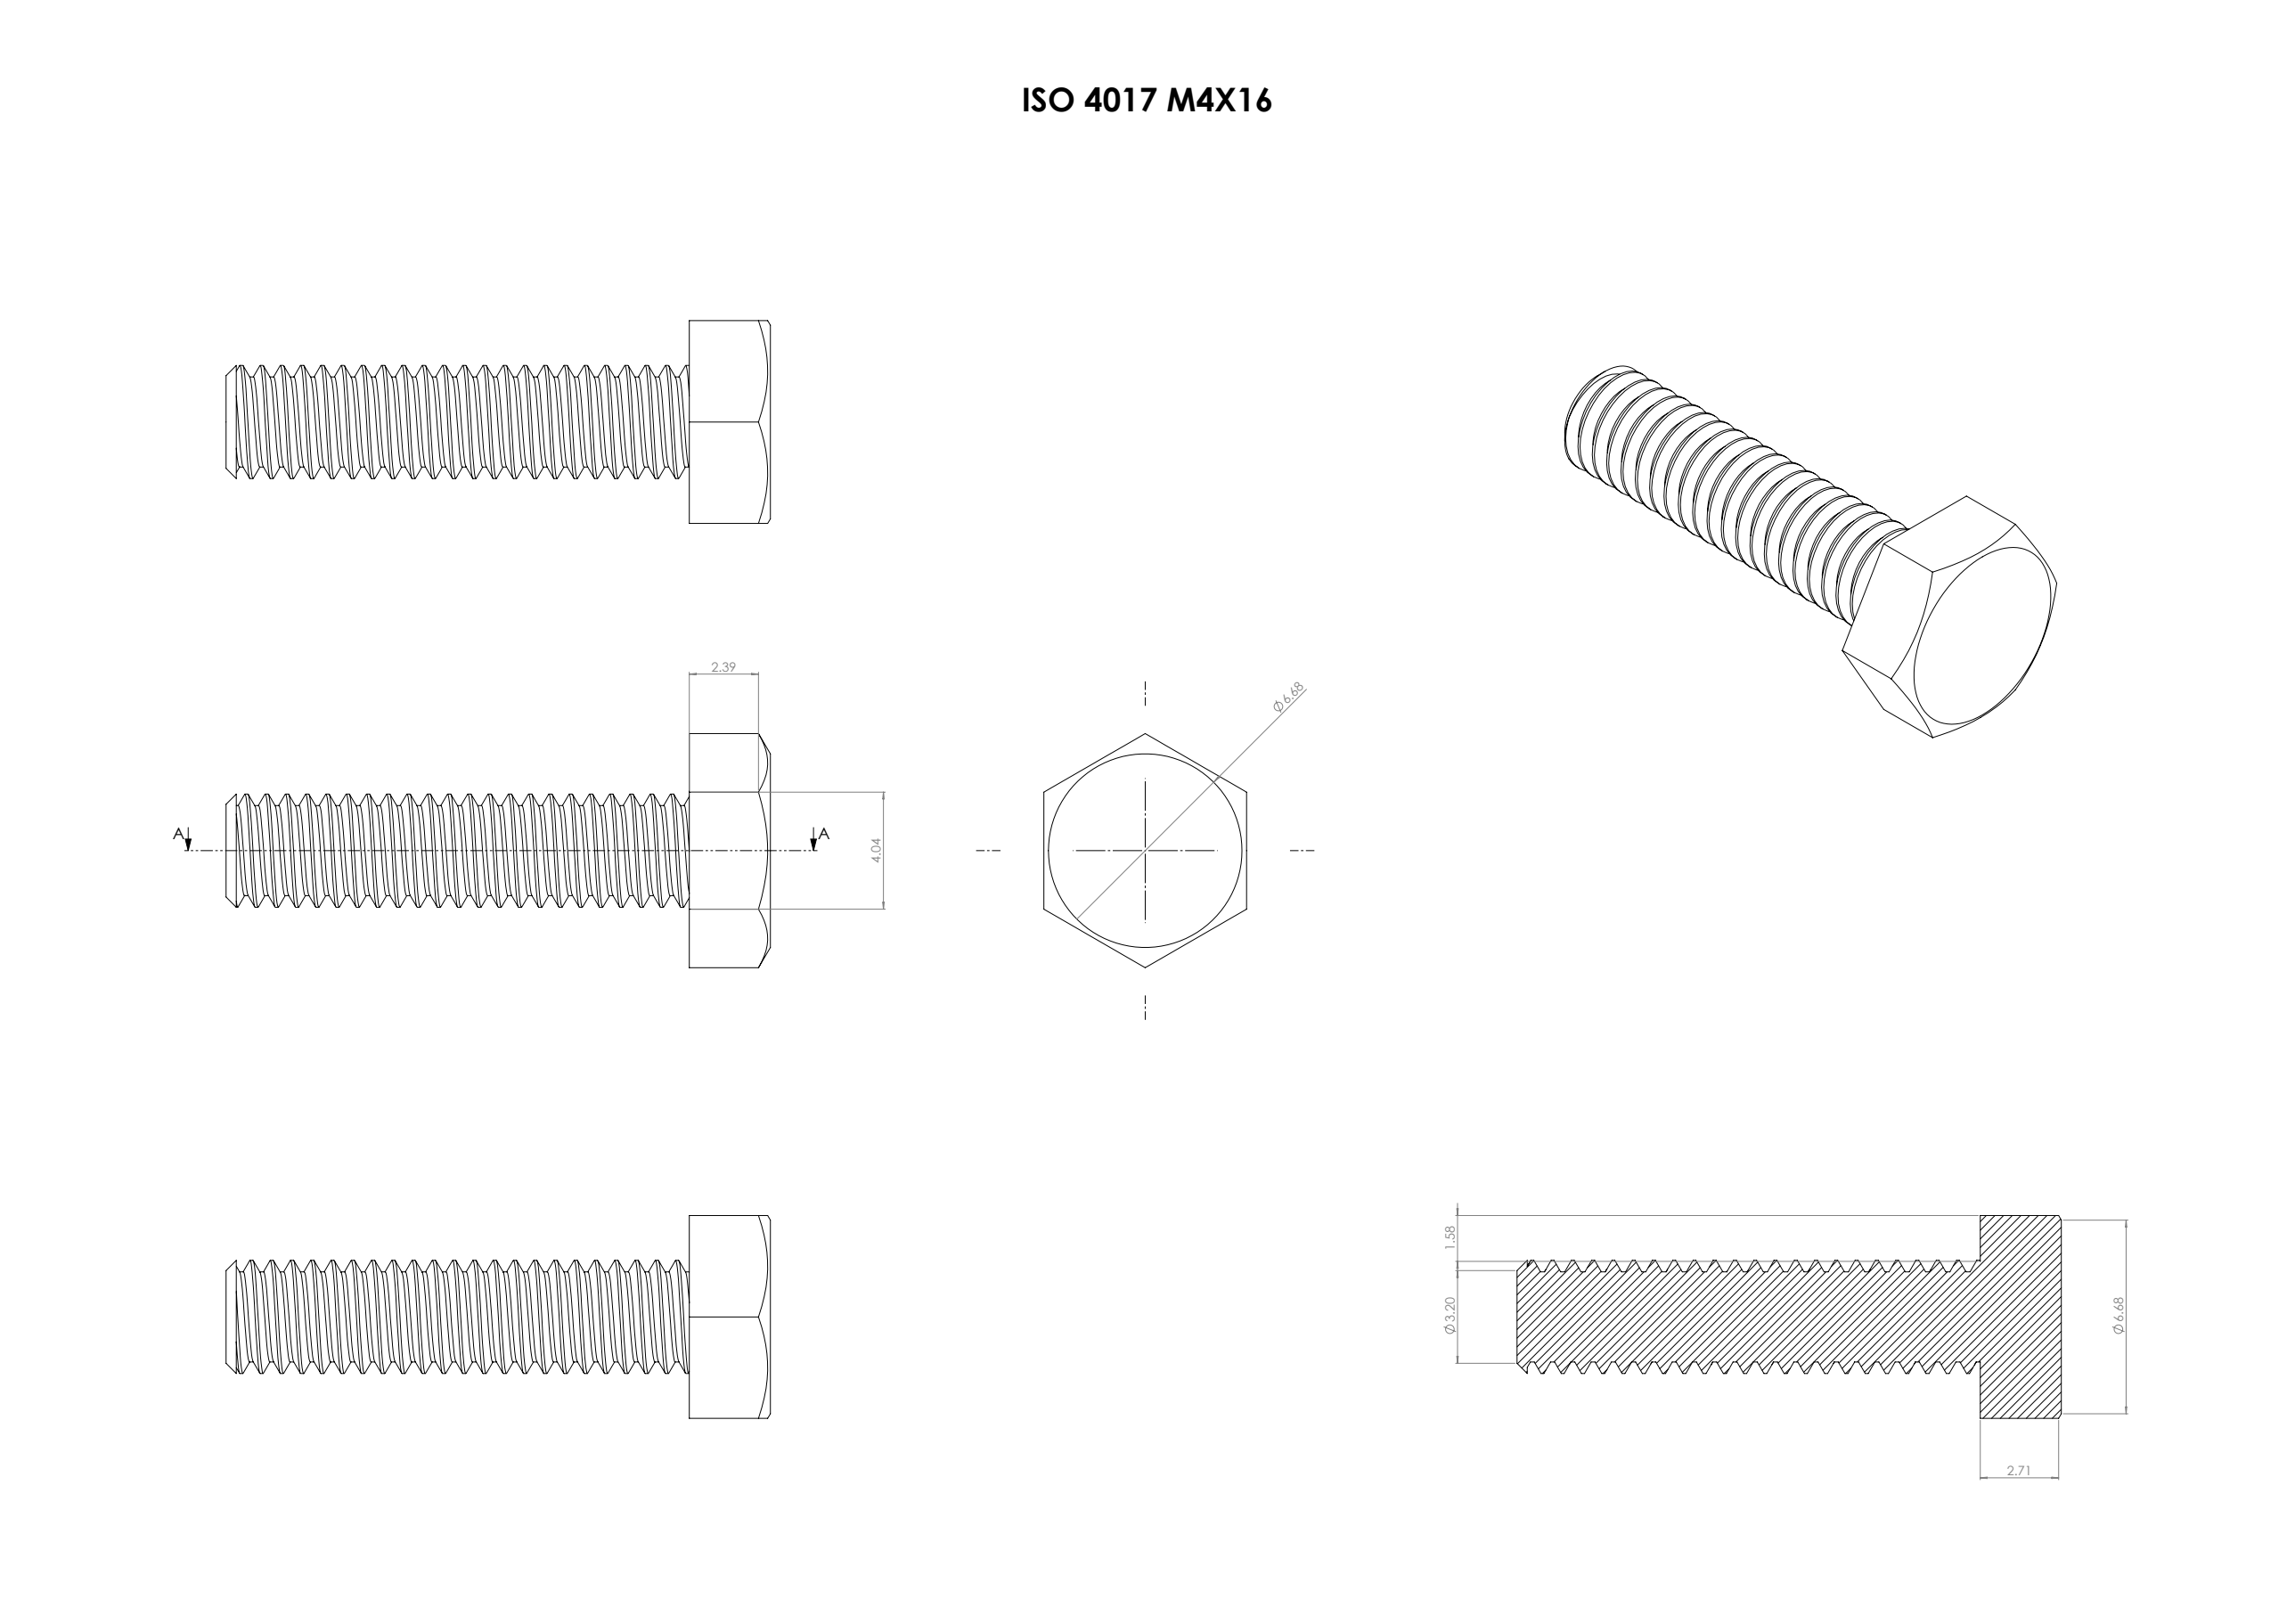
ISO-10303-21;
HEADER;
/* Generated by software containing ST-Developer
 * from STEP Tools, Inc. (www.steptools.com) 
 */

FILE_DESCRIPTION(
/* description */ (''),
/* implementation_level */ '2;1');

FILE_NAME(
/* name */ '09_ISO_4017_M4x16.step',
/* time_stamp */ '2026-10-21T02:01:14-07:00',
/* author */ (''),
/* organization */ (''),
/* preprocessor_version */ 'ST-DEVELOPER v20.2',
/* originating_system */ 'Autodesk Translation Framework v15.15.0.0',
/* authorisation */ '');

FILE_SCHEMA (('AUTOMOTIVE_DESIGN { 1 0 10303 214 3 1 1 }'));
ENDSEC;

DATA;
#10=MECHANICAL_DESIGN_GEOMETRIC_PRESENTATION_REPRESENTATION('',(#622),#37181);
#114=B_SPLINE_SURFACE_WITH_KNOTS('',3,3,((#28629,#28630,#28631,#28632,#28633,
#28634,#28635,#28636,#28637,#28638,#28639,#28640,#28641,#28642,#28643,#28644,
#28645,#28646,#28647,#28648,#28649,#28650,#28651,#28652,#28653,#28654,#28655,
#28656,#28657,#28658,#28659,#28660,#28661,#28662,#28663,#28664,#28665,#28666,
#28667,#28668,#28669,#28670,#28671,#28672,#28673,#28674,#28675,#28676,#28677,
#28678,#28679,#28680,#28681,#28682,#28683,#28684,#28685,#28686,#28687,#28688,
#28689,#28690,#28691,#28692,#28693,#28694,#28695,#28696,#28697,#28698,#28699,
#28700,#28701,#28702,#28703,#28704,#28705,#28706,#28707,#28708,#28709,#28710,
#28711,#28712,#28713,#28714,#28715,#28716,#28717,#28718,#28719,#28720,#28721,
#28722,#28723,#28724,#28725,#28726,#28727,#28728,#28729,#28730,#28731,#28732,
#28733,#28734,#28735,#28736,#28737,#28738,#28739,#28740,#28741,#28742,#28743,
#28744,#28745,#28746,#28747,#28748,#28749,#28750,#28751,#28752,#28753,#28754,
#28755,#28756,#28757,#28758,#28759,#28760,#28761,#28762,#28763,#28764,#28765,
#28766,#28767,#28768,#28769,#28770,#28771,#28772,#28773,#28774),(#28775,
#28776,#28777,#28778,#28779,#28780,#28781,#28782,#28783,#28784,#28785,#28786,
#28787,#28788,#28789,#28790,#28791,#28792,#28793,#28794,#28795,#28796,#28797,
#28798,#28799,#28800,#28801,#28802,#28803,#28804,#28805,#28806,#28807,#28808,
#28809,#28810,#28811,#28812,#28813,#28814,#28815,#28816,#28817,#28818,#28819,
#28820,#28821,#28822,#28823,#28824,#28825,#28826,#28827,#28828,#28829,#28830,
#28831,#28832,#28833,#28834,#28835,#28836,#28837,#28838,#28839,#28840,#28841,
#28842,#28843,#28844,#28845,#28846,#28847,#28848,#28849,#28850,#28851,#28852,
#28853,#28854,#28855,#28856,#28857,#28858,#28859,#28860,#28861,#28862,#28863,
#28864,#28865,#28866,#28867,#28868,#28869,#28870,#28871,#28872,#28873,#28874,
#28875,#28876,#28877,#28878,#28879,#28880,#28881,#28882,#28883,#28884,#28885,
#28886,#28887,#28888,#28889,#28890,#28891,#28892,#28893,#28894,#28895,#28896,
#28897,#28898,#28899,#28900,#28901,#28902,#28903,#28904,#28905,#28906,#28907,
#28908,#28909,#28910,#28911,#28912,#28913,#28914,#28915,#28916,#28917,#28918,
#28919,#28920),(#28921,#28922,#28923,#28924,#28925,#28926,#28927,#28928,
#28929,#28930,#28931,#28932,#28933,#28934,#28935,#28936,#28937,#28938,#28939,
#28940,#28941,#28942,#28943,#28944,#28945,#28946,#28947,#28948,#28949,#28950,
#28951,#28952,#28953,#28954,#28955,#28956,#28957,#28958,#28959,#28960,#28961,
#28962,#28963,#28964,#28965,#28966,#28967,#28968,#28969,#28970,#28971,#28972,
#28973,#28974,#28975,#28976,#28977,#28978,#28979,#28980,#28981,#28982,#28983,
#28984,#28985,#28986,#28987,#28988,#28989,#28990,#28991,#28992,#28993,#28994,
#28995,#28996,#28997,#28998,#28999,#29000,#29001,#29002,#29003,#29004,#29005,
#29006,#29007,#29008,#29009,#29010,#29011,#29012,#29013,#29014,#29015,#29016,
#29017,#29018,#29019,#29020,#29021,#29022,#29023,#29024,#29025,#29026,#29027,
#29028,#29029,#29030,#29031,#29032,#29033,#29034,#29035,#29036,#29037,#29038,
#29039,#29040,#29041,#29042,#29043,#29044,#29045,#29046,#29047,#29048,#29049,
#29050,#29051,#29052,#29053,#29054,#29055,#29056,#29057,#29058,#29059,#29060,
#29061,#29062,#29063,#29064,#29065,#29066),(#29067,#29068,#29069,#29070,
#29071,#29072,#29073,#29074,#29075,#29076,#29077,#29078,#29079,#29080,#29081,
#29082,#29083,#29084,#29085,#29086,#29087,#29088,#29089,#29090,#29091,#29092,
#29093,#29094,#29095,#29096,#29097,#29098,#29099,#29100,#29101,#29102,#29103,
#29104,#29105,#29106,#29107,#29108,#29109,#29110,#29111,#29112,#29113,#29114,
#29115,#29116,#29117,#29118,#29119,#29120,#29121,#29122,#29123,#29124,#29125,
#29126,#29127,#29128,#29129,#29130,#29131,#29132,#29133,#29134,#29135,#29136,
#29137,#29138,#29139,#29140,#29141,#29142,#29143,#29144,#29145,#29146,#29147,
#29148,#29149,#29150,#29151,#29152,#29153,#29154,#29155,#29156,#29157,#29158,
#29159,#29160,#29161,#29162,#29163,#29164,#29165,#29166,#29167,#29168,#29169,
#29170,#29171,#29172,#29173,#29174,#29175,#29176,#29177,#29178,#29179,#29180,
#29181,#29182,#29183,#29184,#29185,#29186,#29187,#29188,#29189,#29190,#29191,
#29192,#29193,#29194,#29195,#29196,#29197,#29198,#29199,#29200,#29201,#29202,
#29203,#29204,#29205,#29206,#29207,#29208,#29209,#29210,#29211,#29212)),
 .UNSPECIFIED.,.F.,.F.,.F.,(4,4),(4,1,1,1,1,1,1,1,1,1,1,1,1,1,1,1,1,1,1,
1,1,1,1,1,1,1,1,1,1,1,1,1,1,1,1,1,1,1,1,1,1,1,1,1,1,1,1,1,1,1,1,1,1,1,1,
1,1,1,1,1,1,1,1,1,1,1,1,1,1,1,1,1,1,1,1,1,1,1,1,1,1,1,1,1,1,1,1,1,1,1,1,
1,1,1,1,1,1,1,1,1,1,1,1,1,1,1,1,1,1,1,1,1,1,1,1,1,1,1,1,1,1,1,1,1,1,1,1,
1,1,1,1,1,1,1,1,1,1,1,1,1,1,1,1,4),(0.,0.0460148164544131),(8.31058692273977,
9.30711355020657,10.3036401776734,11.3001668051402,12.296693432607,13.2932200600738,
14.2897466875406,15.2862733150074,16.2827999424742,17.279326569941,18.2758531974078,
19.2723798248745,20.2689064523413,21.2654330798081,22.2619597072749,23.2584863347417,
24.2550129622085,25.2515395896753,26.2480662171421,27.2445928446089,28.2411194720757,
29.2376460995425,30.2341727270093,31.2306993544761,32.2272259819429,33.2237526094097,
34.2202792368765,35.2168058643433,36.2133324918101,37.2098591192769,38.2063857467437,
39.2029123742105,40.1994390016773,41.1959656291441,42.1924922566109,43.1890188840777,
44.1855455115445,45.1820721390113,46.1785987664781,47.1751253939449,48.1716520214117,
49.1681786488785,50.1647052763453,51.1612319038121,52.1577585312789,53.1542851587457,
54.1508117862125,55.1473384136793,56.1438650411461,57.1403916686129,58.1369182960797,
59.1334449235465,60.1299715510133,61.1264981784801,62.1230248059469,63.1195514334137,
64.1160780608805,65.1126046883473,66.1091313158141,67.1056579432809,68.1021845707477,
69.0987111982145,70.0952378256813,71.0917644531481,72.0882910806149,73.0848177080817,
74.0813443355485,75.0778709630153,76.0743975904821,77.0709242179488,78.0674508454156,
79.0639774728824,80.0605041003492,81.057030727816,82.0535573552828,83.0500839827496,
84.0466106102164,85.0431372376832,86.03966386515,87.0361904926168,88.0327171200836,
89.0292437475504,90.0257703750172,91.022297002484,92.0188236299508,93.0153502574176,
94.0118768848844,95.0084035123512,96.004930139818,97.0014567672848,97.9979833947516,
98.9945100222184,99.9910366496852,100.987563277152,101.984089904619,102.980616532086,
103.977143159552,104.973669787019,105.970196414486,106.966723041953,107.96324966942,
108.959776296886,109.956302924353,110.95282955182,111.949356179287,112.945882806754,
113.94240943422,114.938936061687,115.935462689154,116.931989316621,117.928515944088,
118.925042571554,119.921569199021,120.918095826488,121.914622453955,122.911149081422,
123.907675708888,124.904202336355,125.900728963822,126.897255591289,127.893782218756,
128.890308846222,129.886835473689,130.883362101156,131.879888728623,132.87641535609,
133.872941983556,134.869468611023,135.86599523849,136.862521865957,137.859048493424,
138.85557512089,139.852101748357,140.848628375824,141.845155003291,142.841681630758,
143.838208258224,144.834734885691,145.831261513158,146.827788140625,147.824314768092,
148.820841395558,149.817368023025,150.813894650492),.UNSPECIFIED.);
#115=B_SPLINE_SURFACE_WITH_KNOTS('',3,3,((#29504,#29505,#29506,#29507,#29508,
#29509,#29510,#29511,#29512,#29513,#29514,#29515,#29516,#29517,#29518,#29519,
#29520,#29521,#29522,#29523,#29524,#29525,#29526,#29527,#29528,#29529,#29530,
#29531,#29532,#29533,#29534,#29535,#29536,#29537,#29538,#29539,#29540,#29541,
#29542,#29543,#29544,#29545,#29546,#29547,#29548,#29549,#29550,#29551,#29552,
#29553,#29554,#29555,#29556,#29557,#29558,#29559,#29560,#29561,#29562,#29563,
#29564,#29565,#29566,#29567,#29568,#29569,#29570,#29571,#29572,#29573,#29574,
#29575,#29576,#29577,#29578,#29579,#29580,#29581,#29582,#29583,#29584,#29585,
#29586,#29587,#29588,#29589,#29590,#29591,#29592,#29593,#29594,#29595,#29596,
#29597,#29598,#29599,#29600,#29601,#29602,#29603,#29604,#29605,#29606,#29607,
#29608,#29609,#29610,#29611,#29612,#29613,#29614,#29615,#29616,#29617,#29618,
#29619,#29620,#29621,#29622,#29623,#29624,#29625,#29626,#29627,#29628,#29629,
#29630,#29631,#29632,#29633,#29634,#29635,#29636,#29637,#29638,#29639,#29640,
#29641,#29642,#29643,#29644,#29645,#29646,#29647,#29648,#29649),(#29650,
#29651,#29652,#29653,#29654,#29655,#29656,#29657,#29658,#29659,#29660,#29661,
#29662,#29663,#29664,#29665,#29666,#29667,#29668,#29669,#29670,#29671,#29672,
#29673,#29674,#29675,#29676,#29677,#29678,#29679,#29680,#29681,#29682,#29683,
#29684,#29685,#29686,#29687,#29688,#29689,#29690,#29691,#29692,#29693,#29694,
#29695,#29696,#29697,#29698,#29699,#29700,#29701,#29702,#29703,#29704,#29705,
#29706,#29707,#29708,#29709,#29710,#29711,#29712,#29713,#29714,#29715,#29716,
#29717,#29718,#29719,#29720,#29721,#29722,#29723,#29724,#29725,#29726,#29727,
#29728,#29729,#29730,#29731,#29732,#29733,#29734,#29735,#29736,#29737,#29738,
#29739,#29740,#29741,#29742,#29743,#29744,#29745,#29746,#29747,#29748,#29749,
#29750,#29751,#29752,#29753,#29754,#29755,#29756,#29757,#29758,#29759,#29760,
#29761,#29762,#29763,#29764,#29765,#29766,#29767,#29768,#29769,#29770,#29771,
#29772,#29773,#29774,#29775,#29776,#29777,#29778,#29779,#29780,#29781,#29782,
#29783,#29784,#29785,#29786,#29787,#29788,#29789,#29790,#29791,#29792,#29793,
#29794,#29795),(#29796,#29797,#29798,#29799,#29800,#29801,#29802,#29803,
#29804,#29805,#29806,#29807,#29808,#29809,#29810,#29811,#29812,#29813,#29814,
#29815,#29816,#29817,#29818,#29819,#29820,#29821,#29822,#29823,#29824,#29825,
#29826,#29827,#29828,#29829,#29830,#29831,#29832,#29833,#29834,#29835,#29836,
#29837,#29838,#29839,#29840,#29841,#29842,#29843,#29844,#29845,#29846,#29847,
#29848,#29849,#29850,#29851,#29852,#29853,#29854,#29855,#29856,#29857,#29858,
#29859,#29860,#29861,#29862,#29863,#29864,#29865,#29866,#29867,#29868,#29869,
#29870,#29871,#29872,#29873,#29874,#29875,#29876,#29877,#29878,#29879,#29880,
#29881,#29882,#29883,#29884,#29885,#29886,#29887,#29888,#29889,#29890,#29891,
#29892,#29893,#29894,#29895,#29896,#29897,#29898,#29899,#29900,#29901,#29902,
#29903,#29904,#29905,#29906,#29907,#29908,#29909,#29910,#29911,#29912,#29913,
#29914,#29915,#29916,#29917,#29918,#29919,#29920,#29921,#29922,#29923,#29924,
#29925,#29926,#29927,#29928,#29929,#29930,#29931,#29932,#29933,#29934,#29935,
#29936,#29937,#29938,#29939,#29940,#29941),(#29942,#29943,#29944,#29945,
#29946,#29947,#29948,#29949,#29950,#29951,#29952,#29953,#29954,#29955,#29956,
#29957,#29958,#29959,#29960,#29961,#29962,#29963,#29964,#29965,#29966,#29967,
#29968,#29969,#29970,#29971,#29972,#29973,#29974,#29975,#29976,#29977,#29978,
#29979,#29980,#29981,#29982,#29983,#29984,#29985,#29986,#29987,#29988,#29989,
#29990,#29991,#29992,#29993,#29994,#29995,#29996,#29997,#29998,#29999,#30000,
#30001,#30002,#30003,#30004,#30005,#30006,#30007,#30008,#30009,#30010,#30011,
#30012,#30013,#30014,#30015,#30016,#30017,#30018,#30019,#30020,#30021,#30022,
#30023,#30024,#30025,#30026,#30027,#30028,#30029,#30030,#30031,#30032,#30033,
#30034,#30035,#30036,#30037,#30038,#30039,#30040,#30041,#30042,#30043,#30044,
#30045,#30046,#30047,#30048,#30049,#30050,#30051,#30052,#30053,#30054,#30055,
#30056,#30057,#30058,#30059,#30060,#30061,#30062,#30063,#30064,#30065,#30066,
#30067,#30068,#30069,#30070,#30071,#30072,#30073,#30074,#30075,#30076,#30077,
#30078,#30079,#30080,#30081,#30082,#30083,#30084,#30085,#30086,#30087)),
 .UNSPECIFIED.,.F.,.F.,.F.,(4,4),(4,1,1,1,1,1,1,1,1,1,1,1,1,1,1,1,1,1,1,
1,1,1,1,1,1,1,1,1,1,1,1,1,1,1,1,1,1,1,1,1,1,1,1,1,1,1,1,1,1,1,1,1,1,1,1,
1,1,1,1,1,1,1,1,1,1,1,1,1,1,1,1,1,1,1,1,1,1,1,1,1,1,1,1,1,1,1,1,1,1,1,1,
1,1,1,1,1,1,1,1,1,1,1,1,1,1,1,1,1,1,1,1,1,1,1,1,1,1,1,1,1,1,1,1,1,1,1,1,
1,1,1,1,1,1,1,1,1,1,1,1,1,1,1,1,4),(0.,0.0460148164544131),(11.6154215191106,
12.6119481465774,13.6084747740442,14.605001401511,15.6015280289778,16.5980546564446,
17.5945812839114,18.5911079113782,19.587634538845,20.5841611663118,21.5806877937786,
22.5772144212454,23.5737410487122,24.570267676179,25.5667943036458,26.5633209311126,
27.5598475585794,28.5563741860462,29.552900813513,30.5494274409798,31.5459540684466,
32.5424806959134,33.5390073233802,34.535533950847,35.5320605783138,36.5285872057806,
37.5251138332474,38.5216404607142,39.518167088181,40.5146937156478,41.5112203431146,
42.5077469705814,43.5042735980482,44.500800225515,45.4973268529818,46.4938534804486,
47.4903801079154,48.4869067353822,49.483433362849,50.4799599903158,51.4764866177826,
52.4730132452493,53.4695398727161,54.4660665001829,55.4625931276497,56.4591197551165,
57.4556463825833,58.4521730100501,59.4486996375169,60.4452262649837,61.4417528924505,
62.4382795199173,63.4348061473841,64.4313327748509,65.4278594023177,66.4243860297845,
67.4209126572513,68.4174392847181,69.4139659121849,70.4104925396517,71.4070191671185,
72.4035457945853,73.4000724220521,74.3965990495189,75.3931256769857,76.3896523044525,
77.3861789319193,78.3827055593861,79.3792321868529,80.3757588143197,81.3722854417865,
82.3688120692533,83.3653386967201,84.3618653241869,85.3583919516537,86.3549185791205,
87.3514452065873,88.3479718340541,89.3444984615209,90.3410250889877,91.3375517164545,
92.3340783439213,93.3306049713881,94.3271315988549,95.3236582263217,96.3201848537885,
97.3167114812553,98.313238108722,99.3097647361889,100.306291363656,101.302817991122,
102.299344618589,103.295871246056,104.292397873523,105.28892450099,106.285451128456,
107.281977755923,108.27850438339,109.275031010857,110.271557638324,111.26808426579,
112.264610893257,113.261137520724,114.257664148191,115.254190775658,116.250717403124,
117.247244030591,118.243770658058,119.240297285525,120.236823912992,121.233350540458,
122.229877167925,123.226403795392,124.222930422859,125.219457050326,126.215983677792,
127.212510305259,128.209036932726,129.205563560193,130.20209018766,131.198616815126,
132.195143442593,133.19167007006,134.188196697527,135.184723324994,136.18124995246,
137.177776579927,138.174303207394,139.170829834861,140.167356462328,141.163883089794,
142.160409717261,143.156936344728,144.153462972195,145.149989599662,146.146516227128,
147.143042854595,148.139569482062,149.136096109529,150.132622736996,151.129149364462,
152.125675991929,153.122202619396,154.118729246863),.UNSPECIFIED.);
#281=B_SPLINE_CURVE_WITH_KNOTS('',3,(#26983,#26984,#26985,#26986,#26987,
#26988,#26989,#26990,#26991,#26992),.UNSPECIFIED.,.F.,.F.,(4,3,3,4),(-4.09254174883829,
-3.98610650986719,-2.98957988240039,-2.06514013327809),.UNSPECIFIED.);
#282=B_SPLINE_CURVE_WITH_KNOTS('',3,(#26995,#26996,#26997,#26998,#26999,
#27000,#27001),.UNSPECIFIED.,.F.,.F.,(4,3,4),(0.,0.996526627466801,1.11419103802947),
 .UNSPECIFIED.);
#283=B_SPLINE_CURVE_WITH_KNOTS('',3,(#27006,#27007,#27008,#27009,#27010,
#27011,#27012,#27013,#27014,#27015,#27016,#27017,#27018,#27019,#27020,#27021,
#27022,#27023,#27024,#27025,#27026,#27027),.UNSPECIFIED.,.F.,.F.,(4,3,3,
3,3,3,3,4),(-10.3757270560179,-9.96526627466798,-8.96873964720119,-7.97221301973439,
-6.97568639226759,-5.97915976480079,-4.98263313733399,-4.09254174883829),
 .UNSPECIFIED.);
#284=B_SPLINE_CURVE_WITH_KNOTS('',3,(#27028,#27029,#27030,#27031,#27032,
#27033,#27034,#27035,#27036,#27037,#27038,#27039,#27040,#27041,#27042,#27043,
#27044,#27045,#27046,#27047,#27048,#27049),.UNSPECIFIED.,.F.,.F.,(4,3,3,
3,3,3,3,4),(1.11419103802947,1.9930532549336,2.9895798824004,3.98610650986719,
4.98263313733399,5.97915976480079,6.97568639226759,7.39737634520906),
 .UNSPECIFIED.);
#285=B_SPLINE_CURVE_WITH_KNOTS('',3,(#27054,#27055,#27056,#27057,#27058,
#27059,#27060,#27061,#27062,#27063,#27064,#27065,#27066,#27067,#27068,#27069,
#27070,#27071,#27072,#27073,#27074,#27075),.UNSPECIFIED.,.F.,.F.,(4,3,3,
3,3,3,3,4),(-16.6589123631975,-15.9444260394688,-14.947899412002,-13.9513727845352,
-12.9548461570684,-11.9583195296016,-10.9617929021348,-10.3757270560179),
 .UNSPECIFIED.);
#286=B_SPLINE_CURVE_WITH_KNOTS('',3,(#27076,#27077,#27078,#27079,#27080,
#27081,#27082,#27083,#27084,#27085,#27086,#27087,#27088,#27089,#27090,#27091,
#27092,#27093,#27094,#27095,#27096,#27097),.UNSPECIFIED.,.F.,.F.,(4,3,3,
3,3,3,3,4),(7.39737634520906,7.97221301973439,8.96873964720119,9.96526627466799,
10.9617929021348,11.9583195296016,12.9548461570684,13.6805616523886),
 .UNSPECIFIED.);
#287=B_SPLINE_CURVE_WITH_KNOTS('',3,(#27102,#27103,#27104,#27105,#27106,
#27107,#27108,#27109,#27110,#27111,#27112,#27113,#27114,#27115,#27116,#27117,
#27118,#27119,#27120,#27121,#27122,#27123,#27124,#27125,#27126),
 .UNSPECIFIED.,.F.,.F.,(4,3,3,3,3,3,3,3,4),(-22.942097670377,-22.9201124317364,
-21.9235858042696,-20.9270591768028,-19.930532549336,-18.9340059218692,
-17.9374792944024,-16.9409526669356,-16.6589123631975),.UNSPECIFIED.);
#288=B_SPLINE_CURVE_WITH_KNOTS('',3,(#27127,#27128,#27129,#27130,#27131,
#27132,#27133,#27134,#27135,#27136,#27137,#27138,#27139,#27140,#27141,#27142,
#27143,#27144,#27145,#27146,#27147,#27148,#27149,#27150,#27151),
 .UNSPECIFIED.,.F.,.F.,(4,3,3,3,3,3,3,3,4),(13.6805616523886,13.9513727845352,
14.947899412002,15.9444260394688,16.9409526669356,17.9374792944024,18.9340059218692,
19.930532549336,19.9637469595682),.UNSPECIFIED.);
#289=B_SPLINE_CURVE_WITH_KNOTS('',3,(#27156,#27157,#27158,#27159,#27160,
#27161,#27162,#27163,#27164,#27165,#27166,#27167,#27168,#27169,#27170,#27171,
#27172,#27173,#27174,#27175,#27176,#27177),.UNSPECIFIED.,.F.,.F.,(4,3,3,
3,3,3,3,4),(-29.2252829775566,-28.8992721965371,-27.9027455690703,-26.9062189416035,
-25.9096923141368,-24.91316568667,-23.9166390592032,-22.942097670377),
 .UNSPECIFIED.);
#290=B_SPLINE_CURVE_WITH_KNOTS('',3,(#27178,#27179,#27180,#27181,#27182,
#27183,#27184,#27185,#27186,#27187,#27188,#27189,#27190,#27191,#27192,#27193,
#27194,#27195,#27196,#27197,#27198,#27199),.UNSPECIFIED.,.F.,.F.,(4,3,3,
3,3,3,3,4),(19.9637469595682,20.9270591768028,21.9235858042696,22.9201124317364,
23.9166390592031,24.91316568667,25.9096923141368,26.2469322667478),
 .UNSPECIFIED.);
#291=B_SPLINE_CURVE_WITH_KNOTS('',3,(#27204,#27205,#27206,#27207,#27208,
#27209,#27210,#27211,#27212,#27213,#27214,#27215,#27216,#27217,#27218,#27219,
#27220,#27221,#27222,#27223,#27224,#27225),.UNSPECIFIED.,.F.,.F.,(4,3,3,
3,3,3,3,4),(-35.5084682847362,-34.8784319613379,-33.8819053338711,-32.8853787064043,
-31.8888520789375,-30.8923254514707,-29.8957988240039,-29.2252829775566),
 .UNSPECIFIED.);
#292=B_SPLINE_CURVE_WITH_KNOTS('',3,(#27226,#27227,#27228,#27229,#27230,
#27231,#27232,#27233,#27234,#27235,#27236,#27237,#27238,#27239,#27240,#27241,
#27242,#27243,#27244,#27245,#27246,#27247),.UNSPECIFIED.,.F.,.F.,(4,3,3,
3,3,3,3,4),(26.2469322667478,26.9062189416035,27.9027455690703,28.8992721965371,
29.895798824004,30.8923254514707,31.8888520789375,32.5301175739274),
 .UNSPECIFIED.);
#293=B_SPLINE_CURVE_WITH_KNOTS('',3,(#27252,#27253,#27254,#27255,#27256,
#27257,#27258,#27259,#27260,#27261,#27262,#27263,#27264,#27265,#27266,#27267,
#27268,#27269,#27270,#27271,#27272,#27273),.UNSPECIFIED.,.F.,.F.,(4,3,3,
3,3,3,3,4),(-41.7916535919158,-40.8575917261387,-39.8610650986719,-38.8645384712051,
-37.8680118437383,-36.8714852162715,-35.8749585888047,-35.5084682847362),
 .UNSPECIFIED.);
#294=B_SPLINE_CURVE_WITH_KNOTS('',3,(#27274,#27275,#27276,#27277,#27278,
#27279,#27280,#27281,#27282,#27283,#27284,#27285,#27286,#27287,#27288,#27289,
#27290,#27291,#27292,#27293,#27294,#27295),.UNSPECIFIED.,.F.,.F.,(4,3,3,
3,3,3,3,4),(32.5301175739274,32.8853787064043,33.8819053338711,34.8784319613379,
35.8749585888047,36.8714852162715,37.8680118437383,38.813302881107),
 .UNSPECIFIED.);
#295=B_SPLINE_CURVE_WITH_KNOTS('',3,(#27300,#27301,#27302,#27303,#27304,
#27305,#27306,#27307,#27308,#27309,#27310,#27311,#27312,#27313,#27314,#27315,
#27316,#27317,#27318,#27319,#27320,#27321,#27322,#27323,#27324),
 .UNSPECIFIED.,.F.,.F.,(4,3,3,3,3,3,3,3,4),(-48.0748388990954,-47.8332781184063,
-46.8367514909395,-45.8402248634727,-44.8436982360059,-43.8471716085391,
-42.8506449810723,-41.8541183536055,-41.7916535919158),.UNSPECIFIED.);
#296=B_SPLINE_CURVE_WITH_KNOTS('',3,(#27325,#27326,#27327,#27328,#27329,
#27330,#27331,#27332,#27333,#27334,#27335,#27336,#27337,#27338,#27339,#27340,
#27341,#27342,#27343,#27344,#27345,#27346,#27347,#27348,#27349),
 .UNSPECIFIED.,.F.,.F.,(4,3,3,3,3,3,3,3,4),(38.813302881107,38.8645384712051,
39.8610650986719,40.8575917261387,41.8541183536055,42.8506449810723,43.8471716085391,
44.8436982360059,45.0964881882866),.UNSPECIFIED.);
#297=B_SPLINE_CURVE_WITH_KNOTS('',3,(#27354,#27355,#27356,#27357,#27358,
#27359,#27360,#27361,#27362,#27363,#27364,#27365,#27366,#27367,#27368,#27369,
#27370,#27371,#27372,#27373,#27374,#27375),.UNSPECIFIED.,.F.,.F.,(4,3,3,
3,3,3,3,4),(-54.358024206275,-53.8124378832071,-52.8159112557403,-51.8193846282735,
-50.8228580008067,-49.8263313733399,-48.8298047458731,-48.0748388990954),
 .UNSPECIFIED.);
#298=B_SPLINE_CURVE_WITH_KNOTS('',3,(#27376,#27377,#27378,#27379,#27380,
#27381,#27382,#27383,#27384,#27385,#27386,#27387,#27388,#27389,#27390,#27391,
#27392,#27393,#27394,#27395,#27396,#27397),.UNSPECIFIED.,.F.,.F.,(4,3,3,
3,3,3,3,4),(45.0964881882866,45.8402248634727,46.8367514909395,47.8332781184063,
48.8298047458731,49.8263313733399,50.8228580008067,51.3796734954662),
 .UNSPECIFIED.);
#299=B_SPLINE_CURVE_WITH_KNOTS('',3,(#27402,#27403,#27404,#27405,#27406,
#27407,#27408,#27409,#27410,#27411,#27412,#27413,#27414,#27415,#27416,#27417,
#27418,#27419,#27420,#27421,#27422,#27423),.UNSPECIFIED.,.F.,.F.,(4,3,3,
3,3,3,3,4),(-60.6412095134546,-59.7915976480079,-58.7950710205411,-57.7985443930743,
-56.8020177656075,-55.8054911381407,-54.8089645106739,-54.358024206275),
 .UNSPECIFIED.);
#300=B_SPLINE_CURVE_WITH_KNOTS('',3,(#27424,#27425,#27426,#27427,#27428,
#27429,#27430,#27431,#27432,#27433,#27434,#27435,#27436,#27437,#27438,#27439,
#27440,#27441,#27442,#27443,#27444,#27445),.UNSPECIFIED.,.F.,.F.,(4,3,3,
3,3,3,3,4),(51.3796734954662,51.8193846282735,52.8159112557403,53.8124378832071,
54.8089645106739,55.8054911381407,56.8020177656075,57.6628588026458),
 .UNSPECIFIED.);
#301=B_SPLINE_CURVE_WITH_KNOTS('',3,(#27450,#27451,#27452,#27453,#27454,
#27455,#27456,#27457,#27458,#27459,#27460,#27461,#27462,#27463,#27464,#27465,
#27466,#27467,#27468,#27469,#27470,#27471,#27472,#27473,#27474),
 .UNSPECIFIED.,.F.,.F.,(4,3,3,3,3,3,3,3,4),(-66.9243948206342,-66.7672840402755,
-65.7707574128087,-64.7742307853419,-63.7777041578751,-62.7811775304083,
-61.7846509029415,-60.7881242754747,-60.6412095134546),.UNSPECIFIED.);
#302=B_SPLINE_CURVE_WITH_KNOTS('',3,(#27475,#27476,#27477,#27478,#27479,
#27480,#27481,#27482,#27483,#27484,#27485,#27486,#27487,#27488,#27489,#27490,
#27491,#27492,#27493,#27494,#27495,#27496,#27497,#27498,#27499),
 .UNSPECIFIED.,.F.,.F.,(4,3,3,3,3,3,3,3,4),(57.6628588026458,57.7985443930743,
58.7950710205411,59.7915976480079,60.7881242754747,61.7846509029415,62.7811775304083,
63.7777041578751,63.9460441098254),.UNSPECIFIED.);
#303=B_SPLINE_CURVE_WITH_KNOTS('',3,(#27504,#27505,#27506,#27507,#27508,
#27509,#27510,#27511,#27512,#27513,#27514,#27515,#27516,#27517,#27518,#27519,
#27520,#27521,#27522,#27523,#27524,#27525),.UNSPECIFIED.,.F.,.F.,(4,3,3,
3,3,3,3,4),(-73.2075801278138,-72.7464438050762,-71.7499171776095,-70.7533905501426,
-69.7568639226759,-68.760337295209,-67.7638106677423,-66.9243948206342),
 .UNSPECIFIED.);
#304=B_SPLINE_CURVE_WITH_KNOTS('',3,(#27526,#27527,#27528,#27529,#27530,
#27531,#27532,#27533,#27534,#27535,#27536,#27537,#27538,#27539,#27540,#27541,
#27542,#27543,#27544,#27545,#27546,#27547),.UNSPECIFIED.,.F.,.F.,(4,3,3,
3,3,3,3,4),(63.9460441098254,64.7742307853419,65.7707574128087,66.7672840402755,
67.7638106677423,68.7603372952091,69.7568639226759,70.229229417005),
 .UNSPECIFIED.);
#305=B_SPLINE_CURVE_WITH_KNOTS('',3,(#27552,#27553,#27554,#27555,#27556,
#27557,#27558,#27559,#27560,#27561,#27562,#27563,#27564,#27565,#27566,#27567,
#27568,#27569,#27570,#27571,#27572,#27573),.UNSPECIFIED.,.F.,.F.,(4,3,3,
3,3,3,3,4),(-79.4907654349934,-78.725603569877,-77.7290769424102,-76.7325503149434,
-75.7360236874766,-74.7394970600099,-73.742970432543,-73.2075801278138),
 .UNSPECIFIED.);
#306=B_SPLINE_CURVE_WITH_KNOTS('',3,(#27574,#27575,#27576,#27577,#27578,
#27579,#27580,#27581,#27582,#27583,#27584,#27585,#27586,#27587,#27588,#27589,
#27590,#27591,#27592,#27593,#27594,#27595),.UNSPECIFIED.,.F.,.F.,(4,3,3,
3,3,3,3,4),(70.229229417005,70.7533905501427,71.7499171776095,72.7464438050763,
73.7429704325431,74.7394970600099,75.7360236874767,76.5124147241846),
 .UNSPECIFIED.);
#307=B_SPLINE_CURVE_WITH_KNOTS('',3,(#27600,#27601,#27602,#27603,#27604,
#27605,#27606,#27607,#27608,#27609,#27610,#27611,#27612,#27613,#27614,#27615,
#27616,#27617,#27618,#27619,#27620,#27621,#27622,#27623,#27624),
 .UNSPECIFIED.,.F.,.F.,(4,3,3,3,3,3,3,3,4),(-85.773950742173,-85.7012899621446,
-84.7047633346778,-83.708236707211,-82.7117100797442,-81.7151834522774,
-80.7186568248106,-79.7221301973438,-79.4907654349934),.UNSPECIFIED.);
#308=B_SPLINE_CURVE_WITH_KNOTS('',3,(#27625,#27626,#27627,#27628,#27629,
#27630,#27631,#27632,#27633,#27634,#27635,#27636,#27637,#27638,#27639,#27640,
#27641,#27642,#27643,#27644,#27645,#27646,#27647,#27648,#27649),
 .UNSPECIFIED.,.F.,.F.,(4,3,3,3,3,3,3,3,4),(76.5124147241846,76.7325503149435,
77.7290769424103,78.7256035698771,79.7221301973439,80.7186568248107,81.7151834522775,
82.7117100797443,82.7956000313641),.UNSPECIFIED.);
#309=B_SPLINE_CURVE_WITH_KNOTS('',3,(#27654,#27655,#27656,#27657,#27658,
#27659,#27660,#27661,#27662,#27663,#27664,#27665,#27666,#27667,#27668,#27669,
#27670,#27671,#27672,#27673,#27674,#27675),.UNSPECIFIED.,.F.,.F.,(4,3,3,
3,3,3,3,4),(-92.0571360493526,-91.6804497269454,-90.6839230994786,-89.6873964720118,
-88.690869844545,-87.6943432170782,-86.6978165896114,-85.773950742173),
 .UNSPECIFIED.);
#310=B_SPLINE_CURVE_WITH_KNOTS('',3,(#27676,#27677,#27678,#27679,#27680,
#27681,#27682,#27683,#27684,#27685,#27686,#27687,#27688,#27689,#27690,#27691,
#27692,#27693,#27694,#27695,#27696,#27697),.UNSPECIFIED.,.F.,.F.,(4,3,3,
3,3,3,3,4),(82.7956000313641,83.7082367072111,84.7047633346779,85.7012899621447,
86.6978165896115,87.6943432170783,88.690869844545,89.0787853385437),
 .UNSPECIFIED.);
#311=B_SPLINE_CURVE_WITH_KNOTS('',3,(#27702,#27703,#27704,#27705,#27706,
#27707,#27708,#27709,#27710,#27711,#27712,#27713,#27714,#27715,#27716,#27717,
#27718,#27719,#27720,#27721,#27722,#27723),.UNSPECIFIED.,.F.,.F.,(4,3,3,
3,3,3,3,4),(-98.3403213565322,-97.6596094917462,-96.6630828642794,-95.6665562368126,
-94.6700296093458,-93.673502981879,-92.6769763544122,-92.0571360493526),
 .UNSPECIFIED.);
#312=B_SPLINE_CURVE_WITH_KNOTS('',3,(#27724,#27725,#27726,#27727,#27728,
#27729,#27730,#27731,#27732,#27733,#27734,#27735,#27736,#27737,#27738,#27739,
#27740,#27741,#27742,#27743,#27744,#27745),.UNSPECIFIED.,.F.,.F.,(4,3,3,
3,3,3,3,4),(89.0787853385437,89.6873964720119,90.6839230994786,91.6804497269455,
92.6769763544122,93.673502981879,94.6700296093458,95.3619706457233),
 .UNSPECIFIED.);
#313=B_SPLINE_CURVE_WITH_KNOTS('',3,(#27750,#27751,#27752,#27753,#27754,
#27755,#27756,#27757,#27758,#27759,#27760,#27761,#27762,#27763,#27764,#27765,
#27766,#27767,#27768,#27769,#27770,#27771),.UNSPECIFIED.,.F.,.F.,(4,3,3,
3,3,3,3,4),(-104.623506663712,-103.638769256547,-102.64224262908,-101.645716001613,
-100.649189374147,-99.6526627466798,-98.656136119213,-98.3403213565322),
 .UNSPECIFIED.);
#314=B_SPLINE_CURVE_WITH_KNOTS('',3,(#27772,#27773,#27774,#27775,#27776,
#27777,#27778,#27779,#27780,#27781,#27782,#27783,#27784,#27785,#27786,#27787,
#27788,#27789,#27790,#27791,#27792,#27793),.UNSPECIFIED.,.F.,.F.,(4,3,3,
3,3,3,3,4),(95.3619706457233,95.6665562368126,96.6630828642794,97.6596094917462,
98.656136119213,99.6526627466798,100.649189374147,101.645155952903),
 .UNSPECIFIED.);
#315=B_SPLINE_CURVE_WITH_KNOTS('',3,(#27798,#27799,#27800,#27801,#27802,
#27803,#27804,#27805,#27806,#27807,#27808,#27809,#27810,#27811,#27812,#27813,
#27814,#27815,#27816,#27817,#27818,#27819,#27820,#27821,#27822),
 .UNSPECIFIED.,.F.,.F.,(4,3,3,3,3,3,3,3,4),(-110.906691970891,-110.614455648815,
-109.617929021348,-108.621402393881,-107.624875766414,-106.628349138947,
-105.631822511481,-104.635295884014,-104.623506663712),.UNSPECIFIED.);
#316=B_SPLINE_CURVE_WITH_KNOTS('',3,(#27823,#27824,#27825,#27826,#27827,
#27828,#27829,#27830,#27831,#27832,#27833,#27834,#27835,#27836,#27837,#27838,
#27839,#27840,#27841,#27842,#27843,#27844),.UNSPECIFIED.,.F.,.F.,(4,3,3,
3,3,3,3,4),(101.645155952903,102.64224262908,103.638769256547,104.635295884014,
105.631822511481,106.628349138947,107.624875766414,107.928341260083),
 .UNSPECIFIED.);
#317=B_SPLINE_CURVE_WITH_KNOTS('',3,(#27849,#27850,#27851,#27852,#27853,
#27854,#27855,#27856,#27857,#27858,#27859,#27860,#27861,#27862,#27863,#27864,
#27865,#27866,#27867,#27868,#27869,#27870),.UNSPECIFIED.,.F.,.F.,(4,3,3,
3,3,3,3,4),(-117.189877278071,-116.593615413615,-115.597088786149,-114.600562158682,
-113.604035531215,-112.607508903748,-111.610982276281,-110.906691970891),
 .UNSPECIFIED.);
#318=B_SPLINE_CURVE_WITH_KNOTS('',3,(#27871,#27872,#27873,#27874,#27875,
#27876,#27877,#27878,#27879,#27880,#27881,#27882,#27883,#27884,#27885,#27886,
#27887,#27888,#27889,#27890,#27891,#27892),.UNSPECIFIED.,.F.,.F.,(4,3,3,
3,3,3,3,4),(107.928341260083,108.621402393881,109.617929021348,110.614455648815,
111.610982276281,112.607508903748,113.604035531215,114.211526567262),
 .UNSPECIFIED.);
#319=B_SPLINE_CURVE_WITH_KNOTS('',3,(#27897,#27898,#27899,#27900,#27901,
#27902,#27903,#27904,#27905,#27906,#27907,#27908,#27909,#27910,#27911,#27912,
#27913,#27914,#27915,#27916,#27917,#27918),.UNSPECIFIED.,.F.,.F.,(4,3,3,
3,3,3,3,4),(-123.473062585251,-122.572775178416,-121.576248550949,-120.579721923483,
-119.583195296016,-118.586668668549,-117.590142041082,-117.189877278071),
 .UNSPECIFIED.);
#320=B_SPLINE_CURVE_WITH_KNOTS('',3,(#27919,#27920,#27921,#27922,#27923,
#27924,#27925,#27926,#27927,#27928,#27929,#27930,#27931,#27932,#27933,#27934,
#27935,#27936,#27937,#27938,#27939,#27940),.UNSPECIFIED.,.F.,.F.,(4,3,3,
3,3,3,3,4),(114.211526567262,114.600562158682,115.597088786149,116.593615413615,
117.590142041082,118.586668668549,119.583195296016,120.494711874442),
 .UNSPECIFIED.);
#321=B_SPLINE_CURVE_WITH_KNOTS('',3,(#27945,#27946,#27947,#27948,#27949,
#27950,#27951,#27952,#27953,#27954,#27955,#27956,#27957,#27958,#27959,#27960,
#27961,#27962,#27963,#27964,#27965,#27966,#27967,#27968,#27969),
 .UNSPECIFIED.,.F.,.F.,(4,3,3,3,3,3,3,3,4),(-129.75624789243,-129.548461570684,
-128.551934943217,-127.55540831575,-126.558881688283,-125.562355060817,
-124.56582843335,-123.569301805883,-123.473062585251),.UNSPECIFIED.);
#322=B_SPLINE_CURVE_WITH_KNOTS('',3,(#27970,#27971,#27972,#27973,#27974,
#27975,#27976,#27977,#27978,#27979,#27980,#27981,#27982,#27983,#27984,#27985,
#27986,#27987,#27988,#27989,#27990,#27991,#27992,#27993,#27994),
 .UNSPECIFIED.,.F.,.F.,(4,3,3,3,3,3,3,3,4),(120.494711874442,120.579721923483,
121.576248550949,122.572775178416,123.569301805883,124.56582843335,125.562355060817,
126.558881688283,126.777897181621),.UNSPECIFIED.);
#323=B_SPLINE_CURVE_WITH_KNOTS('',3,(#27999,#28000,#28001,#28002,#28003,
#28004,#28005,#28006,#28007,#28008,#28009,#28010,#28011,#28012,#28013,#28014,
#28015,#28016,#28017,#28018,#28019,#28020),.UNSPECIFIED.,.F.,.F.,(4,3,3,
3,3,3,3,4),(-136.03943319961,-135.527621335485,-134.531094708018,-133.534568080551,
-132.538041453084,-131.541514825617,-130.544988198151,-129.75624789243),
 .UNSPECIFIED.);
#324=B_SPLINE_CURVE_WITH_KNOTS('',3,(#28021,#28022,#28023,#28024,#28025,
#28026,#28027,#28028,#28029,#28030,#28031,#28032,#28033,#28034,#28035,#28036,
#28037,#28038,#28039,#28040,#28041,#28042),.UNSPECIFIED.,.F.,.F.,(4,3,3,
3,3,3,3,4),(126.777897181621,127.55540831575,128.551934943217,129.548461570684,
130.544988198151,131.541514825617,132.538041453084,133.061082488801),
 .UNSPECIFIED.);
#325=B_SPLINE_CURVE_WITH_KNOTS('',3,(#28047,#28048,#28049,#28050,#28051,
#28052,#28053,#28054,#28055,#28056,#28057,#28058,#28059,#28060,#28061,#28062,
#28063,#28064,#28065,#28066,#28067,#28068),.UNSPECIFIED.,.F.,.F.,(4,3,3,
3,3,3,3,4),(-142.322618506789,-141.506781100285,-140.510254472819,-139.513727845352,
-138.517201217885,-137.520674590418,-136.524147962951,-136.03943319961),
 .UNSPECIFIED.);
#326=B_SPLINE_CURVE_WITH_KNOTS('',3,(#28069,#28070,#28071,#28072,#28073,
#28074,#28075,#28076,#28077,#28078,#28079,#28080,#28081,#28082,#28083,#28084,
#28085,#28086,#28087,#28088,#28089,#28090),.UNSPECIFIED.,.F.,.F.,(4,3,3,
3,3,3,3,4),(133.061082488801,133.534568080551,134.531094708018,135.527621335485,
136.524147962951,137.520674590418,138.517201217885,139.34426779598),
 .UNSPECIFIED.);
#327=B_SPLINE_CURVE_WITH_KNOTS('',3,(#28096,#28097,#28098,#28099,#28100,
#28101,#28102,#28103),.UNSPECIFIED.,.F.,.F.,(4,1,1,1,1,4),(147.65485471872,
148.139569482062,149.136096109529,150.132622736996,151.129149364462,152.053589113585),
 .UNSPECIFIED.);
#328=B_SPLINE_CURVE_WITH_KNOTS('',3,(#28106,#28107,#28108,#28109,#28110,
#28111,#28112),.UNSPECIFIED.,.F.,.F.,(4,1,1,1,4),(147.65485471872,147.824314768092,
148.820841395558,149.817368023025,150.813894650492),.UNSPECIFIED.);
#329=B_SPLINE_CURVE_WITH_KNOTS('',3,(#28117,#28118,#28119,#28120,#28121,
#28122,#28123,#28124,#28125,#28126),.UNSPECIFIED.,.F.,.F.,(4,1,1,1,1,1,
1,4),(141.371669411541,142.160409717261,143.156936344728,144.153462972195,
145.149989599662,146.146516227128,147.143042854595,147.65485471872),
 .UNSPECIFIED.);
#330=B_SPLINE_CURVE_WITH_KNOTS('',3,(#28127,#28128,#28129,#28130,#28131,
#28132,#28133,#28134,#28135,#28136),.UNSPECIFIED.,.F.,.F.,(4,1,1,1,1,1,
1,4),(141.371669411541,141.845155003291,142.841681630758,143.838208258224,
144.834734885691,145.831261513158,146.827788140625,147.65485471872),
 .UNSPECIFIED.);
#331=B_SPLINE_CURVE_WITH_KNOTS('',3,(#28141,#28142,#28143,#28144,#28145,
#28146,#28147,#28148,#28149,#28150,#28151),.UNSPECIFIED.,.F.,.F.,(4,1,1,
1,1,1,1,1,4),(135.088484104361,135.184723324994,136.18124995246,137.177776579927,
138.174303207394,139.170829834861,140.167356462328,141.163883089794,141.371669411541),
 .UNSPECIFIED.);
#332=B_SPLINE_CURVE_WITH_KNOTS('',3,(#28152,#28153,#28154,#28155,#28156,
#28157,#28158,#28159,#28160,#28161),.UNSPECIFIED.,.F.,.F.,(4,1,1,1,1,1,
1,4),(135.088484104361,135.86599523849,136.862521865957,137.859048493424,
138.85557512089,139.852101748357,140.848628375824,141.371669411541),
 .UNSPECIFIED.);
#333=B_SPLINE_CURVE_WITH_KNOTS('',3,(#28166,#28167,#28168,#28169,#28170,
#28171,#28172,#28173,#28174,#28175),.UNSPECIFIED.,.F.,.F.,(4,1,1,1,1,1,
1,4),(128.805298797182,129.205563560193,130.20209018766,131.198616815126,
132.195143442593,133.19167007006,134.188196697527,135.088484104361),
 .UNSPECIFIED.);
#334=B_SPLINE_CURVE_WITH_KNOTS('',3,(#28176,#28177,#28178,#28179,#28180,
#28181,#28182,#28183,#28184,#28185,#28186),.UNSPECIFIED.,.F.,.F.,(4,1,1,
1,1,1,1,1,4),(128.805298797182,128.890308846222,129.886835473689,130.883362101156,
131.879888728623,132.87641535609,133.872941983556,134.869468611023,135.088484104361),
 .UNSPECIFIED.);
#335=B_SPLINE_CURVE_WITH_KNOTS('',3,(#28191,#28192,#28193,#28194,#28195,
#28196,#28197,#28198,#28199,#28200),.UNSPECIFIED.,.F.,.F.,(4,1,1,1,1,1,
1,4),(122.522113490002,123.226403795392,124.222930422859,125.219457050326,
126.215983677792,127.212510305259,128.209036932726,128.805298797182),
 .UNSPECIFIED.);
#336=B_SPLINE_CURVE_WITH_KNOTS('',3,(#28201,#28202,#28203,#28204,#28205,
#28206,#28207,#28208,#28209,#28210),.UNSPECIFIED.,.F.,.F.,(4,1,1,1,1,1,
1,4),(122.522113490002,122.911149081422,123.907675708888,124.904202336355,
125.900728963822,126.897255591289,127.893782218756,128.805298797182),
 .UNSPECIFIED.);
#337=B_SPLINE_CURVE_WITH_KNOTS('',3,(#28215,#28216,#28217,#28218,#28219,
#28220,#28221,#28222,#28223,#28224,#28225),.UNSPECIFIED.,.F.,.F.,(4,1,1,
1,1,1,1,1,4),(116.238928182822,116.250717403124,117.247244030591,118.243770658058,
119.240297285525,120.236823912992,121.233350540458,122.229877167925,122.522113490002),
 .UNSPECIFIED.);
#338=B_SPLINE_CURVE_WITH_KNOTS('',3,(#28226,#28227,#28228,#28229,#28230,
#28231,#28232,#28233,#28234,#28235),.UNSPECIFIED.,.F.,.F.,(4,1,1,1,1,1,
1,4),(116.238928182822,116.931989316621,117.928515944088,118.925042571554,
119.921569199021,120.918095826488,121.914622453955,122.522113490002),
 .UNSPECIFIED.);
#339=B_SPLINE_CURVE_WITH_KNOTS('',3,(#28240,#28241,#28242,#28243,#28244,
#28245,#28246,#28247,#28248,#28249),.UNSPECIFIED.,.F.,.F.,(4,1,1,1,1,1,
1,4),(109.955742875643,110.271557638324,111.26808426579,112.264610893257,
113.261137520724,114.257664148191,115.254190775658,116.238928182822),
 .UNSPECIFIED.);
#340=B_SPLINE_CURVE_WITH_KNOTS('',3,(#28250,#28251,#28252,#28253,#28254,
#28255,#28256,#28257,#28258,#28259,#28260),.UNSPECIFIED.,.F.,.F.,(4,1,1,
1,1,1,1,1,4),(109.955742875643,109.956302924353,110.95282955182,111.949356179287,
112.945882806754,113.94240943422,114.938936061687,115.935462689154,116.238928182822),
 .UNSPECIFIED.);
#341=B_SPLINE_CURVE_WITH_KNOTS('',3,(#28265,#28266,#28267,#28268,#28269,
#28270,#28271,#28272,#28273,#28274),.UNSPECIFIED.,.F.,.F.,(4,1,1,1,1,1,
1,4),(103.672557568463,104.292397873523,105.28892450099,106.285451128456,
107.281977755923,108.27850438339,109.275031010857,109.955742875643),
 .UNSPECIFIED.);
#342=B_SPLINE_CURVE_WITH_KNOTS('',3,(#28275,#28276,#28277,#28278,#28279,
#28280,#28281,#28282,#28283,#28284),.UNSPECIFIED.,.F.,.F.,(4,1,1,1,1,1,
1,4),(103.672557568463,103.977143159552,104.973669787019,105.970196414486,
106.966723041953,107.96324966942,108.959776296886,109.955742875643),
 .UNSPECIFIED.);
#343=B_SPLINE_CURVE_WITH_KNOTS('',3,(#28289,#28290,#28291,#28292,#28293,
#28294,#28295,#28296,#28297,#28298),.UNSPECIFIED.,.F.,.F.,(4,1,1,1,1,1,
1,4),(97.3893722612836,98.313238108722,99.3097647361889,100.306291363656,
101.302817991122,102.299344618589,103.295871246056,103.672557568463),
 .UNSPECIFIED.);
#344=B_SPLINE_CURVE_WITH_KNOTS('',3,(#28299,#28300,#28301,#28302,#28303,
#28304,#28305,#28306,#28307,#28308),.UNSPECIFIED.,.F.,.F.,(4,1,1,1,1,1,
1,4),(97.3893722612836,97.9979833947516,98.9945100222184,99.9910366496852,
100.987563277152,101.984089904619,102.980616532086,103.672557568463),
 .UNSPECIFIED.);
#345=B_SPLINE_CURVE_WITH_KNOTS('',3,(#28313,#28314,#28315,#28316,#28317,
#28318,#28319,#28320,#28321,#28322,#28323),.UNSPECIFIED.,.F.,.F.,(4,1,1,
1,1,1,1,1,4),(91.106186954104,91.3375517164545,92.3340783439213,93.3306049713881,
94.3271315988549,95.3236582263217,96.3201848537885,97.3167114812553,97.3893722612836),
 .UNSPECIFIED.);
#346=B_SPLINE_CURVE_WITH_KNOTS('',3,(#28324,#28325,#28326,#28327,#28328,
#28329,#28330,#28331,#28332,#28333),.UNSPECIFIED.,.F.,.F.,(4,1,1,1,1,1,
1,4),(91.106186954104,92.0188236299508,93.0153502574176,94.0118768848844,
95.0084035123512,96.004930139818,97.0014567672848,97.3893722612836),
 .UNSPECIFIED.);
#347=B_SPLINE_CURVE_WITH_KNOTS('',3,(#28338,#28339,#28340,#28341,#28342,
#28343,#28344,#28345,#28346,#28347),.UNSPECIFIED.,.F.,.F.,(4,1,1,1,1,1,
1,4),(84.8230016469244,85.3583919516537,86.3549185791205,87.3514452065873,
88.3479718340541,89.3444984615209,90.3410250889877,91.106186954104),
 .UNSPECIFIED.);
#348=B_SPLINE_CURVE_WITH_KNOTS('',3,(#28348,#28349,#28350,#28351,#28352,
#28353,#28354,#28355,#28356,#28357,#28358),.UNSPECIFIED.,.F.,.F.,(4,1,1,
1,1,1,1,1,4),(84.8230016469244,85.0431372376832,86.03966386515,87.0361904926168,
88.0327171200836,89.0292437475504,90.0257703750172,91.022297002484,91.106186954104),
 .UNSPECIFIED.);
#349=B_SPLINE_CURVE_WITH_KNOTS('',3,(#28363,#28364,#28365,#28366,#28367,
#28368,#28369,#28370,#28371,#28372),.UNSPECIFIED.,.F.,.F.,(4,1,1,1,1,1,
1,4),(78.5398163397449,79.3792321868529,80.3757588143197,81.3722854417865,
82.3688120692533,83.3653386967201,84.3618653241869,84.8230016469244),
 .UNSPECIFIED.);
#350=B_SPLINE_CURVE_WITH_KNOTS('',3,(#28373,#28374,#28375,#28376,#28377,
#28378,#28379,#28380,#28381,#28382),.UNSPECIFIED.,.F.,.F.,(4,1,1,1,1,1,
1,4),(78.5398163397449,79.0639774728824,80.0605041003492,81.057030727816,
82.0535573552828,83.0500839827496,84.0466106102164,84.8230016469244),
 .UNSPECIFIED.);
#351=B_SPLINE_CURVE_WITH_KNOTS('',3,(#28387,#28388,#28389,#28390,#28391,
#28392,#28393,#28394,#28395,#28396,#28397),.UNSPECIFIED.,.F.,.F.,(4,1,1,
1,1,1,1,1,4),(72.2566310325653,72.4035457945853,73.4000724220521,74.3965990495189,
75.3931256769857,76.3896523044525,77.3861789319193,78.3827055593861,78.5398163397449),
 .UNSPECIFIED.);
#352=B_SPLINE_CURVE_WITH_KNOTS('',3,(#28398,#28399,#28400,#28401,#28402,
#28403,#28404,#28405,#28406,#28407),.UNSPECIFIED.,.F.,.F.,(4,1,1,1,1,1,
1,4),(72.2566310325653,73.0848177080817,74.0813443355485,75.0778709630153,
76.0743975904821,77.0709242179488,78.0674508454156,78.5398163397449),
 .UNSPECIFIED.);
#353=B_SPLINE_CURVE_WITH_KNOTS('',3,(#28412,#28413,#28414,#28415,#28416,
#28417,#28418,#28419,#28420,#28421),.UNSPECIFIED.,.F.,.F.,(4,1,1,1,1,1,
1,4),(65.9734457253856,66.4243860297845,67.4209126572513,68.4174392847181,
69.4139659121849,70.4104925396517,71.4070191671185,72.2566310325653),
 .UNSPECIFIED.);
#354=B_SPLINE_CURVE_WITH_KNOTS('',3,(#28422,#28423,#28424,#28425,#28426,
#28427,#28428,#28429,#28430,#28431,#28432),.UNSPECIFIED.,.F.,.F.,(4,1,1,
1,1,1,1,1,4),(65.9734457253856,66.1091313158141,67.1056579432809,68.1021845707477,
69.0987111982145,70.0952378256813,71.0917644531481,72.0882910806149,72.2566310325653),
 .UNSPECIFIED.);
#355=B_SPLINE_CURVE_WITH_KNOTS('',3,(#28437,#28438,#28439,#28440,#28441,
#28442,#28443,#28444,#28445,#28446),.UNSPECIFIED.,.F.,.F.,(4,1,1,1,1,1,
1,4),(59.6902604182061,60.4452262649837,61.4417528924505,62.4382795199173,
63.4348061473841,64.4313327748509,65.4278594023177,65.9734457253856),
 .UNSPECIFIED.);
#356=B_SPLINE_CURVE_WITH_KNOTS('',3,(#28447,#28448,#28449,#28450,#28451,
#28452,#28453,#28454,#28455,#28456),.UNSPECIFIED.,.F.,.F.,(4,1,1,1,1,1,
1,4),(59.6902604182061,60.1299715510133,61.1264981784801,62.1230248059469,
63.1195514334137,64.1160780608805,65.1126046883473,65.9734457253856),
 .UNSPECIFIED.);
#357=B_SPLINE_CURVE_WITH_KNOTS('',3,(#28461,#28462,#28463,#28464,#28465,
#28466,#28467,#28468,#28469,#28470,#28471),.UNSPECIFIED.,.F.,.F.,(4,1,1,
1,1,1,1,1,4),(53.4070751110265,53.4695398727161,54.4660665001829,55.4625931276497,
56.4591197551165,57.4556463825833,58.4521730100501,59.4486996375169,59.6902604182061),
 .UNSPECIFIED.);
#358=B_SPLINE_CURVE_WITH_KNOTS('',3,(#28472,#28473,#28474,#28475,#28476,
#28477,#28478,#28479,#28480,#28481),.UNSPECIFIED.,.F.,.F.,(4,1,1,1,1,1,
1,4),(53.4070751110265,54.1508117862125,55.1473384136793,56.1438650411461,
57.1403916686129,58.1369182960797,59.1334449235465,59.6902604182061),
 .UNSPECIFIED.);
#359=B_SPLINE_CURVE_WITH_KNOTS('',3,(#28486,#28487,#28488,#28489,#28490,
#28491,#28492,#28493,#28494,#28495),.UNSPECIFIED.,.F.,.F.,(4,1,1,1,1,1,
1,4),(47.1238898038469,47.4903801079154,48.4869067353822,49.483433362849,
50.4799599903158,51.4764866177826,52.4730132452493,53.4070751110265),
 .UNSPECIFIED.);
#360=B_SPLINE_CURVE_WITH_KNOTS('',3,(#28496,#28497,#28498,#28499,#28500,
#28501,#28502,#28503,#28504,#28505,#28506),.UNSPECIFIED.,.F.,.F.,(4,1,1,
1,1,1,1,1,4),(47.1238898038469,47.1751253939449,48.1716520214117,49.1681786488785,
50.1647052763453,51.1612319038121,52.1577585312789,53.1542851587457,53.4070751110265),
 .UNSPECIFIED.);
#361=B_SPLINE_CURVE_WITH_KNOTS('',3,(#28511,#28512,#28513,#28514,#28515,
#28516,#28517,#28518,#28519,#28520),.UNSPECIFIED.,.F.,.F.,(4,1,1,1,1,1,
1,4),(40.8407044966673,41.5112203431146,42.5077469705814,43.5042735980482,
44.500800225515,45.4973268529818,46.4938534804486,47.1238898038469),
 .UNSPECIFIED.);
#362=B_SPLINE_CURVE_WITH_KNOTS('',3,(#28521,#28522,#28523,#28524,#28525,
#28526,#28527,#28528,#28529,#28530),.UNSPECIFIED.,.F.,.F.,(4,1,1,1,1,1,
1,4),(40.8407044966673,41.1959656291441,42.1924922566109,43.1890188840777,
44.1855455115445,45.1820721390113,46.1785987664781,47.1238898038469),
 .UNSPECIFIED.);
#363=B_SPLINE_CURVE_WITH_KNOTS('',3,(#28535,#28536,#28537,#28538,#28539,
#28540,#28541,#28542,#28543,#28544),.UNSPECIFIED.,.F.,.F.,(4,1,1,1,1,1,
1,4),(34.5575191894877,35.5320605783138,36.5285872057806,37.5251138332474,
38.5216404607142,39.518167088181,40.5146937156478,40.8407044966673),
 .UNSPECIFIED.);
#364=B_SPLINE_CURVE_WITH_KNOTS('',3,(#28545,#28546,#28547,#28548,#28549,
#28550,#28551,#28552,#28553,#28554),.UNSPECIFIED.,.F.,.F.,(4,1,1,1,1,1,
1,4),(34.5575191894877,35.2168058643433,36.2133324918101,37.2098591192769,
38.2063857467437,39.2029123742105,40.1994390016773,40.8407044966673),
 .UNSPECIFIED.);
#365=B_SPLINE_CURVE_WITH_KNOTS('',3,(#28559,#28560,#28561,#28562,#28563,
#28564,#28565,#28566,#28567,#28568,#28569),.UNSPECIFIED.,.F.,.F.,(4,1,1,
1,1,1,1,1,4),(28.2743338823081,28.5563741860462,29.552900813513,30.5494274409798,
31.5459540684466,32.5424806959134,33.5390073233802,34.535533950847,34.5575191894877),
 .UNSPECIFIED.);
#366=B_SPLINE_CURVE_WITH_KNOTS('',3,(#28570,#28571,#28572,#28573,#28574,
#28575,#28576,#28577,#28578,#28579),.UNSPECIFIED.,.F.,.F.,(4,1,1,1,1,1,
1,4),(28.2743338823081,29.2376460995425,30.2341727270093,31.2306993544761,
32.2272259819429,33.2237526094097,34.2202792368765,34.5575191894877),
 .UNSPECIFIED.);
#367=B_SPLINE_CURVE_WITH_KNOTS('',3,(#28584,#28585,#28586,#28587,#28588,
#28589,#28590,#28591,#28592,#28593),.UNSPECIFIED.,.F.,.F.,(4,1,1,1,1,1,
1,4),(21.9911485751285,22.5772144212454,23.5737410487122,24.570267676179,
25.5667943036458,26.5633209311126,27.5598475585794,28.2743338823081),
 .UNSPECIFIED.);
#368=B_SPLINE_CURVE_WITH_KNOTS('',3,(#28594,#28595,#28596,#28597,#28598,
#28599,#28600,#28601,#28602,#28603,#28604),.UNSPECIFIED.,.F.,.F.,(4,1,1,
1,1,1,1,1,4),(21.9911485751285,22.2619597072749,23.2584863347417,24.2550129622085,
25.2515395896753,26.2480662171421,27.2445928446089,28.2411194720757,28.2743338823081),
 .UNSPECIFIED.);
#369=B_SPLINE_CURVE_WITH_KNOTS('',3,(#28609,#28610,#28611,#28612,#28613,
#28614,#28615,#28616,#28617,#28618),.UNSPECIFIED.,.F.,.F.,(4,1,1,1,1,1,
1,4),(15.7079632679489,16.5980546564446,17.5945812839114,18.5911079113782,
19.587634538845,20.5841611663118,21.5806877937786,21.9911485751285),
 .UNSPECIFIED.);
#370=B_SPLINE_CURVE_WITH_KNOTS('',3,(#28619,#28620,#28621,#28622,#28623,
#28624,#28625,#28626,#28627,#28628),.UNSPECIFIED.,.F.,.F.,(4,1,1,1,1,1,
1,4),(15.7079632679489,16.2827999424742,17.279326569941,18.2758531974078,
19.2723798248745,20.2689064523413,21.2654330798081,21.9911485751285),
 .UNSPECIFIED.);
#371=B_SPLINE_CURVE_WITH_KNOTS('',3,(#29214,#29215,#29216,#29217,#29218,
#29219,#29220,#29221,#29222,#29223,#29224,#29225,#29226,#29227,#29228,#29229,
#29230,#29231,#29232,#29233,#29234,#29235,#29236,#29237,#29238,#29239,#29240,
#29241,#29242,#29243,#29244,#29245,#29246,#29247,#29248,#29249,#29250,#29251,
#29252,#29253,#29254,#29255,#29256,#29257,#29258,#29259,#29260,#29261,#29262,
#29263,#29264,#29265,#29266,#29267,#29268,#29269,#29270,#29271,#29272,#29273,
#29274,#29275,#29276,#29277,#29278,#29279,#29280,#29281,#29282,#29283,#29284,
#29285,#29286,#29287,#29288,#29289,#29290,#29291,#29292,#29293,#29294,#29295,
#29296,#29297,#29298),.UNSPECIFIED.,.F.,.F.,(4,3,3,3,3,3,3,3,3,3,3,3,3,
3,3,3,3,3,3,3,3,3,3,3,3,3,3,3,4),(-0.364629307890647,-0.350570973320307,
-0.328978052818744,-0.318517199510329,-0.314077304067069,-0.309443350704567,
-0.288121479269547,-0.272860168701457,-0.264083461271192,-0.260314272498768,
-0.239583028334462,-0.219361432489358,-0.206028823048227,-0.194764789032429,
-0.191353184809912,-0.171767825397509,-0.166030994724833,-0.145277120384229,
-0.126464847198481,-0.122930812072354,-0.103474254747116,-0.0841030460574836,
-0.065133557541488,-0.0617046221863798,-0.0585874619642264,-0.0400020264087737,
-0.0217528946302394,-0.00408444113370017,0.),.UNSPECIFIED.);
#372=B_SPLINE_CURVE_WITH_KNOTS('',3,(#29299,#29300,#29301,#29302,#29303,
#29304,#29305),.UNSPECIFIED.,.F.,.F.,(4,3,4),(139.34426779598,139.513727845352,
140.438167594474),.UNSPECIFIED.);
#373=B_SPLINE_CURVE_WITH_KNOTS('',3,(#29307,#29308,#29309,#29310,#29311,
#29312,#29313,#29314,#29315,#29316,#29317,#29318,#29319,#29320,#29321,#29322,
#29323,#29324,#29325,#29326,#29327,#29328,#29329,#29330,#29331,#29332,#29333,
#29334,#29335,#29336,#29337,#29338,#29339,#29340,#29341,#29342,#29343,#29344,
#29345,#29346,#29347,#29348,#29349,#29350,#29351,#29352,#29353,#29354,#29355,
#29356,#29357,#29358,#29359,#29360,#29361,#29362,#29363,#29364,#29365,#29366,
#29367,#29368,#29369,#29370,#29371,#29372,#29373,#29374,#29375,#29376,#29377,
#29378,#29379,#29380,#29381,#29382,#29383,#29384,#29385,#29386,#29387,#29388,
#29389,#29390,#29391,#29392,#29393,#29394),.UNSPECIFIED.,.F.,.F.,(4,3,3,
3,3,3,3,3,3,3,3,3,3,3,3,3,3,3,3,3,3,3,3,3,3,3,3,3,3,4),(-0.366397579005848,
-0.354990427718542,-0.337010231564958,-0.326410787528287,-0.321616430488346,
-0.302809998808161,-0.288326910148396,-0.283342059075868,-0.278582852742593,
-0.25916977354628,-0.239351473889624,-0.226249927799729,-0.21981438558208,
-0.215722421417741,-0.212569226271925,-0.19213662083836,-0.186945289530043,
-0.167235228589776,-0.156543539884273,-0.148369952063709,-0.143888792518516,
-0.123411612445278,-0.102503519065178,-0.081437114422489,-0.0761190075298889,
-0.072239458013529,-0.0505972726117569,-0.0289036910298352,-0.0076720951992491,
0.),.UNSPECIFIED.);
#374=B_SPLINE_CURVE_WITH_KNOTS('',3,(#29395,#29396,#29397,#29398,#29399,
#29400,#29401,#29402,#29403),.UNSPECIFIED.,.F.,.F.,(4,1,1,1,1,1,4),(10.3757270560179,
11.3001668051402,12.296693432607,13.2932200600738,14.2897466875406,15.2862733150074,
15.7079632679489),.UNSPECIFIED.);
#375=B_SPLINE_CURVE_WITH_KNOTS('',3,(#29409,#29410,#29411,#29412,#29413,
#29414,#29415,#29416,#29417,#29418,#29419,#29420,#29421,#29422,#29423,#29424,
#29425,#29426,#29427,#29428,#29429,#29430,#29431,#29432,#29433,#29434,#29435,
#29436,#29437,#29438,#29439,#29440,#29441,#29442,#29443,#29444,#29445,#29446,
#29447,#29448,#29449,#29450,#29451,#29452,#29453,#29454,#29455,#29456,#29457,
#29458,#29459,#29460,#29461,#29462,#29463,#29464,#29465,#29466,#29467,#29468,
#29469,#29470,#29471,#29472,#29473,#29474,#29475,#29476,#29477,#29478,#29479,
#29480,#29481,#29482,#29483,#29484,#29485,#29486,#29487,#29488,#29489,#29490,
#29491,#29492,#29493),.UNSPECIFIED.,.F.,.F.,(4,3,3,3,3,3,3,3,3,3,3,3,3,
3,3,3,3,3,3,3,3,3,3,3,3,3,3,3,4),(-0.364629307890666,-0.350570973320324,
-0.328978052669231,-0.318517197828435,-0.314077299887452,-0.309443349083419,
-0.288121477417662,-0.272860167081056,-0.264083457003318,-0.260314270665685,
-0.239583025704171,-0.219361424327907,-0.206028816927134,-0.194764778888859,
-0.191353179101175,-0.171767814271692,-0.166030994724817,-0.145277120384215,
-0.126464843813837,-0.122930811559716,-0.103474253035366,-0.0841030482674331,
-0.0651335676695573,-0.0617046646810245,-0.0585874714057973,-0.0400020414921941,
-0.0217529178875472,-0.00408447427804078,0.),.UNSPECIFIED.);
#376=B_SPLINE_CURVE_WITH_KNOTS('',3,(#29496,#29497,#29498,#29499,#29500,
#29501,#29502,#29503),.UNSPECIFIED.,.F.,.F.,(4,1,1,1,1,4),(11.6154215191106,
12.6119481465774,13.6084747740442,14.605001401511,15.6015280289778,15.7079632679489),
 .UNSPECIFIED.);
#377=B_SPLINE_CURVE_WITH_KNOTS('',3,(#30089,#30090,#30091,#30092,#30093,
#30094,#30095,#30096,#30097,#30098,#30099,#30100,#30101,#30102,#30103,#30104,
#30105,#30106,#30107,#30108,#30109,#30110,#30111,#30112,#30113,#30114,#30115,
#30116,#30117,#30118,#30119,#30120,#30121,#30122,#30123,#30124,#30125,#30126,
#30127,#30128,#30129,#30130,#30131,#30132,#30133,#30134,#30135,#30136,#30137,
#30138,#30139,#30140,#30141,#30142,#30143,#30144,#30145,#30146,#30147,#30148,
#30149,#30150,#30151,#30152,#30153,#30154,#30155,#30156,#30157,#30158,#30159,
#30160,#30161,#30162,#30163,#30164,#30165,#30166,#30167,#30168,#30169,#30170,
#30171,#30172,#30173,#30174,#30175,#30176),.UNSPECIFIED.,.F.,.F.,(4,3,3,
3,3,3,3,3,3,3,3,3,3,3,3,3,3,3,3,3,3,3,3,3,3,3,3,3,3,4),(-0.366397579005786,
-0.354990427718483,-0.337010225011654,-0.326410775254011,-0.321616427612408,
-0.302809991569146,-0.288326903814256,-0.283342034586426,-0.278582850271486,
-0.259169767533232,-0.239351468146884,-0.226249923492668,-0.219814377104185,
-0.215722361896418,-0.212569123121559,-0.192136517860909,-0.18694528953002,
-0.167235226419274,-0.156543536652707,-0.148369941282216,-0.143888792324927,
-0.123411609583119,-0.102503513459085,-0.0814371085565346,-0.0761189992864274,
-0.0722394608782654,-0.0505972736076427,-0.0289036933900785,-0.00767210533094177,
0.),.UNSPECIFIED.);
#378=B_SPLINE_CURVE_WITH_KNOTS('',3,(#30177,#30178,#30179,#30180),
 .UNSPECIFIED.,.F.,.F.,(4,4),(-142.503307727752,-142.322618506789),
 .UNSPECIFIED.);
#596=SHAPE_REPRESENTATION_RELATIONSHIP('SRR','None',#37246,#609);
#609=ADVANCED_BREP_SHAPE_REPRESENTATION('',(#635),#37176);
#622=STYLED_ITEM('',(#37380),#635);
#635=MANIFOLD_SOLID_BREP('Body1',#14784);
#681=FACE_BOUND('',#2937,.T.);
#804=CYLINDRICAL_SURFACE('',#15849,1.954);
#805=CYLINDRICAL_SURFACE('',#15851,1.954);
#806=CYLINDRICAL_SURFACE('',#15852,1.954);
#807=CYLINDRICAL_SURFACE('',#15853,1.954);
#808=CYLINDRICAL_SURFACE('',#15854,1.954);
#809=CYLINDRICAL_SURFACE('',#15855,1.954);
#810=CYLINDRICAL_SURFACE('',#15856,1.954);
#811=CYLINDRICAL_SURFACE('',#15857,1.954);
#812=CYLINDRICAL_SURFACE('',#15858,1.954);
#813=CYLINDRICAL_SURFACE('',#15859,1.954);
#814=CYLINDRICAL_SURFACE('',#15860,1.954);
#815=CYLINDRICAL_SURFACE('',#15861,1.954);
#816=CYLINDRICAL_SURFACE('',#15862,1.954);
#817=CYLINDRICAL_SURFACE('',#15863,1.954);
#818=CYLINDRICAL_SURFACE('',#15864,1.954);
#819=CYLINDRICAL_SURFACE('',#15865,1.954);
#820=CYLINDRICAL_SURFACE('',#15866,1.954);
#821=CYLINDRICAL_SURFACE('',#15867,1.954);
#822=CYLINDRICAL_SURFACE('',#15868,1.954);
#823=CYLINDRICAL_SURFACE('',#15869,1.954);
#824=CYLINDRICAL_SURFACE('',#15870,1.954);
#825=CYLINDRICAL_SURFACE('',#15871,1.954);
#826=CYLINDRICAL_SURFACE('',#15872,1.954);
#827=CYLINDRICAL_SURFACE('',#15873,1.5555);
#828=CYLINDRICAL_SURFACE('',#15875,1.5555);
#829=CYLINDRICAL_SURFACE('',#15876,1.5555);
#830=CYLINDRICAL_SURFACE('',#15877,1.5555);
#831=CYLINDRICAL_SURFACE('',#15878,1.5555);
#832=CYLINDRICAL_SURFACE('',#15879,1.5555);
#833=CYLINDRICAL_SURFACE('',#15880,1.5555);
#834=CYLINDRICAL_SURFACE('',#15881,1.5555);
#835=CYLINDRICAL_SURFACE('',#15882,1.5555);
#836=CYLINDRICAL_SURFACE('',#15883,1.5555);
#837=CYLINDRICAL_SURFACE('',#15884,1.5555);
#838=CYLINDRICAL_SURFACE('',#15885,1.5555);
#839=CYLINDRICAL_SURFACE('',#15886,1.5555);
#840=CYLINDRICAL_SURFACE('',#15887,1.5555);
#841=CYLINDRICAL_SURFACE('',#15888,1.5555);
#842=CYLINDRICAL_SURFACE('',#15889,1.5555);
#843=CYLINDRICAL_SURFACE('',#15890,1.5555);
#844=CYLINDRICAL_SURFACE('',#15891,1.5555);
#845=CYLINDRICAL_SURFACE('',#15892,1.5555);
#846=CYLINDRICAL_SURFACE('',#15893,1.5555);
#847=CYLINDRICAL_SURFACE('',#15894,1.5555);
#848=CYLINDRICAL_SURFACE('',#15895,1.5555);
#849=CYLINDRICAL_SURFACE('',#15900,1.5555);
#850=CYLINDRICAL_SURFACE('',#15901,1.954);
#1239=CIRCLE('',#15850,1.954);
#1240=CIRCLE('',#15874,1.5555);
#1241=CIRCLE('',#15897,1.954);
#1242=CIRCLE('',#15898,1.954);
#1243=CIRCLE('',#15899,1.5555);
#1244=CIRCLE('',#15902,1.954);
#1245=CIRCLE('',#15904,1.6);
#1246=CIRCLE('',#15907,3.34203030879952);
#1356=CONICAL_SURFACE('',#15905,1.8,0.785398163397448);
#1357=CONICAL_SURFACE('',#15906,3.83322594216369,1.03985037524359);
#1995=FACE_OUTER_BOUND('',#2876,.T.);
#1996=FACE_OUTER_BOUND('',#2877,.T.);
#1997=FACE_OUTER_BOUND('',#2878,.T.);
#1998=FACE_OUTER_BOUND('',#2879,.T.);
#1999=FACE_OUTER_BOUND('',#2880,.T.);
#2000=FACE_OUTER_BOUND('',#2881,.T.);
#2001=FACE_OUTER_BOUND('',#2882,.T.);
#2002=FACE_OUTER_BOUND('',#2883,.T.);
#2003=FACE_OUTER_BOUND('',#2884,.T.);
#2004=FACE_OUTER_BOUND('',#2885,.T.);
#2005=FACE_OUTER_BOUND('',#2886,.T.);
#2006=FACE_OUTER_BOUND('',#2887,.T.);
#2007=FACE_OUTER_BOUND('',#2888,.T.);
#2008=FACE_OUTER_BOUND('',#2889,.T.);
#2009=FACE_OUTER_BOUND('',#2890,.T.);
#2010=FACE_OUTER_BOUND('',#2891,.T.);
#2011=FACE_OUTER_BOUND('',#2892,.T.);
#2012=FACE_OUTER_BOUND('',#2893,.T.);
#2013=FACE_OUTER_BOUND('',#2894,.T.);
#2014=FACE_OUTER_BOUND('',#2895,.T.);
#2015=FACE_OUTER_BOUND('',#2896,.T.);
#2016=FACE_OUTER_BOUND('',#2897,.T.);
#2017=FACE_OUTER_BOUND('',#2898,.T.);
#2018=FACE_OUTER_BOUND('',#2899,.T.);
#2019=FACE_OUTER_BOUND('',#2900,.T.);
#2020=FACE_OUTER_BOUND('',#2901,.T.);
#2021=FACE_OUTER_BOUND('',#2902,.T.);
#2022=FACE_OUTER_BOUND('',#2903,.T.);
#2023=FACE_OUTER_BOUND('',#2904,.T.);
#2024=FACE_OUTER_BOUND('',#2905,.T.);
#2025=FACE_OUTER_BOUND('',#2906,.T.);
#2026=FACE_OUTER_BOUND('',#2907,.T.);
#2027=FACE_OUTER_BOUND('',#2908,.T.);
#2028=FACE_OUTER_BOUND('',#2909,.T.);
#2029=FACE_OUTER_BOUND('',#2910,.T.);
#2030=FACE_OUTER_BOUND('',#2911,.T.);
#2031=FACE_OUTER_BOUND('',#2912,.T.);
#2032=FACE_OUTER_BOUND('',#2913,.T.);
#2033=FACE_OUTER_BOUND('',#2914,.T.);
#2034=FACE_OUTER_BOUND('',#2915,.T.);
#2035=FACE_OUTER_BOUND('',#2916,.T.);
#2036=FACE_OUTER_BOUND('',#2917,.T.);
#2037=FACE_OUTER_BOUND('',#2918,.T.);
#2038=FACE_OUTER_BOUND('',#2919,.T.);
#2039=FACE_OUTER_BOUND('',#2920,.T.);
#2040=FACE_OUTER_BOUND('',#2921,.T.);
#2041=FACE_OUTER_BOUND('',#2922,.T.);
#2042=FACE_OUTER_BOUND('',#2923,.T.);
#2043=FACE_OUTER_BOUND('',#2924,.T.);
#2044=FACE_OUTER_BOUND('',#2925,.T.);
#2045=FACE_OUTER_BOUND('',#2926,.T.);
#2046=FACE_OUTER_BOUND('',#2927,.T.);
#2047=FACE_OUTER_BOUND('',#2928,.T.);
#2048=FACE_OUTER_BOUND('',#2929,.T.);
#2049=FACE_OUTER_BOUND('',#2930,.T.);
#2050=FACE_OUTER_BOUND('',#2931,.T.);
#2051=FACE_OUTER_BOUND('',#2932,.T.);
#2052=FACE_OUTER_BOUND('',#2933,.T.);
#2053=FACE_OUTER_BOUND('',#2934,.T.);
#2054=FACE_OUTER_BOUND('',#2935,.T.);
#2055=FACE_OUTER_BOUND('',#2936,.T.);
#2876=EDGE_LOOP('',(#12285,#12286,#12287,#12288));
#2877=EDGE_LOOP('',(#12289,#12290,#12291,#12292));
#2878=EDGE_LOOP('',(#12293,#12294,#12295,#12296));
#2879=EDGE_LOOP('',(#12297,#12298,#12299,#12300));
#2880=EDGE_LOOP('',(#12301,#12302,#12303,#12304));
#2881=EDGE_LOOP('',(#12305,#12306,#12307,#12308));
#2882=EDGE_LOOP('',(#12309,#12310,#12311,#12312));
#2883=EDGE_LOOP('',(#12313,#12314,#12315,#12316));
#2884=EDGE_LOOP('',(#12317,#12318,#12319,#12320));
#2885=EDGE_LOOP('',(#12321,#12322,#12323,#12324));
#2886=EDGE_LOOP('',(#12325,#12326,#12327,#12328));
#2887=EDGE_LOOP('',(#12329,#12330,#12331,#12332));
#2888=EDGE_LOOP('',(#12333,#12334,#12335,#12336));
#2889=EDGE_LOOP('',(#12337,#12338,#12339,#12340));
#2890=EDGE_LOOP('',(#12341,#12342,#12343,#12344));
#2891=EDGE_LOOP('',(#12345,#12346,#12347,#12348));
#2892=EDGE_LOOP('',(#12349,#12350,#12351,#12352));
#2893=EDGE_LOOP('',(#12353,#12354,#12355,#12356));
#2894=EDGE_LOOP('',(#12357,#12358,#12359,#12360));
#2895=EDGE_LOOP('',(#12361,#12362,#12363,#12364));
#2896=EDGE_LOOP('',(#12365,#12366,#12367,#12368));
#2897=EDGE_LOOP('',(#12369,#12370,#12371,#12372));
#2898=EDGE_LOOP('',(#12373,#12374,#12375,#12376));
#2899=EDGE_LOOP('',(#12377,#12378,#12379,#12380));
#2900=EDGE_LOOP('',(#12381,#12382,#12383,#12384));
#2901=EDGE_LOOP('',(#12385,#12386,#12387,#12388));
#2902=EDGE_LOOP('',(#12389,#12390,#12391,#12392));
#2903=EDGE_LOOP('',(#12393,#12394,#12395,#12396));
#2904=EDGE_LOOP('',(#12397,#12398,#12399,#12400));
#2905=EDGE_LOOP('',(#12401,#12402,#12403,#12404));
#2906=EDGE_LOOP('',(#12405,#12406,#12407,#12408));
#2907=EDGE_LOOP('',(#12409,#12410,#12411,#12412));
#2908=EDGE_LOOP('',(#12413,#12414,#12415,#12416));
#2909=EDGE_LOOP('',(#12417,#12418,#12419,#12420));
#2910=EDGE_LOOP('',(#12421,#12422,#12423,#12424));
#2911=EDGE_LOOP('',(#12425,#12426,#12427,#12428));
#2912=EDGE_LOOP('',(#12429,#12430,#12431,#12432));
#2913=EDGE_LOOP('',(#12433,#12434,#12435,#12436));
#2914=EDGE_LOOP('',(#12437,#12438,#12439,#12440));
#2915=EDGE_LOOP('',(#12441,#12442,#12443,#12444));
#2916=EDGE_LOOP('',(#12445,#12446,#12447,#12448));
#2917=EDGE_LOOP('',(#12449,#12450,#12451,#12452));
#2918=EDGE_LOOP('',(#12453,#12454,#12455,#12456));
#2919=EDGE_LOOP('',(#12457,#12458,#12459,#12460));
#2920=EDGE_LOOP('',(#12461,#12462,#12463,#12464));
#2921=EDGE_LOOP('',(#12465,#12466,#12467,#12468,#12469,#12470,#12471,#12472,
#12473,#12474,#12475,#12476,#12477,#12478,#12479,#12480,#12481,#12482,#12483,
#12484,#12485,#12486,#12487,#12488,#12489,#12490,#12491,#12492,#12493,#12494,
#12495,#12496,#12497,#12498,#12499,#12500,#12501,#12502,#12503,#12504,#12505,
#12506,#12507,#12508,#12509,#12510,#12511,#12512,#12513));
#2922=EDGE_LOOP('',(#12514,#12515,#12516,#12517,#12518));
#2923=EDGE_LOOP('',(#12519,#12520,#12521,#12522));
#2924=EDGE_LOOP('',(#12523,#12524,#12525,#12526,#12527,#12528,#12529,#12530,
#12531,#12532,#12533,#12534,#12535,#12536,#12537,#12538,#12539,#12540,#12541,
#12542,#12543,#12544,#12545,#12546,#12547,#12548,#12549,#12550,#12551,#12552,
#12553,#12554,#12555,#12556,#12557,#12558,#12559,#12560,#12561,#12562,#12563,
#12564,#12565,#12566,#12567,#12568,#12569,#12570,#12571));
#2925=EDGE_LOOP('',(#12572,#12573,#12574,#12575));
#2926=EDGE_LOOP('',(#12576));
#2927=EDGE_LOOP('',(#12577,#12578,#12579,#12580,#12581,#12582));
#2928=EDGE_LOOP('',(#12583,#12584,#12585,#12586,#12587,#12588,#12589,#12590,
#12591,#12592));
#2929=EDGE_LOOP('',(#12593,#12594,#12595,#12596));
#2930=EDGE_LOOP('',(#12597,#12598,#12599,#12600));
#2931=EDGE_LOOP('',(#12601,#12602,#12603,#12604));
#2932=EDGE_LOOP('',(#12605,#12606,#12607,#12608));
#2933=EDGE_LOOP('',(#12609,#12610,#12611,#12612));
#2934=EDGE_LOOP('',(#12613,#12614,#12615,#12616,#12617));
#2935=EDGE_LOOP('',(#12618));
#2936=EDGE_LOOP('',(#12619,#12620,#12621,#12622,#12623,#12624));
#2937=EDGE_LOOP('',(#12625,#12626,#12627,#12628));
#3168=(
BOUNDED_CURVE()
B_SPLINE_CURVE(2,(#30191,#30192,#30193),.UNSPECIFIED.,.F.,.F.)
B_SPLINE_CURVE_WITH_KNOTS((3,3),(0.0476157841635492,0.475541178108418),
 .UNSPECIFIED.)
CURVE()
GEOMETRIC_REPRESENTATION_ITEM()
RATIONAL_B_SPLINE_CURVE((1.03978013844038,1.20063468565316,1.03978013844038))
REPRESENTATION_ITEM('')
);
#3169=(
BOUNDED_CURVE()
B_SPLINE_CURVE(2,(#30195,#30196,#30197),.UNSPECIFIED.,.F.,.F.)
B_SPLINE_CURVE_WITH_KNOTS((3,3),(0.0476157841635493,0.475541178108419),
 .UNSPECIFIED.)
CURVE()
GEOMETRIC_REPRESENTATION_ITEM()
RATIONAL_B_SPLINE_CURVE((1.03978013844038,1.20063468565316,1.03978013844038))
REPRESENTATION_ITEM('')
);
#3170=(
BOUNDED_CURVE()
B_SPLINE_CURVE(2,(#30199,#30200,#30201),.UNSPECIFIED.,.F.,.F.)
B_SPLINE_CURVE_WITH_KNOTS((3,3),(0.0476157841635493,0.475541178108419),
 .UNSPECIFIED.)
CURVE()
GEOMETRIC_REPRESENTATION_ITEM()
RATIONAL_B_SPLINE_CURVE((1.03978013844038,1.20063468565316,1.03978013844038))
REPRESENTATION_ITEM('')
);
#3171=(
BOUNDED_CURVE()
B_SPLINE_CURVE(2,(#30203,#30204,#30205),.UNSPECIFIED.,.F.,.F.)
B_SPLINE_CURVE_WITH_KNOTS((3,3),(0.0476157841635494,0.475541178108419),
 .UNSPECIFIED.)
CURVE()
GEOMETRIC_REPRESENTATION_ITEM()
RATIONAL_B_SPLINE_CURVE((1.03978013844038,1.20063468565316,1.03978013844038))
REPRESENTATION_ITEM('')
);
#3172=(
BOUNDED_CURVE()
B_SPLINE_CURVE(2,(#30207,#30208,#30209),.UNSPECIFIED.,.F.,.F.)
B_SPLINE_CURVE_WITH_KNOTS((3,3),(0.261578481135984,0.475541178108418),
 .UNSPECIFIED.)
CURVE()
GEOMETRIC_REPRESENTATION_ITEM()
RATIONAL_B_SPLINE_CURVE((1.12020741204677,1.12020741204677,1.03978013844038))
REPRESENTATION_ITEM('')
);
#3173=(
BOUNDED_CURVE()
B_SPLINE_CURVE(2,(#30214,#30215,#30216),.UNSPECIFIED.,.F.,.F.)
B_SPLINE_CURVE_WITH_KNOTS((3,3),(0.0476157841635493,0.261578481135984),
 .UNSPECIFIED.)
CURVE()
GEOMETRIC_REPRESENTATION_ITEM()
RATIONAL_B_SPLINE_CURVE((1.03978013844038,1.12020741204677,1.12020741204677))
REPRESENTATION_ITEM('')
);
#3174=(
BOUNDED_CURVE()
B_SPLINE_CURVE(2,(#30217,#30218,#30219),.UNSPECIFIED.,.F.,.F.)
B_SPLINE_CURVE_WITH_KNOTS((3,3),(0.0476157841635491,0.475541178108418),
 .UNSPECIFIED.)
CURVE()
GEOMETRIC_REPRESENTATION_ITEM()
RATIONAL_B_SPLINE_CURVE((1.03978013844038,1.20063468565316,1.03978013844038))
REPRESENTATION_ITEM('')
);
#4241=LINE('',#26981,#5480);
#4242=LINE('',#27005,#5481);
#4243=LINE('',#27053,#5482);
#4244=LINE('',#27101,#5483);
#4245=LINE('',#27155,#5484);
#4246=LINE('',#27203,#5485);
#4247=LINE('',#27251,#5486);
#4248=LINE('',#27299,#5487);
#4249=LINE('',#27353,#5488);
#4250=LINE('',#27401,#5489);
#4251=LINE('',#27449,#5490);
#4252=LINE('',#27503,#5491);
#4253=LINE('',#27551,#5492);
#4254=LINE('',#27599,#5493);
#4255=LINE('',#27653,#5494);
#4256=LINE('',#27701,#5495);
#4257=LINE('',#27749,#5496);
#4258=LINE('',#27797,#5497);
#4259=LINE('',#27848,#5498);
#4260=LINE('',#27896,#5499);
#4261=LINE('',#27944,#5500);
#4262=LINE('',#27998,#5501);
#4263=LINE('',#28046,#5502);
#4264=LINE('',#28094,#5503);
#4265=LINE('',#28116,#5504);
#4266=LINE('',#28140,#5505);
#4267=LINE('',#28165,#5506);
#4268=LINE('',#28190,#5507);
#4269=LINE('',#28214,#5508);
#4270=LINE('',#28239,#5509);
#4271=LINE('',#28264,#5510);
#4272=LINE('',#28288,#5511);
#4273=LINE('',#28312,#5512);
#4274=LINE('',#28337,#5513);
#4275=LINE('',#28362,#5514);
#4276=LINE('',#28386,#5515);
#4277=LINE('',#28411,#5516);
#4278=LINE('',#28436,#5517);
#4279=LINE('',#28460,#5518);
#4280=LINE('',#28485,#5519);
#4281=LINE('',#28510,#5520);
#4282=LINE('',#28534,#5521);
#4283=LINE('',#28558,#5522);
#4284=LINE('',#28583,#5523);
#4285=LINE('',#28608,#5524);
#4286=LINE('',#30187,#5525);
#4287=LINE('',#30211,#5526);
#4288=LINE('',#30222,#5527);
#4289=LINE('',#30224,#5528);
#4290=LINE('',#30225,#5529);
#4291=LINE('',#30228,#5530);
#4292=LINE('',#30229,#5531);
#4293=LINE('',#30232,#5532);
#4294=LINE('',#30233,#5533);
#4295=LINE('',#30236,#5534);
#4296=LINE('',#30237,#5535);
#4297=LINE('',#30240,#5536);
#4298=LINE('',#30241,#5537);
#4299=LINE('',#30243,#5538);
#5480=VECTOR('',#18997,2.);
#5481=VECTOR('',#19002,2.);
#5482=VECTOR('',#19005,2.);
#5483=VECTOR('',#19008,2.);
#5484=VECTOR('',#19011,2.);
#5485=VECTOR('',#19014,2.);
#5486=VECTOR('',#19017,2.);
#5487=VECTOR('',#19020,2.);
#5488=VECTOR('',#19023,2.);
#5489=VECTOR('',#19026,2.);
#5490=VECTOR('',#19029,2.);
#5491=VECTOR('',#19032,2.);
#5492=VECTOR('',#19035,2.);
#5493=VECTOR('',#19038,2.);
#5494=VECTOR('',#19041,2.);
#5495=VECTOR('',#19044,2.);
#5496=VECTOR('',#19047,2.);
#5497=VECTOR('',#19050,2.);
#5498=VECTOR('',#19053,2.);
#5499=VECTOR('',#19056,2.);
#5500=VECTOR('',#19059,2.);
#5501=VECTOR('',#19062,2.);
#5502=VECTOR('',#19065,2.);
#5503=VECTOR('',#19068,1.5555);
#5504=VECTOR('',#19073,1.5555);
#5505=VECTOR('',#19076,1.5555);
#5506=VECTOR('',#19079,1.5555);
#5507=VECTOR('',#19082,1.5555);
#5508=VECTOR('',#19085,1.5555);
#5509=VECTOR('',#19088,1.5555);
#5510=VECTOR('',#19091,1.5555);
#5511=VECTOR('',#19094,1.5555);
#5512=VECTOR('',#19097,1.5555);
#5513=VECTOR('',#19100,1.5555);
#5514=VECTOR('',#19103,1.5555);
#5515=VECTOR('',#19106,1.5555);
#5516=VECTOR('',#19109,1.5555);
#5517=VECTOR('',#19112,1.5555);
#5518=VECTOR('',#19115,1.5555);
#5519=VECTOR('',#19118,1.5555);
#5520=VECTOR('',#19121,1.5555);
#5521=VECTOR('',#19124,1.5555);
#5522=VECTOR('',#19127,1.5555);
#5523=VECTOR('',#19130,1.5555);
#5524=VECTOR('',#19133,1.5555);
#5525=VECTOR('',#19154,1.8);
#5526=VECTOR('',#19157,3.83322594216369);
#5527=VECTOR('',#19162,10.);
#5528=VECTOR('',#19163,10.);
#5529=VECTOR('',#19164,10.);
#5530=VECTOR('',#19167,10.);
#5531=VECTOR('',#19168,10.);
#5532=VECTOR('',#19171,10.);
#5533=VECTOR('',#19172,10.);
#5534=VECTOR('',#19175,10.);
#5535=VECTOR('',#19176,10.);
#5536=VECTOR('',#19179,10.);
#5537=VECTOR('',#19180,10.);
#5538=VECTOR('',#19183,10.);
#6638=VERTEX_POINT('',#26979);
#6639=VERTEX_POINT('',#26980);
#6640=VERTEX_POINT('',#26982);
#6641=VERTEX_POINT('',#26993);
#6642=VERTEX_POINT('',#27003);
#6643=VERTEX_POINT('',#27004);
#6644=VERTEX_POINT('',#27051);
#6645=VERTEX_POINT('',#27052);
#6646=VERTEX_POINT('',#27099);
#6647=VERTEX_POINT('',#27100);
#6648=VERTEX_POINT('',#27153);
#6649=VERTEX_POINT('',#27154);
#6650=VERTEX_POINT('',#27201);
#6651=VERTEX_POINT('',#27202);
#6652=VERTEX_POINT('',#27249);
#6653=VERTEX_POINT('',#27250);
#6654=VERTEX_POINT('',#27297);
#6655=VERTEX_POINT('',#27298);
#6656=VERTEX_POINT('',#27351);
#6657=VERTEX_POINT('',#27352);
#6658=VERTEX_POINT('',#27399);
#6659=VERTEX_POINT('',#27400);
#6660=VERTEX_POINT('',#27447);
#6661=VERTEX_POINT('',#27448);
#6662=VERTEX_POINT('',#27501);
#6663=VERTEX_POINT('',#27502);
#6664=VERTEX_POINT('',#27549);
#6665=VERTEX_POINT('',#27550);
#6666=VERTEX_POINT('',#27597);
#6667=VERTEX_POINT('',#27598);
#6668=VERTEX_POINT('',#27651);
#6669=VERTEX_POINT('',#27652);
#6670=VERTEX_POINT('',#27699);
#6671=VERTEX_POINT('',#27700);
#6672=VERTEX_POINT('',#27747);
#6673=VERTEX_POINT('',#27748);
#6674=VERTEX_POINT('',#27795);
#6675=VERTEX_POINT('',#27796);
#6676=VERTEX_POINT('',#27846);
#6677=VERTEX_POINT('',#27847);
#6678=VERTEX_POINT('',#27894);
#6679=VERTEX_POINT('',#27895);
#6680=VERTEX_POINT('',#27942);
#6681=VERTEX_POINT('',#27943);
#6682=VERTEX_POINT('',#27996);
#6683=VERTEX_POINT('',#27997);
#6684=VERTEX_POINT('',#28044);
#6685=VERTEX_POINT('',#28045);
#6686=VERTEX_POINT('',#28092);
#6687=VERTEX_POINT('',#28093);
#6688=VERTEX_POINT('',#28095);
#6689=VERTEX_POINT('',#28104);
#6690=VERTEX_POINT('',#28114);
#6691=VERTEX_POINT('',#28115);
#6692=VERTEX_POINT('',#28138);
#6693=VERTEX_POINT('',#28139);
#6694=VERTEX_POINT('',#28163);
#6695=VERTEX_POINT('',#28164);
#6696=VERTEX_POINT('',#28188);
#6697=VERTEX_POINT('',#28189);
#6698=VERTEX_POINT('',#28212);
#6699=VERTEX_POINT('',#28213);
#6700=VERTEX_POINT('',#28237);
#6701=VERTEX_POINT('',#28238);
#6702=VERTEX_POINT('',#28262);
#6703=VERTEX_POINT('',#28263);
#6704=VERTEX_POINT('',#28286);
#6705=VERTEX_POINT('',#28287);
#6706=VERTEX_POINT('',#28310);
#6707=VERTEX_POINT('',#28311);
#6708=VERTEX_POINT('',#28335);
#6709=VERTEX_POINT('',#28336);
#6710=VERTEX_POINT('',#28360);
#6711=VERTEX_POINT('',#28361);
#6712=VERTEX_POINT('',#28384);
#6713=VERTEX_POINT('',#28385);
#6714=VERTEX_POINT('',#28409);
#6715=VERTEX_POINT('',#28410);
#6716=VERTEX_POINT('',#28434);
#6717=VERTEX_POINT('',#28435);
#6718=VERTEX_POINT('',#28458);
#6719=VERTEX_POINT('',#28459);
#6720=VERTEX_POINT('',#28483);
#6721=VERTEX_POINT('',#28484);
#6722=VERTEX_POINT('',#28508);
#6723=VERTEX_POINT('',#28509);
#6724=VERTEX_POINT('',#28532);
#6725=VERTEX_POINT('',#28533);
#6726=VERTEX_POINT('',#28556);
#6727=VERTEX_POINT('',#28557);
#6728=VERTEX_POINT('',#28581);
#6729=VERTEX_POINT('',#28582);
#6730=VERTEX_POINT('',#28606);
#6731=VERTEX_POINT('',#28607);
#6732=VERTEX_POINT('',#29213);
#6733=VERTEX_POINT('',#29306);
#6734=VERTEX_POINT('',#29405);
#6735=VERTEX_POINT('',#29408);
#6736=VERTEX_POINT('',#30088);
#6737=VERTEX_POINT('',#30184);
#6738=VERTEX_POINT('',#30189);
#6739=VERTEX_POINT('',#30190);
#6740=VERTEX_POINT('',#30194);
#6741=VERTEX_POINT('',#30198);
#6742=VERTEX_POINT('',#30202);
#6743=VERTEX_POINT('',#30206);
#6744=VERTEX_POINT('',#30210);
#6745=VERTEX_POINT('',#30213);
#6746=VERTEX_POINT('',#30221);
#6747=VERTEX_POINT('',#30223);
#6748=VERTEX_POINT('',#30227);
#6749=VERTEX_POINT('',#30231);
#6750=VERTEX_POINT('',#30235);
#6751=VERTEX_POINT('',#30239);
#8584=EDGE_CURVE('',#6638,#6639,#4241,.T.);
#8585=EDGE_CURVE('',#6638,#6640,#281,.T.);
#8586=EDGE_CURVE('',#6640,#6641,#1239,.T.);
#8587=EDGE_CURVE('',#6641,#6639,#282,.T.);
#8588=EDGE_CURVE('',#6642,#6643,#4242,.T.);
#8589=EDGE_CURVE('',#6642,#6638,#283,.T.);
#8590=EDGE_CURVE('',#6639,#6643,#284,.T.);
#8591=EDGE_CURVE('',#6644,#6645,#4243,.T.);
#8592=EDGE_CURVE('',#6644,#6642,#285,.T.);
#8593=EDGE_CURVE('',#6643,#6645,#286,.T.);
#8594=EDGE_CURVE('',#6646,#6647,#4244,.T.);
#8595=EDGE_CURVE('',#6646,#6644,#287,.T.);
#8596=EDGE_CURVE('',#6645,#6647,#288,.T.);
#8597=EDGE_CURVE('',#6648,#6649,#4245,.T.);
#8598=EDGE_CURVE('',#6648,#6646,#289,.T.);
#8599=EDGE_CURVE('',#6647,#6649,#290,.T.);
#8600=EDGE_CURVE('',#6650,#6651,#4246,.T.);
#8601=EDGE_CURVE('',#6650,#6648,#291,.T.);
#8602=EDGE_CURVE('',#6649,#6651,#292,.T.);
#8603=EDGE_CURVE('',#6652,#6653,#4247,.T.);
#8604=EDGE_CURVE('',#6652,#6650,#293,.T.);
#8605=EDGE_CURVE('',#6651,#6653,#294,.T.);
#8606=EDGE_CURVE('',#6654,#6655,#4248,.T.);
#8607=EDGE_CURVE('',#6654,#6652,#295,.T.);
#8608=EDGE_CURVE('',#6653,#6655,#296,.T.);
#8609=EDGE_CURVE('',#6656,#6657,#4249,.T.);
#8610=EDGE_CURVE('',#6656,#6654,#297,.T.);
#8611=EDGE_CURVE('',#6655,#6657,#298,.T.);
#8612=EDGE_CURVE('',#6658,#6659,#4250,.T.);
#8613=EDGE_CURVE('',#6658,#6656,#299,.T.);
#8614=EDGE_CURVE('',#6657,#6659,#300,.T.);
#8615=EDGE_CURVE('',#6660,#6661,#4251,.T.);
#8616=EDGE_CURVE('',#6660,#6658,#301,.T.);
#8617=EDGE_CURVE('',#6659,#6661,#302,.T.);
#8618=EDGE_CURVE('',#6662,#6663,#4252,.T.);
#8619=EDGE_CURVE('',#6662,#6660,#303,.T.);
#8620=EDGE_CURVE('',#6661,#6663,#304,.T.);
#8621=EDGE_CURVE('',#6664,#6665,#4253,.T.);
#8622=EDGE_CURVE('',#6664,#6662,#305,.T.);
#8623=EDGE_CURVE('',#6663,#6665,#306,.T.);
#8624=EDGE_CURVE('',#6666,#6667,#4254,.T.);
#8625=EDGE_CURVE('',#6666,#6664,#307,.T.);
#8626=EDGE_CURVE('',#6665,#6667,#308,.T.);
#8627=EDGE_CURVE('',#6668,#6669,#4255,.T.);
#8628=EDGE_CURVE('',#6668,#6666,#309,.T.);
#8629=EDGE_CURVE('',#6667,#6669,#310,.T.);
#8630=EDGE_CURVE('',#6670,#6671,#4256,.T.);
#8631=EDGE_CURVE('',#6670,#6668,#311,.T.);
#8632=EDGE_CURVE('',#6669,#6671,#312,.T.);
#8633=EDGE_CURVE('',#6672,#6673,#4257,.T.);
#8634=EDGE_CURVE('',#6672,#6670,#313,.T.);
#8635=EDGE_CURVE('',#6671,#6673,#314,.T.);
#8636=EDGE_CURVE('',#6674,#6675,#4258,.T.);
#8637=EDGE_CURVE('',#6674,#6672,#315,.T.);
#8638=EDGE_CURVE('',#6673,#6675,#316,.T.);
#8639=EDGE_CURVE('',#6676,#6677,#4259,.T.);
#8640=EDGE_CURVE('',#6676,#6674,#317,.T.);
#8641=EDGE_CURVE('',#6675,#6677,#318,.T.);
#8642=EDGE_CURVE('',#6678,#6679,#4260,.T.);
#8643=EDGE_CURVE('',#6678,#6676,#319,.T.);
#8644=EDGE_CURVE('',#6677,#6679,#320,.T.);
#8645=EDGE_CURVE('',#6680,#6681,#4261,.T.);
#8646=EDGE_CURVE('',#6680,#6678,#321,.T.);
#8647=EDGE_CURVE('',#6679,#6681,#322,.T.);
#8648=EDGE_CURVE('',#6682,#6683,#4262,.T.);
#8649=EDGE_CURVE('',#6682,#6680,#323,.T.);
#8650=EDGE_CURVE('',#6681,#6683,#324,.T.);
#8651=EDGE_CURVE('',#6684,#6685,#4263,.T.);
#8652=EDGE_CURVE('',#6684,#6682,#325,.T.);
#8653=EDGE_CURVE('',#6683,#6685,#326,.T.);
#8654=EDGE_CURVE('',#6686,#6687,#4264,.T.);
#8655=EDGE_CURVE('',#6686,#6688,#327,.T.);
#8656=EDGE_CURVE('',#6689,#6688,#1240,.T.);
#8657=EDGE_CURVE('',#6687,#6689,#328,.T.);
#8658=EDGE_CURVE('',#6690,#6691,#4265,.T.);
#8659=EDGE_CURVE('',#6690,#6686,#329,.T.);
#8660=EDGE_CURVE('',#6691,#6687,#330,.T.);
#8661=EDGE_CURVE('',#6692,#6693,#4266,.T.);
#8662=EDGE_CURVE('',#6692,#6690,#331,.T.);
#8663=EDGE_CURVE('',#6693,#6691,#332,.T.);
#8664=EDGE_CURVE('',#6694,#6695,#4267,.T.);
#8665=EDGE_CURVE('',#6694,#6692,#333,.T.);
#8666=EDGE_CURVE('',#6695,#6693,#334,.T.);
#8667=EDGE_CURVE('',#6696,#6697,#4268,.T.);
#8668=EDGE_CURVE('',#6696,#6694,#335,.T.);
#8669=EDGE_CURVE('',#6697,#6695,#336,.T.);
#8670=EDGE_CURVE('',#6698,#6699,#4269,.T.);
#8671=EDGE_CURVE('',#6698,#6696,#337,.T.);
#8672=EDGE_CURVE('',#6699,#6697,#338,.T.);
#8673=EDGE_CURVE('',#6700,#6701,#4270,.T.);
#8674=EDGE_CURVE('',#6700,#6698,#339,.T.);
#8675=EDGE_CURVE('',#6701,#6699,#340,.T.);
#8676=EDGE_CURVE('',#6702,#6703,#4271,.T.);
#8677=EDGE_CURVE('',#6702,#6700,#341,.T.);
#8678=EDGE_CURVE('',#6703,#6701,#342,.T.);
#8679=EDGE_CURVE('',#6704,#6705,#4272,.T.);
#8680=EDGE_CURVE('',#6704,#6702,#343,.T.);
#8681=EDGE_CURVE('',#6705,#6703,#344,.T.);
#8682=EDGE_CURVE('',#6706,#6707,#4273,.T.);
#8683=EDGE_CURVE('',#6706,#6704,#345,.T.);
#8684=EDGE_CURVE('',#6707,#6705,#346,.T.);
#8685=EDGE_CURVE('',#6708,#6709,#4274,.T.);
#8686=EDGE_CURVE('',#6708,#6706,#347,.T.);
#8687=EDGE_CURVE('',#6709,#6707,#348,.T.);
#8688=EDGE_CURVE('',#6710,#6711,#4275,.T.);
#8689=EDGE_CURVE('',#6710,#6708,#349,.T.);
#8690=EDGE_CURVE('',#6711,#6709,#350,.T.);
#8691=EDGE_CURVE('',#6712,#6713,#4276,.T.);
#8692=EDGE_CURVE('',#6712,#6710,#351,.T.);
#8693=EDGE_CURVE('',#6713,#6711,#352,.T.);
#8694=EDGE_CURVE('',#6714,#6715,#4277,.T.);
#8695=EDGE_CURVE('',#6714,#6712,#353,.T.);
#8696=EDGE_CURVE('',#6715,#6713,#354,.T.);
#8697=EDGE_CURVE('',#6716,#6717,#4278,.T.);
#8698=EDGE_CURVE('',#6716,#6714,#355,.T.);
#8699=EDGE_CURVE('',#6717,#6715,#356,.T.);
#8700=EDGE_CURVE('',#6718,#6719,#4279,.T.);
#8701=EDGE_CURVE('',#6718,#6716,#357,.T.);
#8702=EDGE_CURVE('',#6719,#6717,#358,.T.);
#8703=EDGE_CURVE('',#6720,#6721,#4280,.T.);
#8704=EDGE_CURVE('',#6720,#6718,#359,.T.);
#8705=EDGE_CURVE('',#6721,#6719,#360,.T.);
#8706=EDGE_CURVE('',#6722,#6723,#4281,.T.);
#8707=EDGE_CURVE('',#6722,#6720,#361,.T.);
#8708=EDGE_CURVE('',#6723,#6721,#362,.T.);
#8709=EDGE_CURVE('',#6724,#6725,#4282,.T.);
#8710=EDGE_CURVE('',#6724,#6722,#363,.T.);
#8711=EDGE_CURVE('',#6725,#6723,#364,.T.);
#8712=EDGE_CURVE('',#6726,#6727,#4283,.T.);
#8713=EDGE_CURVE('',#6726,#6724,#365,.T.);
#8714=EDGE_CURVE('',#6727,#6725,#366,.T.);
#8715=EDGE_CURVE('',#6728,#6729,#4284,.T.);
#8716=EDGE_CURVE('',#6728,#6726,#367,.T.);
#8717=EDGE_CURVE('',#6729,#6727,#368,.T.);
#8718=EDGE_CURVE('',#6730,#6731,#4285,.T.);
#8719=EDGE_CURVE('',#6730,#6728,#369,.T.);
#8720=EDGE_CURVE('',#6731,#6729,#370,.T.);
#8721=EDGE_CURVE('',#6732,#6689,#371,.T.);
#8722=EDGE_CURVE('',#6685,#6732,#372,.T.);
#8723=EDGE_CURVE('',#6733,#6641,#373,.T.);
#8724=EDGE_CURVE('',#6733,#6731,#374,.T.);
#8725=EDGE_CURVE('',#6641,#6734,#1241,.T.);
#8726=EDGE_CURVE('',#6734,#6640,#1242,.T.);
#8727=EDGE_CURVE('',#6640,#6735,#375,.T.);
#8728=EDGE_CURVE('',#6735,#6733,#1243,.T.);
#8729=EDGE_CURVE('',#6735,#6730,#376,.T.);
#8730=EDGE_CURVE('',#6688,#6736,#377,.T.);
#8731=EDGE_CURVE('',#6736,#6684,#378,.T.);
#8732=EDGE_CURVE('',#6736,#6732,#1244,.F.);
#8733=EDGE_CURVE('',#6737,#6737,#1245,.T.);
#8734=EDGE_CURVE('',#6734,#6737,#4286,.T.);
#8735=EDGE_CURVE('',#6738,#6739,#3168,.T.);
#8736=EDGE_CURVE('',#6740,#6738,#3169,.T.);
#8737=EDGE_CURVE('',#6741,#6740,#3170,.T.);
#8738=EDGE_CURVE('',#6742,#6741,#3171,.T.);
#8739=EDGE_CURVE('',#6743,#6742,#3172,.T.);
#8740=EDGE_CURVE('',#6743,#6744,#4287,.T.);
#8741=EDGE_CURVE('',#6744,#6744,#1246,.T.);
#8742=EDGE_CURVE('',#6745,#6743,#3173,.T.);
#8743=EDGE_CURVE('',#6739,#6745,#3174,.T.);
#8744=EDGE_CURVE('',#6746,#6741,#4288,.T.);
#8745=EDGE_CURVE('',#6746,#6747,#4289,.T.);
#8746=EDGE_CURVE('',#6747,#6742,#4290,.T.);
#8747=EDGE_CURVE('',#6748,#6740,#4291,.T.);
#8748=EDGE_CURVE('',#6748,#6746,#4292,.T.);
#8749=EDGE_CURVE('',#6749,#6738,#4293,.T.);
#8750=EDGE_CURVE('',#6749,#6748,#4294,.T.);
#8751=EDGE_CURVE('',#6750,#6739,#4295,.T.);
#8752=EDGE_CURVE('',#6750,#6749,#4296,.T.);
#8753=EDGE_CURVE('',#6751,#6745,#4297,.T.);
#8754=EDGE_CURVE('',#6751,#6750,#4298,.T.);
#8755=EDGE_CURVE('',#6747,#6751,#4299,.T.);
#12285=ORIENTED_EDGE('',*,*,#8584,.F.);
#12286=ORIENTED_EDGE('',*,*,#8585,.T.);
#12287=ORIENTED_EDGE('',*,*,#8586,.T.);
#12288=ORIENTED_EDGE('',*,*,#8587,.T.);
#12289=ORIENTED_EDGE('',*,*,#8588,.F.);
#12290=ORIENTED_EDGE('',*,*,#8589,.T.);
#12291=ORIENTED_EDGE('',*,*,#8584,.T.);
#12292=ORIENTED_EDGE('',*,*,#8590,.T.);
#12293=ORIENTED_EDGE('',*,*,#8591,.F.);
#12294=ORIENTED_EDGE('',*,*,#8592,.T.);
#12295=ORIENTED_EDGE('',*,*,#8588,.T.);
#12296=ORIENTED_EDGE('',*,*,#8593,.T.);
#12297=ORIENTED_EDGE('',*,*,#8594,.F.);
#12298=ORIENTED_EDGE('',*,*,#8595,.T.);
#12299=ORIENTED_EDGE('',*,*,#8591,.T.);
#12300=ORIENTED_EDGE('',*,*,#8596,.T.);
#12301=ORIENTED_EDGE('',*,*,#8597,.F.);
#12302=ORIENTED_EDGE('',*,*,#8598,.T.);
#12303=ORIENTED_EDGE('',*,*,#8594,.T.);
#12304=ORIENTED_EDGE('',*,*,#8599,.T.);
#12305=ORIENTED_EDGE('',*,*,#8600,.F.);
#12306=ORIENTED_EDGE('',*,*,#8601,.T.);
#12307=ORIENTED_EDGE('',*,*,#8597,.T.);
#12308=ORIENTED_EDGE('',*,*,#8602,.T.);
#12309=ORIENTED_EDGE('',*,*,#8603,.F.);
#12310=ORIENTED_EDGE('',*,*,#8604,.T.);
#12311=ORIENTED_EDGE('',*,*,#8600,.T.);
#12312=ORIENTED_EDGE('',*,*,#8605,.T.);
#12313=ORIENTED_EDGE('',*,*,#8606,.F.);
#12314=ORIENTED_EDGE('',*,*,#8607,.T.);
#12315=ORIENTED_EDGE('',*,*,#8603,.T.);
#12316=ORIENTED_EDGE('',*,*,#8608,.T.);
#12317=ORIENTED_EDGE('',*,*,#8609,.F.);
#12318=ORIENTED_EDGE('',*,*,#8610,.T.);
#12319=ORIENTED_EDGE('',*,*,#8606,.T.);
#12320=ORIENTED_EDGE('',*,*,#8611,.T.);
#12321=ORIENTED_EDGE('',*,*,#8612,.F.);
#12322=ORIENTED_EDGE('',*,*,#8613,.T.);
#12323=ORIENTED_EDGE('',*,*,#8609,.T.);
#12324=ORIENTED_EDGE('',*,*,#8614,.T.);
#12325=ORIENTED_EDGE('',*,*,#8615,.F.);
#12326=ORIENTED_EDGE('',*,*,#8616,.T.);
#12327=ORIENTED_EDGE('',*,*,#8612,.T.);
#12328=ORIENTED_EDGE('',*,*,#8617,.T.);
#12329=ORIENTED_EDGE('',*,*,#8618,.F.);
#12330=ORIENTED_EDGE('',*,*,#8619,.T.);
#12331=ORIENTED_EDGE('',*,*,#8615,.T.);
#12332=ORIENTED_EDGE('',*,*,#8620,.T.);
#12333=ORIENTED_EDGE('',*,*,#8621,.F.);
#12334=ORIENTED_EDGE('',*,*,#8622,.T.);
#12335=ORIENTED_EDGE('',*,*,#8618,.T.);
#12336=ORIENTED_EDGE('',*,*,#8623,.T.);
#12337=ORIENTED_EDGE('',*,*,#8624,.F.);
#12338=ORIENTED_EDGE('',*,*,#8625,.T.);
#12339=ORIENTED_EDGE('',*,*,#8621,.T.);
#12340=ORIENTED_EDGE('',*,*,#8626,.T.);
#12341=ORIENTED_EDGE('',*,*,#8627,.F.);
#12342=ORIENTED_EDGE('',*,*,#8628,.T.);
#12343=ORIENTED_EDGE('',*,*,#8624,.T.);
#12344=ORIENTED_EDGE('',*,*,#8629,.T.);
#12345=ORIENTED_EDGE('',*,*,#8630,.F.);
#12346=ORIENTED_EDGE('',*,*,#8631,.T.);
#12347=ORIENTED_EDGE('',*,*,#8627,.T.);
#12348=ORIENTED_EDGE('',*,*,#8632,.T.);
#12349=ORIENTED_EDGE('',*,*,#8633,.F.);
#12350=ORIENTED_EDGE('',*,*,#8634,.T.);
#12351=ORIENTED_EDGE('',*,*,#8630,.T.);
#12352=ORIENTED_EDGE('',*,*,#8635,.T.);
#12353=ORIENTED_EDGE('',*,*,#8636,.F.);
#12354=ORIENTED_EDGE('',*,*,#8637,.T.);
#12355=ORIENTED_EDGE('',*,*,#8633,.T.);
#12356=ORIENTED_EDGE('',*,*,#8638,.T.);
#12357=ORIENTED_EDGE('',*,*,#8639,.F.);
#12358=ORIENTED_EDGE('',*,*,#8640,.T.);
#12359=ORIENTED_EDGE('',*,*,#8636,.T.);
#12360=ORIENTED_EDGE('',*,*,#8641,.T.);
#12361=ORIENTED_EDGE('',*,*,#8642,.F.);
#12362=ORIENTED_EDGE('',*,*,#8643,.T.);
#12363=ORIENTED_EDGE('',*,*,#8639,.T.);
#12364=ORIENTED_EDGE('',*,*,#8644,.T.);
#12365=ORIENTED_EDGE('',*,*,#8645,.F.);
#12366=ORIENTED_EDGE('',*,*,#8646,.T.);
#12367=ORIENTED_EDGE('',*,*,#8642,.T.);
#12368=ORIENTED_EDGE('',*,*,#8647,.T.);
#12369=ORIENTED_EDGE('',*,*,#8648,.F.);
#12370=ORIENTED_EDGE('',*,*,#8649,.T.);
#12371=ORIENTED_EDGE('',*,*,#8645,.T.);
#12372=ORIENTED_EDGE('',*,*,#8650,.T.);
#12373=ORIENTED_EDGE('',*,*,#8651,.F.);
#12374=ORIENTED_EDGE('',*,*,#8652,.T.);
#12375=ORIENTED_EDGE('',*,*,#8648,.T.);
#12376=ORIENTED_EDGE('',*,*,#8653,.T.);
#12377=ORIENTED_EDGE('',*,*,#8654,.F.);
#12378=ORIENTED_EDGE('',*,*,#8655,.T.);
#12379=ORIENTED_EDGE('',*,*,#8656,.F.);
#12380=ORIENTED_EDGE('',*,*,#8657,.F.);
#12381=ORIENTED_EDGE('',*,*,#8658,.F.);
#12382=ORIENTED_EDGE('',*,*,#8659,.T.);
#12383=ORIENTED_EDGE('',*,*,#8654,.T.);
#12384=ORIENTED_EDGE('',*,*,#8660,.F.);
#12385=ORIENTED_EDGE('',*,*,#8661,.F.);
#12386=ORIENTED_EDGE('',*,*,#8662,.T.);
#12387=ORIENTED_EDGE('',*,*,#8658,.T.);
#12388=ORIENTED_EDGE('',*,*,#8663,.F.);
#12389=ORIENTED_EDGE('',*,*,#8664,.F.);
#12390=ORIENTED_EDGE('',*,*,#8665,.T.);
#12391=ORIENTED_EDGE('',*,*,#8661,.T.);
#12392=ORIENTED_EDGE('',*,*,#8666,.F.);
#12393=ORIENTED_EDGE('',*,*,#8667,.F.);
#12394=ORIENTED_EDGE('',*,*,#8668,.T.);
#12395=ORIENTED_EDGE('',*,*,#8664,.T.);
#12396=ORIENTED_EDGE('',*,*,#8669,.F.);
#12397=ORIENTED_EDGE('',*,*,#8670,.F.);
#12398=ORIENTED_EDGE('',*,*,#8671,.T.);
#12399=ORIENTED_EDGE('',*,*,#8667,.T.);
#12400=ORIENTED_EDGE('',*,*,#8672,.F.);
#12401=ORIENTED_EDGE('',*,*,#8673,.F.);
#12402=ORIENTED_EDGE('',*,*,#8674,.T.);
#12403=ORIENTED_EDGE('',*,*,#8670,.T.);
#12404=ORIENTED_EDGE('',*,*,#8675,.F.);
#12405=ORIENTED_EDGE('',*,*,#8676,.F.);
#12406=ORIENTED_EDGE('',*,*,#8677,.T.);
#12407=ORIENTED_EDGE('',*,*,#8673,.T.);
#12408=ORIENTED_EDGE('',*,*,#8678,.F.);
#12409=ORIENTED_EDGE('',*,*,#8679,.F.);
#12410=ORIENTED_EDGE('',*,*,#8680,.T.);
#12411=ORIENTED_EDGE('',*,*,#8676,.T.);
#12412=ORIENTED_EDGE('',*,*,#8681,.F.);
#12413=ORIENTED_EDGE('',*,*,#8682,.F.);
#12414=ORIENTED_EDGE('',*,*,#8683,.T.);
#12415=ORIENTED_EDGE('',*,*,#8679,.T.);
#12416=ORIENTED_EDGE('',*,*,#8684,.F.);
#12417=ORIENTED_EDGE('',*,*,#8685,.F.);
#12418=ORIENTED_EDGE('',*,*,#8686,.T.);
#12419=ORIENTED_EDGE('',*,*,#8682,.T.);
#12420=ORIENTED_EDGE('',*,*,#8687,.F.);
#12421=ORIENTED_EDGE('',*,*,#8688,.F.);
#12422=ORIENTED_EDGE('',*,*,#8689,.T.);
#12423=ORIENTED_EDGE('',*,*,#8685,.T.);
#12424=ORIENTED_EDGE('',*,*,#8690,.F.);
#12425=ORIENTED_EDGE('',*,*,#8691,.F.);
#12426=ORIENTED_EDGE('',*,*,#8692,.T.);
#12427=ORIENTED_EDGE('',*,*,#8688,.T.);
#12428=ORIENTED_EDGE('',*,*,#8693,.F.);
#12429=ORIENTED_EDGE('',*,*,#8694,.F.);
#12430=ORIENTED_EDGE('',*,*,#8695,.T.);
#12431=ORIENTED_EDGE('',*,*,#8691,.T.);
#12432=ORIENTED_EDGE('',*,*,#8696,.F.);
#12433=ORIENTED_EDGE('',*,*,#8697,.F.);
#12434=ORIENTED_EDGE('',*,*,#8698,.T.);
#12435=ORIENTED_EDGE('',*,*,#8694,.T.);
#12436=ORIENTED_EDGE('',*,*,#8699,.F.);
#12437=ORIENTED_EDGE('',*,*,#8700,.F.);
#12438=ORIENTED_EDGE('',*,*,#8701,.T.);
#12439=ORIENTED_EDGE('',*,*,#8697,.T.);
#12440=ORIENTED_EDGE('',*,*,#8702,.F.);
#12441=ORIENTED_EDGE('',*,*,#8703,.F.);
#12442=ORIENTED_EDGE('',*,*,#8704,.T.);
#12443=ORIENTED_EDGE('',*,*,#8700,.T.);
#12444=ORIENTED_EDGE('',*,*,#8705,.F.);
#12445=ORIENTED_EDGE('',*,*,#8706,.F.);
#12446=ORIENTED_EDGE('',*,*,#8707,.T.);
#12447=ORIENTED_EDGE('',*,*,#8703,.T.);
#12448=ORIENTED_EDGE('',*,*,#8708,.F.);
#12449=ORIENTED_EDGE('',*,*,#8709,.F.);
#12450=ORIENTED_EDGE('',*,*,#8710,.T.);
#12451=ORIENTED_EDGE('',*,*,#8706,.T.);
#12452=ORIENTED_EDGE('',*,*,#8711,.F.);
#12453=ORIENTED_EDGE('',*,*,#8712,.F.);
#12454=ORIENTED_EDGE('',*,*,#8713,.T.);
#12455=ORIENTED_EDGE('',*,*,#8709,.T.);
#12456=ORIENTED_EDGE('',*,*,#8714,.F.);
#12457=ORIENTED_EDGE('',*,*,#8715,.F.);
#12458=ORIENTED_EDGE('',*,*,#8716,.T.);
#12459=ORIENTED_EDGE('',*,*,#8712,.T.);
#12460=ORIENTED_EDGE('',*,*,#8717,.F.);
#12461=ORIENTED_EDGE('',*,*,#8718,.F.);
#12462=ORIENTED_EDGE('',*,*,#8719,.T.);
#12463=ORIENTED_EDGE('',*,*,#8715,.T.);
#12464=ORIENTED_EDGE('',*,*,#8720,.F.);
#12465=ORIENTED_EDGE('',*,*,#8721,.F.);
#12466=ORIENTED_EDGE('',*,*,#8722,.F.);
#12467=ORIENTED_EDGE('',*,*,#8653,.F.);
#12468=ORIENTED_EDGE('',*,*,#8650,.F.);
#12469=ORIENTED_EDGE('',*,*,#8647,.F.);
#12470=ORIENTED_EDGE('',*,*,#8644,.F.);
#12471=ORIENTED_EDGE('',*,*,#8641,.F.);
#12472=ORIENTED_EDGE('',*,*,#8638,.F.);
#12473=ORIENTED_EDGE('',*,*,#8635,.F.);
#12474=ORIENTED_EDGE('',*,*,#8632,.F.);
#12475=ORIENTED_EDGE('',*,*,#8629,.F.);
#12476=ORIENTED_EDGE('',*,*,#8626,.F.);
#12477=ORIENTED_EDGE('',*,*,#8623,.F.);
#12478=ORIENTED_EDGE('',*,*,#8620,.F.);
#12479=ORIENTED_EDGE('',*,*,#8617,.F.);
#12480=ORIENTED_EDGE('',*,*,#8614,.F.);
#12481=ORIENTED_EDGE('',*,*,#8611,.F.);
#12482=ORIENTED_EDGE('',*,*,#8608,.F.);
#12483=ORIENTED_EDGE('',*,*,#8605,.F.);
#12484=ORIENTED_EDGE('',*,*,#8602,.F.);
#12485=ORIENTED_EDGE('',*,*,#8599,.F.);
#12486=ORIENTED_EDGE('',*,*,#8596,.F.);
#12487=ORIENTED_EDGE('',*,*,#8593,.F.);
#12488=ORIENTED_EDGE('',*,*,#8590,.F.);
#12489=ORIENTED_EDGE('',*,*,#8587,.F.);
#12490=ORIENTED_EDGE('',*,*,#8723,.F.);
#12491=ORIENTED_EDGE('',*,*,#8724,.T.);
#12492=ORIENTED_EDGE('',*,*,#8720,.T.);
#12493=ORIENTED_EDGE('',*,*,#8717,.T.);
#12494=ORIENTED_EDGE('',*,*,#8714,.T.);
#12495=ORIENTED_EDGE('',*,*,#8711,.T.);
#12496=ORIENTED_EDGE('',*,*,#8708,.T.);
#12497=ORIENTED_EDGE('',*,*,#8705,.T.);
#12498=ORIENTED_EDGE('',*,*,#8702,.T.);
#12499=ORIENTED_EDGE('',*,*,#8699,.T.);
#12500=ORIENTED_EDGE('',*,*,#8696,.T.);
#12501=ORIENTED_EDGE('',*,*,#8693,.T.);
#12502=ORIENTED_EDGE('',*,*,#8690,.T.);
#12503=ORIENTED_EDGE('',*,*,#8687,.T.);
#12504=ORIENTED_EDGE('',*,*,#8684,.T.);
#12505=ORIENTED_EDGE('',*,*,#8681,.T.);
#12506=ORIENTED_EDGE('',*,*,#8678,.T.);
#12507=ORIENTED_EDGE('',*,*,#8675,.T.);
#12508=ORIENTED_EDGE('',*,*,#8672,.T.);
#12509=ORIENTED_EDGE('',*,*,#8669,.T.);
#12510=ORIENTED_EDGE('',*,*,#8666,.T.);
#12511=ORIENTED_EDGE('',*,*,#8663,.T.);
#12512=ORIENTED_EDGE('',*,*,#8660,.T.);
#12513=ORIENTED_EDGE('',*,*,#8657,.T.);
#12514=ORIENTED_EDGE('',*,*,#8725,.T.);
#12515=ORIENTED_EDGE('',*,*,#8726,.T.);
#12516=ORIENTED_EDGE('',*,*,#8727,.T.);
#12517=ORIENTED_EDGE('',*,*,#8728,.T.);
#12518=ORIENTED_EDGE('',*,*,#8723,.T.);
#12519=ORIENTED_EDGE('',*,*,#8718,.T.);
#12520=ORIENTED_EDGE('',*,*,#8724,.F.);
#12521=ORIENTED_EDGE('',*,*,#8728,.F.);
#12522=ORIENTED_EDGE('',*,*,#8729,.T.);
#12523=ORIENTED_EDGE('',*,*,#8730,.F.);
#12524=ORIENTED_EDGE('',*,*,#8655,.F.);
#12525=ORIENTED_EDGE('',*,*,#8659,.F.);
#12526=ORIENTED_EDGE('',*,*,#8662,.F.);
#12527=ORIENTED_EDGE('',*,*,#8665,.F.);
#12528=ORIENTED_EDGE('',*,*,#8668,.F.);
#12529=ORIENTED_EDGE('',*,*,#8671,.F.);
#12530=ORIENTED_EDGE('',*,*,#8674,.F.);
#12531=ORIENTED_EDGE('',*,*,#8677,.F.);
#12532=ORIENTED_EDGE('',*,*,#8680,.F.);
#12533=ORIENTED_EDGE('',*,*,#8683,.F.);
#12534=ORIENTED_EDGE('',*,*,#8686,.F.);
#12535=ORIENTED_EDGE('',*,*,#8689,.F.);
#12536=ORIENTED_EDGE('',*,*,#8692,.F.);
#12537=ORIENTED_EDGE('',*,*,#8695,.F.);
#12538=ORIENTED_EDGE('',*,*,#8698,.F.);
#12539=ORIENTED_EDGE('',*,*,#8701,.F.);
#12540=ORIENTED_EDGE('',*,*,#8704,.F.);
#12541=ORIENTED_EDGE('',*,*,#8707,.F.);
#12542=ORIENTED_EDGE('',*,*,#8710,.F.);
#12543=ORIENTED_EDGE('',*,*,#8713,.F.);
#12544=ORIENTED_EDGE('',*,*,#8716,.F.);
#12545=ORIENTED_EDGE('',*,*,#8719,.F.);
#12546=ORIENTED_EDGE('',*,*,#8729,.F.);
#12547=ORIENTED_EDGE('',*,*,#8727,.F.);
#12548=ORIENTED_EDGE('',*,*,#8585,.F.);
#12549=ORIENTED_EDGE('',*,*,#8589,.F.);
#12550=ORIENTED_EDGE('',*,*,#8592,.F.);
#12551=ORIENTED_EDGE('',*,*,#8595,.F.);
#12552=ORIENTED_EDGE('',*,*,#8598,.F.);
#12553=ORIENTED_EDGE('',*,*,#8601,.F.);
#12554=ORIENTED_EDGE('',*,*,#8604,.F.);
#12555=ORIENTED_EDGE('',*,*,#8607,.F.);
#12556=ORIENTED_EDGE('',*,*,#8610,.F.);
#12557=ORIENTED_EDGE('',*,*,#8613,.F.);
#12558=ORIENTED_EDGE('',*,*,#8616,.F.);
#12559=ORIENTED_EDGE('',*,*,#8619,.F.);
#12560=ORIENTED_EDGE('',*,*,#8622,.F.);
#12561=ORIENTED_EDGE('',*,*,#8625,.F.);
#12562=ORIENTED_EDGE('',*,*,#8628,.F.);
#12563=ORIENTED_EDGE('',*,*,#8631,.F.);
#12564=ORIENTED_EDGE('',*,*,#8634,.F.);
#12565=ORIENTED_EDGE('',*,*,#8637,.F.);
#12566=ORIENTED_EDGE('',*,*,#8640,.F.);
#12567=ORIENTED_EDGE('',*,*,#8643,.F.);
#12568=ORIENTED_EDGE('',*,*,#8646,.F.);
#12569=ORIENTED_EDGE('',*,*,#8649,.F.);
#12570=ORIENTED_EDGE('',*,*,#8652,.F.);
#12571=ORIENTED_EDGE('',*,*,#8731,.F.);
#12572=ORIENTED_EDGE('',*,*,#8651,.T.);
#12573=ORIENTED_EDGE('',*,*,#8722,.T.);
#12574=ORIENTED_EDGE('',*,*,#8732,.F.);
#12575=ORIENTED_EDGE('',*,*,#8731,.T.);
#12576=ORIENTED_EDGE('',*,*,#8733,.F.);
#12577=ORIENTED_EDGE('',*,*,#8725,.F.);
#12578=ORIENTED_EDGE('',*,*,#8586,.F.);
#12579=ORIENTED_EDGE('',*,*,#8726,.F.);
#12580=ORIENTED_EDGE('',*,*,#8734,.T.);
#12581=ORIENTED_EDGE('',*,*,#8733,.T.);
#12582=ORIENTED_EDGE('',*,*,#8734,.F.);
#12583=ORIENTED_EDGE('',*,*,#8735,.F.);
#12584=ORIENTED_EDGE('',*,*,#8736,.F.);
#12585=ORIENTED_EDGE('',*,*,#8737,.F.);
#12586=ORIENTED_EDGE('',*,*,#8738,.F.);
#12587=ORIENTED_EDGE('',*,*,#8739,.F.);
#12588=ORIENTED_EDGE('',*,*,#8740,.T.);
#12589=ORIENTED_EDGE('',*,*,#8741,.F.);
#12590=ORIENTED_EDGE('',*,*,#8740,.F.);
#12591=ORIENTED_EDGE('',*,*,#8742,.F.);
#12592=ORIENTED_EDGE('',*,*,#8743,.F.);
#12593=ORIENTED_EDGE('',*,*,#8738,.T.);
#12594=ORIENTED_EDGE('',*,*,#8744,.F.);
#12595=ORIENTED_EDGE('',*,*,#8745,.T.);
#12596=ORIENTED_EDGE('',*,*,#8746,.T.);
#12597=ORIENTED_EDGE('',*,*,#8737,.T.);
#12598=ORIENTED_EDGE('',*,*,#8747,.F.);
#12599=ORIENTED_EDGE('',*,*,#8748,.T.);
#12600=ORIENTED_EDGE('',*,*,#8744,.T.);
#12601=ORIENTED_EDGE('',*,*,#8736,.T.);
#12602=ORIENTED_EDGE('',*,*,#8749,.F.);
#12603=ORIENTED_EDGE('',*,*,#8750,.T.);
#12604=ORIENTED_EDGE('',*,*,#8747,.T.);
#12605=ORIENTED_EDGE('',*,*,#8735,.T.);
#12606=ORIENTED_EDGE('',*,*,#8751,.F.);
#12607=ORIENTED_EDGE('',*,*,#8752,.T.);
#12608=ORIENTED_EDGE('',*,*,#8749,.T.);
#12609=ORIENTED_EDGE('',*,*,#8743,.T.);
#12610=ORIENTED_EDGE('',*,*,#8753,.F.);
#12611=ORIENTED_EDGE('',*,*,#8754,.T.);
#12612=ORIENTED_EDGE('',*,*,#8751,.T.);
#12613=ORIENTED_EDGE('',*,*,#8742,.T.);
#12614=ORIENTED_EDGE('',*,*,#8739,.T.);
#12615=ORIENTED_EDGE('',*,*,#8746,.F.);
#12616=ORIENTED_EDGE('',*,*,#8755,.T.);
#12617=ORIENTED_EDGE('',*,*,#8753,.T.);
#12618=ORIENTED_EDGE('',*,*,#8741,.T.);
#12619=ORIENTED_EDGE('',*,*,#8750,.F.);
#12620=ORIENTED_EDGE('',*,*,#8752,.F.);
#12621=ORIENTED_EDGE('',*,*,#8754,.F.);
#12622=ORIENTED_EDGE('',*,*,#8755,.F.);
#12623=ORIENTED_EDGE('',*,*,#8745,.F.);
#12624=ORIENTED_EDGE('',*,*,#8748,.F.);
#12625=ORIENTED_EDGE('',*,*,#8732,.T.);
#12626=ORIENTED_EDGE('',*,*,#8721,.T.);
#12627=ORIENTED_EDGE('',*,*,#8656,.T.);
#12628=ORIENTED_EDGE('',*,*,#8730,.T.);
#13890=PLANE('',#15896);
#13891=PLANE('',#15903);
#13892=PLANE('',#15908);
#13893=PLANE('',#15909);
#13894=PLANE('',#15910);
#13895=PLANE('',#15911);
#13896=PLANE('',#15912);
#13897=PLANE('',#15913);
#13898=PLANE('',#15914);
#13899=PLANE('',#15915);
#14563=ADVANCED_FACE('',(#1995),#804,.T.);
#14564=ADVANCED_FACE('',(#1996),#805,.T.);
#14565=ADVANCED_FACE('',(#1997),#806,.T.);
#14566=ADVANCED_FACE('',(#1998),#807,.T.);
#14567=ADVANCED_FACE('',(#1999),#808,.T.);
#14568=ADVANCED_FACE('',(#2000),#809,.T.);
#14569=ADVANCED_FACE('',(#2001),#810,.T.);
#14570=ADVANCED_FACE('',(#2002),#811,.T.);
#14571=ADVANCED_FACE('',(#2003),#812,.T.);
#14572=ADVANCED_FACE('',(#2004),#813,.T.);
#14573=ADVANCED_FACE('',(#2005),#814,.T.);
#14574=ADVANCED_FACE('',(#2006),#815,.T.);
#14575=ADVANCED_FACE('',(#2007),#816,.T.);
#14576=ADVANCED_FACE('',(#2008),#817,.T.);
#14577=ADVANCED_FACE('',(#2009),#818,.T.);
#14578=ADVANCED_FACE('',(#2010),#819,.T.);
#14579=ADVANCED_FACE('',(#2011),#820,.T.);
#14580=ADVANCED_FACE('',(#2012),#821,.T.);
#14581=ADVANCED_FACE('',(#2013),#822,.T.);
#14582=ADVANCED_FACE('',(#2014),#823,.T.);
#14583=ADVANCED_FACE('',(#2015),#824,.T.);
#14584=ADVANCED_FACE('',(#2016),#825,.T.);
#14585=ADVANCED_FACE('',(#2017),#826,.T.);
#14586=ADVANCED_FACE('',(#2018),#827,.T.);
#14587=ADVANCED_FACE('',(#2019),#828,.T.);
#14588=ADVANCED_FACE('',(#2020),#829,.T.);
#14589=ADVANCED_FACE('',(#2021),#830,.T.);
#14590=ADVANCED_FACE('',(#2022),#831,.T.);
#14591=ADVANCED_FACE('',(#2023),#832,.T.);
#14592=ADVANCED_FACE('',(#2024),#833,.T.);
#14593=ADVANCED_FACE('',(#2025),#834,.T.);
#14594=ADVANCED_FACE('',(#2026),#835,.T.);
#14595=ADVANCED_FACE('',(#2027),#836,.T.);
#14596=ADVANCED_FACE('',(#2028),#837,.T.);
#14597=ADVANCED_FACE('',(#2029),#838,.T.);
#14598=ADVANCED_FACE('',(#2030),#839,.T.);
#14599=ADVANCED_FACE('',(#2031),#840,.T.);
#14600=ADVANCED_FACE('',(#2032),#841,.T.);
#14601=ADVANCED_FACE('',(#2033),#842,.T.);
#14602=ADVANCED_FACE('',(#2034),#843,.T.);
#14603=ADVANCED_FACE('',(#2035),#844,.T.);
#14604=ADVANCED_FACE('',(#2036),#845,.T.);
#14605=ADVANCED_FACE('',(#2037),#846,.T.);
#14606=ADVANCED_FACE('',(#2038),#847,.T.);
#14607=ADVANCED_FACE('',(#2039),#848,.T.);
#14608=ADVANCED_FACE('',(#2040),#114,.F.);
#14609=ADVANCED_FACE('',(#2041),#13890,.T.);
#14610=ADVANCED_FACE('',(#2042),#849,.T.);
#14611=ADVANCED_FACE('',(#2043),#115,.F.);
#14612=ADVANCED_FACE('',(#2044),#850,.T.);
#14613=ADVANCED_FACE('',(#2045),#13891,.T.);
#14614=ADVANCED_FACE('',(#2046),#1356,.T.);
#14615=ADVANCED_FACE('',(#2047),#1357,.T.);
#14616=ADVANCED_FACE('',(#2048),#13892,.T.);
#14617=ADVANCED_FACE('',(#2049),#13893,.T.);
#14618=ADVANCED_FACE('',(#2050),#13894,.T.);
#14619=ADVANCED_FACE('',(#2051),#13895,.T.);
#14620=ADVANCED_FACE('',(#2052),#13896,.T.);
#14621=ADVANCED_FACE('',(#2053),#13897,.T.);
#14622=ADVANCED_FACE('',(#2054),#13898,.T.);
#14623=ADVANCED_FACE('',(#2055,#681),#13899,.F.);
#14784=CLOSED_SHELL('',(#14563,#14564,#14565,#14566,#14567,#14568,#14569,
#14570,#14571,#14572,#14573,#14574,#14575,#14576,#14577,#14578,#14579,#14580,
#14581,#14582,#14583,#14584,#14585,#14586,#14587,#14588,#14589,#14590,#14591,
#14592,#14593,#14594,#14595,#14596,#14597,#14598,#14599,#14600,#14601,#14602,
#14603,#14604,#14605,#14606,#14607,#14608,#14609,#14610,#14611,#14612,#14613,
#14614,#14615,#14616,#14617,#14618,#14619,#14620,#14621,#14622,#14623));
#15848=AXIS2_PLACEMENT_3D('',#26977,#18993,#18994);
#15849=AXIS2_PLACEMENT_3D('',#26978,#18995,#18996);
#15850=AXIS2_PLACEMENT_3D('',#26994,#18998,#18999);
#15851=AXIS2_PLACEMENT_3D('',#27002,#19000,#19001);
#15852=AXIS2_PLACEMENT_3D('',#27050,#19003,#19004);
#15853=AXIS2_PLACEMENT_3D('',#27098,#19006,#19007);
#15854=AXIS2_PLACEMENT_3D('',#27152,#19009,#19010);
#15855=AXIS2_PLACEMENT_3D('',#27200,#19012,#19013);
#15856=AXIS2_PLACEMENT_3D('',#27248,#19015,#19016);
#15857=AXIS2_PLACEMENT_3D('',#27296,#19018,#19019);
#15858=AXIS2_PLACEMENT_3D('',#27350,#19021,#19022);
#15859=AXIS2_PLACEMENT_3D('',#27398,#19024,#19025);
#15860=AXIS2_PLACEMENT_3D('',#27446,#19027,#19028);
#15861=AXIS2_PLACEMENT_3D('',#27500,#19030,#19031);
#15862=AXIS2_PLACEMENT_3D('',#27548,#19033,#19034);
#15863=AXIS2_PLACEMENT_3D('',#27596,#19036,#19037);
#15864=AXIS2_PLACEMENT_3D('',#27650,#19039,#19040);
#15865=AXIS2_PLACEMENT_3D('',#27698,#19042,#19043);
#15866=AXIS2_PLACEMENT_3D('',#27746,#19045,#19046);
#15867=AXIS2_PLACEMENT_3D('',#27794,#19048,#19049);
#15868=AXIS2_PLACEMENT_3D('',#27845,#19051,#19052);
#15869=AXIS2_PLACEMENT_3D('',#27893,#19054,#19055);
#15870=AXIS2_PLACEMENT_3D('',#27941,#19057,#19058);
#15871=AXIS2_PLACEMENT_3D('',#27995,#19060,#19061);
#15872=AXIS2_PLACEMENT_3D('',#28043,#19063,#19064);
#15873=AXIS2_PLACEMENT_3D('',#28091,#19066,#19067);
#15874=AXIS2_PLACEMENT_3D('',#28105,#19069,#19070);
#15875=AXIS2_PLACEMENT_3D('',#28113,#19071,#19072);
#15876=AXIS2_PLACEMENT_3D('',#28137,#19074,#19075);
#15877=AXIS2_PLACEMENT_3D('',#28162,#19077,#19078);
#15878=AXIS2_PLACEMENT_3D('',#28187,#19080,#19081);
#15879=AXIS2_PLACEMENT_3D('',#28211,#19083,#19084);
#15880=AXIS2_PLACEMENT_3D('',#28236,#19086,#19087);
#15881=AXIS2_PLACEMENT_3D('',#28261,#19089,#19090);
#15882=AXIS2_PLACEMENT_3D('',#28285,#19092,#19093);
#15883=AXIS2_PLACEMENT_3D('',#28309,#19095,#19096);
#15884=AXIS2_PLACEMENT_3D('',#28334,#19098,#19099);
#15885=AXIS2_PLACEMENT_3D('',#28359,#19101,#19102);
#15886=AXIS2_PLACEMENT_3D('',#28383,#19104,#19105);
#15887=AXIS2_PLACEMENT_3D('',#28408,#19107,#19108);
#15888=AXIS2_PLACEMENT_3D('',#28433,#19110,#19111);
#15889=AXIS2_PLACEMENT_3D('',#28457,#19113,#19114);
#15890=AXIS2_PLACEMENT_3D('',#28482,#19116,#19117);
#15891=AXIS2_PLACEMENT_3D('',#28507,#19119,#19120);
#15892=AXIS2_PLACEMENT_3D('',#28531,#19122,#19123);
#15893=AXIS2_PLACEMENT_3D('',#28555,#19125,#19126);
#15894=AXIS2_PLACEMENT_3D('',#28580,#19128,#19129);
#15895=AXIS2_PLACEMENT_3D('',#28605,#19131,#19132);
#15896=AXIS2_PLACEMENT_3D('',#29404,#19134,#19135);
#15897=AXIS2_PLACEMENT_3D('',#29406,#19136,#19137);
#15898=AXIS2_PLACEMENT_3D('',#29407,#19138,#19139);
#15899=AXIS2_PLACEMENT_3D('',#29494,#19140,#19141);
#15900=AXIS2_PLACEMENT_3D('',#29495,#19142,#19143);
#15901=AXIS2_PLACEMENT_3D('',#30181,#19144,#19145);
#15902=AXIS2_PLACEMENT_3D('',#30182,#19146,#19147);
#15903=AXIS2_PLACEMENT_3D('',#30183,#19148,#19149);
#15904=AXIS2_PLACEMENT_3D('',#30185,#19150,#19151);
#15905=AXIS2_PLACEMENT_3D('',#30186,#19152,#19153);
#15906=AXIS2_PLACEMENT_3D('',#30188,#19155,#19156);
#15907=AXIS2_PLACEMENT_3D('',#30212,#19158,#19159);
#15908=AXIS2_PLACEMENT_3D('',#30220,#19160,#19161);
#15909=AXIS2_PLACEMENT_3D('',#30226,#19165,#19166);
#15910=AXIS2_PLACEMENT_3D('',#30230,#19169,#19170);
#15911=AXIS2_PLACEMENT_3D('',#30234,#19173,#19174);
#15912=AXIS2_PLACEMENT_3D('',#30238,#19177,#19178);
#15913=AXIS2_PLACEMENT_3D('',#30242,#19181,#19182);
#15914=AXIS2_PLACEMENT_3D('',#30244,#19184,#19185);
#15915=AXIS2_PLACEMENT_3D('',#30245,#19186,#19187);
#18993=DIRECTION('axis',(0.,0.,1.));
#18994=DIRECTION('refdir',(1.,0.,0.));
#18995=DIRECTION('center_axis',(1.,0.,0.));
#18996=DIRECTION('ref_axis',(0.,1.,0.));
#18997=DIRECTION('',(-1.,0.,0.));
#18998=DIRECTION('center_axis',(1.,0.,0.));
#18999=DIRECTION('ref_axis',(0.,1.,0.));
#19000=DIRECTION('center_axis',(1.,0.,0.));
#19001=DIRECTION('ref_axis',(0.,1.,0.));
#19002=DIRECTION('',(-1.,0.,0.));
#19003=DIRECTION('center_axis',(1.,0.,0.));
#19004=DIRECTION('ref_axis',(0.,1.,0.));
#19005=DIRECTION('',(-1.,0.,0.));
#19006=DIRECTION('center_axis',(1.,0.,0.));
#19007=DIRECTION('ref_axis',(0.,1.,0.));
#19008=DIRECTION('',(-1.,0.,0.));
#19009=DIRECTION('center_axis',(1.,0.,0.));
#19010=DIRECTION('ref_axis',(0.,1.,0.));
#19011=DIRECTION('',(-1.,0.,0.));
#19012=DIRECTION('center_axis',(1.,0.,0.));
#19013=DIRECTION('ref_axis',(0.,1.,0.));
#19014=DIRECTION('',(-1.,0.,0.));
#19015=DIRECTION('center_axis',(1.,0.,0.));
#19016=DIRECTION('ref_axis',(0.,1.,0.));
#19017=DIRECTION('',(-1.,0.,0.));
#19018=DIRECTION('center_axis',(1.,0.,0.));
#19019=DIRECTION('ref_axis',(0.,1.,0.));
#19020=DIRECTION('',(-1.,0.,0.));
#19021=DIRECTION('center_axis',(1.,0.,0.));
#19022=DIRECTION('ref_axis',(0.,1.,0.));
#19023=DIRECTION('',(-1.,0.,0.));
#19024=DIRECTION('center_axis',(1.,0.,0.));
#19025=DIRECTION('ref_axis',(0.,1.,0.));
#19026=DIRECTION('',(-1.,0.,0.));
#19027=DIRECTION('center_axis',(1.,0.,0.));
#19028=DIRECTION('ref_axis',(0.,1.,0.));
#19029=DIRECTION('',(-1.,0.,0.));
#19030=DIRECTION('center_axis',(1.,0.,0.));
#19031=DIRECTION('ref_axis',(0.,1.,0.));
#19032=DIRECTION('',(-1.,0.,0.));
#19033=DIRECTION('center_axis',(1.,0.,0.));
#19034=DIRECTION('ref_axis',(0.,1.,0.));
#19035=DIRECTION('',(-1.,0.,0.));
#19036=DIRECTION('center_axis',(1.,0.,0.));
#19037=DIRECTION('ref_axis',(0.,1.,0.));
#19038=DIRECTION('',(-1.,0.,0.));
#19039=DIRECTION('center_axis',(1.,0.,0.));
#19040=DIRECTION('ref_axis',(0.,1.,0.));
#19041=DIRECTION('',(-1.,0.,0.));
#19042=DIRECTION('center_axis',(1.,0.,0.));
#19043=DIRECTION('ref_axis',(0.,1.,0.));
#19044=DIRECTION('',(-1.,0.,0.));
#19045=DIRECTION('center_axis',(1.,0.,0.));
#19046=DIRECTION('ref_axis',(0.,1.,0.));
#19047=DIRECTION('',(-1.,0.,0.));
#19048=DIRECTION('center_axis',(1.,0.,0.));
#19049=DIRECTION('ref_axis',(0.,1.,0.));
#19050=DIRECTION('',(-1.,0.,0.));
#19051=DIRECTION('center_axis',(1.,0.,0.));
#19052=DIRECTION('ref_axis',(0.,1.,0.));
#19053=DIRECTION('',(-1.,0.,0.));
#19054=DIRECTION('center_axis',(1.,0.,0.));
#19055=DIRECTION('ref_axis',(0.,1.,0.));
#19056=DIRECTION('',(-1.,0.,0.));
#19057=DIRECTION('center_axis',(1.,0.,0.));
#19058=DIRECTION('ref_axis',(0.,1.,0.));
#19059=DIRECTION('',(-1.,0.,0.));
#19060=DIRECTION('center_axis',(1.,0.,0.));
#19061=DIRECTION('ref_axis',(0.,1.,0.));
#19062=DIRECTION('',(-1.,0.,0.));
#19063=DIRECTION('center_axis',(1.,0.,0.));
#19064=DIRECTION('ref_axis',(0.,1.,0.));
#19065=DIRECTION('',(-1.,0.,0.));
#19066=DIRECTION('center_axis',(1.,0.,0.));
#19067=DIRECTION('ref_axis',(0.,1.,4.93993055488555E-14));
#19068=DIRECTION('',(1.,0.,0.));
#19069=DIRECTION('center_axis',(1.,0.,0.));
#19070=DIRECTION('ref_axis',(0.,1.,4.93993055488555E-14));
#19071=DIRECTION('center_axis',(1.,0.,0.));
#19072=DIRECTION('ref_axis',(0.,1.,4.93993055488555E-14));
#19073=DIRECTION('',(1.,0.,0.));
#19074=DIRECTION('center_axis',(1.,0.,0.));
#19075=DIRECTION('ref_axis',(0.,1.,4.93993055488555E-14));
#19076=DIRECTION('',(1.,0.,0.));
#19077=DIRECTION('center_axis',(1.,0.,0.));
#19078=DIRECTION('ref_axis',(0.,1.,4.93993055488555E-14));
#19079=DIRECTION('',(1.,0.,0.));
#19080=DIRECTION('center_axis',(1.,0.,0.));
#19081=DIRECTION('ref_axis',(0.,1.,4.93993055488555E-14));
#19082=DIRECTION('',(1.,0.,0.));
#19083=DIRECTION('center_axis',(1.,0.,0.));
#19084=DIRECTION('ref_axis',(0.,1.,4.93993055488555E-14));
#19085=DIRECTION('',(1.,0.,0.));
#19086=DIRECTION('center_axis',(1.,0.,0.));
#19087=DIRECTION('ref_axis',(0.,1.,4.93993055488555E-14));
#19088=DIRECTION('',(1.,0.,0.));
#19089=DIRECTION('center_axis',(1.,0.,0.));
#19090=DIRECTION('ref_axis',(0.,1.,4.93993055488555E-14));
#19091=DIRECTION('',(1.,0.,0.));
#19092=DIRECTION('center_axis',(1.,0.,0.));
#19093=DIRECTION('ref_axis',(0.,1.,4.93993055488555E-14));
#19094=DIRECTION('',(1.,0.,0.));
#19095=DIRECTION('center_axis',(1.,0.,0.));
#19096=DIRECTION('ref_axis',(0.,1.,4.93993055488555E-14));
#19097=DIRECTION('',(1.,0.,0.));
#19098=DIRECTION('center_axis',(1.,0.,0.));
#19099=DIRECTION('ref_axis',(0.,1.,4.93993055488555E-14));
#19100=DIRECTION('',(1.,0.,0.));
#19101=DIRECTION('center_axis',(1.,0.,0.));
#19102=DIRECTION('ref_axis',(0.,1.,4.93993055488555E-14));
#19103=DIRECTION('',(1.,0.,0.));
#19104=DIRECTION('center_axis',(1.,0.,0.));
#19105=DIRECTION('ref_axis',(0.,1.,4.93993055488555E-14));
#19106=DIRECTION('',(1.,0.,0.));
#19107=DIRECTION('center_axis',(1.,0.,0.));
#19108=DIRECTION('ref_axis',(0.,1.,4.93993055488555E-14));
#19109=DIRECTION('',(1.,0.,0.));
#19110=DIRECTION('center_axis',(1.,0.,0.));
#19111=DIRECTION('ref_axis',(0.,1.,4.93993055488555E-14));
#19112=DIRECTION('',(1.,0.,0.));
#19113=DIRECTION('center_axis',(1.,0.,0.));
#19114=DIRECTION('ref_axis',(0.,1.,4.93993055488555E-14));
#19115=DIRECTION('',(1.,0.,0.));
#19116=DIRECTION('center_axis',(1.,0.,0.));
#19117=DIRECTION('ref_axis',(0.,1.,4.93993055488555E-14));
#19118=DIRECTION('',(1.,0.,0.));
#19119=DIRECTION('center_axis',(1.,0.,0.));
#19120=DIRECTION('ref_axis',(0.,1.,4.93993055488555E-14));
#19121=DIRECTION('',(1.,0.,0.));
#19122=DIRECTION('center_axis',(1.,0.,0.));
#19123=DIRECTION('ref_axis',(0.,1.,4.93993055488555E-14));
#19124=DIRECTION('',(1.,0.,0.));
#19125=DIRECTION('center_axis',(1.,0.,0.));
#19126=DIRECTION('ref_axis',(0.,1.,4.93993055488555E-14));
#19127=DIRECTION('',(1.,0.,0.));
#19128=DIRECTION('center_axis',(1.,0.,0.));
#19129=DIRECTION('ref_axis',(0.,1.,4.93993055488555E-14));
#19130=DIRECTION('',(1.,0.,0.));
#19131=DIRECTION('center_axis',(1.,0.,0.));
#19132=DIRECTION('ref_axis',(0.,1.,4.93993055488555E-14));
#19133=DIRECTION('',(1.,0.,0.));
#19134=DIRECTION('center_axis',(1.,0.,0.));
#19135=DIRECTION('ref_axis',(0.,0.,-1.));
#19136=DIRECTION('center_axis',(1.,0.,0.));
#19137=DIRECTION('ref_axis',(0.,1.,0.));
#19138=DIRECTION('center_axis',(1.,0.,0.));
#19139=DIRECTION('ref_axis',(0.,1.,0.));
#19140=DIRECTION('center_axis',(-1.,0.,0.));
#19141=DIRECTION('ref_axis',(0.,1.,4.93993055488555E-14));
#19142=DIRECTION('center_axis',(1.,0.,0.));
#19143=DIRECTION('ref_axis',(0.,1.,4.93993055488555E-14));
#19144=DIRECTION('center_axis',(1.,0.,0.));
#19145=DIRECTION('ref_axis',(0.,1.,0.));
#19146=DIRECTION('center_axis',(-1.,0.,0.));
#19147=DIRECTION('ref_axis',(0.,1.,0.));
#19148=DIRECTION('center_axis',(-1.,0.,0.));
#19149=DIRECTION('ref_axis',(0.,0.,1.));
#19150=DIRECTION('center_axis',(1.,0.,0.));
#19151=DIRECTION('ref_axis',(0.,0.,-1.));
#19152=DIRECTION('center_axis',(1.,0.,0.));
#19153=DIRECTION('ref_axis',(0.,1.,0.));
#19154=DIRECTION('',(-0.707106781186548,0.707106781186547,8.65956056235493E-17));
#19155=DIRECTION('center_axis',(-1.,0.,0.));
#19156=DIRECTION('ref_axis',(0.,1.,0.));
#19157=DIRECTION('',(0.506349288588207,0.862328474507375,1.05604780611908E-16));
#19158=DIRECTION('center_axis',(1.,0.,0.));
#19159=DIRECTION('ref_axis',(0.,1.,0.));
#19160=DIRECTION('center_axis',(0.,-0.5,0.866025403784439));
#19161=DIRECTION('ref_axis',(0.,-0.866025403784439,-0.5));
#19162=DIRECTION('',(1.,0.,0.));
#19163=DIRECTION('',(0.,-0.866025403784439,-0.5));
#19164=DIRECTION('',(1.,0.,0.));
#19165=DIRECTION('center_axis',(0.,0.5,0.866025403784439));
#19166=DIRECTION('ref_axis',(0.,-0.866025403784439,0.5));
#19167=DIRECTION('',(1.,0.,0.));
#19168=DIRECTION('',(0.,-0.866025403784439,0.5));
#19169=DIRECTION('center_axis',(0.,1.,-2.74708955197652E-16));
#19170=DIRECTION('ref_axis',(0.,2.74708955197652E-16,1.));
#19171=DIRECTION('',(1.,0.,0.));
#19172=DIRECTION('',(0.,2.74708955197652E-16,1.));
#19173=DIRECTION('center_axis',(0.,0.5,-0.866025403784439));
#19174=DIRECTION('ref_axis',(0.,0.866025403784439,0.5));
#19175=DIRECTION('',(1.,0.,0.));
#19176=DIRECTION('',(0.,0.866025403784439,0.5));
#19177=DIRECTION('center_axis',(0.,-0.5,-0.866025403784439));
#19178=DIRECTION('ref_axis',(0.,0.866025403784439,-0.5));
#19179=DIRECTION('',(1.,0.,0.));
#19180=DIRECTION('',(0.,0.866025403784439,-0.5));
#19181=DIRECTION('center_axis',(0.,-1.,-1.37354477598826E-16));
#19182=DIRECTION('ref_axis',(0.,1.37354477598826E-16,-1.));
#19183=DIRECTION('',(0.,1.37354477598826E-16,-1.));
#19184=DIRECTION('center_axis',(1.,0.,0.));
#19185=DIRECTION('ref_axis',(0.,0.,-1.));
#19186=DIRECTION('center_axis',(1.,0.,0.));
#19187=DIRECTION('ref_axis',(0.,0.,-1.));
#26977=CARTESIAN_POINT('',(0.,0.,0.));
#26978=CARTESIAN_POINT('Origin',(-7.7,0.,0.));
#26979=CARTESIAN_POINT('',(-15.4201303078758,-1.95627805222981,0.00129796472068854));
#26980=CARTESIAN_POINT('',(-15.5218696921242,-1.95584014130724,0.00207447844652431));
#26981=CARTESIAN_POINT('',(-7.7,-1.954,-2.39295984553393E-16));
#26982=CARTESIAN_POINT('',(-15.646,0.8625464214531,1.75510199459808));
#26983=CARTESIAN_POINT('Ctrl Pts',(-15.4201303078758,-1.95627805222981,
0.00129796472068854));
#26984=CARTESIAN_POINT('Ctrl Pts',(-15.4240829032361,-1.9567658369566,0.0703871063130427));
#26985=CARTESIAN_POINT('Ctrl Pts',(-15.4280354985964,-1.95342314936077,
0.139425514587532));
#26986=CARTESIAN_POINT('Ctrl Pts',(-15.4319880939568,-1.94609376501883,
0.20803425151521));
#26987=CARTESIAN_POINT('Ctrl Pts',(-15.4689952596497,-1.8774705653127,0.850400763642468));
#26988=CARTESIAN_POINT('Ctrl Pts',(-15.5060024253426,-1.45936912727697,
1.4551018111239));
#26989=CARTESIAN_POINT('Ctrl Pts',(-15.5430095910356,-0.882640818020853,
1.74666960837442));
#26990=CARTESIAN_POINT('Ctrl Pts',(-15.5773397273571,-0.347631959425933,
2.01714593475978));
#26991=CARTESIAN_POINT('Ctrl Pts',(-15.6116698636785,0.323884289759532,
2.01815339646098));
#26992=CARTESIAN_POINT('Ctrl Pts',(-15.646,0.863566983235696,1.7563826775686));
#26993=CARTESIAN_POINT('',(-15.646,-0.861525859670576,1.75382131162752));
#26994=CARTESIAN_POINT('Origin',(-15.646,0.,0.));
#26995=CARTESIAN_POINT('Ctrl Pts',(-15.646,-0.861525859670577,1.75382131162752));
#26996=CARTESIAN_POINT('Ctrl Pts',(-15.6089928343071,-1.44410240528909,
1.4676434918232));
#26997=CARTESIAN_POINT('Ctrl Pts',(-15.5719856686141,-1.86790219595322,
0.87091756707116));
#26998=CARTESIAN_POINT('Ctrl Pts',(-15.5349785029212,-1.94344388370824,
0.230308838951939));
#26999=CARTESIAN_POINT('Ctrl Pts',(-15.5306088993222,-1.95236343278762,
0.154669266141868));
#27000=CARTESIAN_POINT('Ctrl Pts',(-15.5262392957232,-1.95642770878322,
0.0784178971029367));
#27001=CARTESIAN_POINT('Ctrl Pts',(-15.5218696921242,-1.95584014130724,
0.00207447844652431));
#27002=CARTESIAN_POINT('Origin',(-7.7,0.,0.));
#27003=CARTESIAN_POINT('',(-14.7201303078758,-1.95121230271199,0.000898656016518479));
#27004=CARTESIAN_POINT('',(-14.8218696921242,-1.95111217225575,0.000805047651922751));
#27005=CARTESIAN_POINT('',(-7.7,-1.954,-2.39295984553393E-16));
#27006=CARTESIAN_POINT('Ctrl Pts',(-14.7201303078758,-1.95121230271199,
0.000898656016518479));
#27007=CARTESIAN_POINT('Ctrl Pts',(-14.7353732424118,-1.95232561653816,
0.269132749016255));
#27008=CARTESIAN_POINT('Ctrl Pts',(-14.7506161769478,-1.90081399086995,
0.536957184421699));
#27009=CARTESIAN_POINT('Ctrl Pts',(-14.7658591114838,-1.7946187287383,0.78098321012694));
#27010=CARTESIAN_POINT('Ctrl Pts',(-14.8028662771768,-1.53679529898949,
1.37343550632542));
#27011=CARTESIAN_POINT('Ctrl Pts',(-14.8398734428697,-0.956648445347352,
1.82561211140535));
#27012=CARTESIAN_POINT('Ctrl Pts',(-14.8768806085626,-0.319173913014248,
1.93098415809826));
#27013=CARTESIAN_POINT('Ctrl Pts',(-14.9138877742556,0.318300619318858,
2.03635620479117));
#27014=CARTESIAN_POINT('Ctrl Pts',(-14.9508949399485,1.01310283034293,1.79492369309705));
#27015=CARTESIAN_POINT('Ctrl Pts',(-14.9879021056415,1.447857066046,1.31693812925936));
#27016=CARTESIAN_POINT('Ctrl Pts',(-15.0249092713344,1.88261130174908,0.838952565421676));
#27017=CARTESIAN_POINT('Ctrl Pts',(-15.0619164370273,2.05731756213117,0.124413949440425));
#27018=CARTESIAN_POINT('Ctrl Pts',(-15.0989236027203,1.89218361321693,-0.500235697810672));
#27019=CARTESIAN_POINT('Ctrl Pts',(-15.1359307684132,1.72704966430269,-1.12488534506177));
#27020=CARTESIAN_POINT('Ctrl Pts',(-15.1729379341062,1.22207550609213,-1.65964602358271));
#27021=CARTESIAN_POINT('Ctrl Pts',(-15.2099450997991,0.607903721093593,
-1.86035794818561));
#27022=CARTESIAN_POINT('Ctrl Pts',(-15.2469522654921,-0.00626806390494887,
-2.06106987278851));
#27023=CARTESIAN_POINT('Ctrl Pts',(-15.283959431185,-0.729637475691471,
-1.92773304347336));
#27024=CARTESIAN_POINT('Ctrl Pts',(-15.3209665968779,-1.23174970089647,
-1.52104864042925));
#27025=CARTESIAN_POINT('Ctrl Pts',(-15.3540211672105,-1.68023321894303,
-1.1578006598858));
#27026=CARTESIAN_POINT('Ctrl Pts',(-15.3870757375432,-1.95219883007605,
-0.576477315011743));
#27027=CARTESIAN_POINT('Ctrl Pts',(-15.4201303078758,-1.95627805222981,
0.00129796472068854));
#27028=CARTESIAN_POINT('Ctrl Pts',(-15.5218696921242,-1.95584014130724,
0.00207447844652431));
#27029=CARTESIAN_POINT('Ctrl Pts',(-15.4892321300303,-1.95145146632858,
-0.568151861409059));
#27030=CARTESIAN_POINT('Ctrl Pts',(-15.4565945679363,-1.68753944404723,
-1.14351359006107));
#27031=CARTESIAN_POINT('Ctrl Pts',(-15.4239570058423,-1.24887387924439,
-1.50743054347954));
#27032=CARTESIAN_POINT('Ctrl Pts',(-15.3869498401494,-0.751478602179619,
-1.92006966630539));
#27033=CARTESIAN_POINT('Ctrl Pts',(-15.3499426744565,-0.0294044632041637,
-2.06085638047067));
#27034=CARTESIAN_POINT('Ctrl Pts',(-15.3129355087635,0.587041512969193,
-1.86689340445069));
#27035=CARTESIAN_POINT('Ctrl Pts',(-15.2759283430706,1.20348748914255,-1.67293042843072));
#27036=CARTESIAN_POINT('Ctrl Pts',(-15.2389211773776,1.71430530251381,-1.14421776222549));
#27037=CARTESIAN_POINT('Ctrl Pts',(-15.2019140116847,1.88641226529163,-0.521543698302765));
#27038=CARTESIAN_POINT('Ctrl Pts',(-15.1649068459917,2.05851922806946,0.10113036561996));
#27039=CARTESIAN_POINT('Ctrl Pts',(-15.1278996802988,1.89191534025386,0.817765827260178));
#27040=CARTESIAN_POINT('Ctrl Pts',(-15.0908925146059,1.46257189903353,1.30064584196409));
#27041=CARTESIAN_POINT('Ctrl Pts',(-15.0538853489129,1.03322845781319,1.78352585666799));
#27042=CARTESIAN_POINT('Ctrl Pts',(-15.01687818322,0.341145463188129,2.03265042443559));
#27043=CARTESIAN_POINT('Ctrl Pts',(-14.979871017527,-0.297480529695576,
1.93442073680281));
#27044=CARTESIAN_POINT('Ctrl Pts',(-14.9428638518341,-0.936106522579279,
1.83619104917002));
#27045=CARTESIAN_POINT('Ctrl Pts',(-14.9058566861412,-1.52127551372162,
1.39060710613685));
#27046=CARTESIAN_POINT('Ctrl Pts',(-14.8688495204482,-1.78573084508169,
0.801099057527319));
#27047=CARTESIAN_POINT('Ctrl Pts',(-14.8531895776736,-1.89763769549855,
0.551642982370853));
#27048=CARTESIAN_POINT('Ctrl Pts',(-14.8375296348989,-1.95211622085639,
0.276415256812969));
#27049=CARTESIAN_POINT('Ctrl Pts',(-14.8218696921242,-1.95111217225575,
0.000805047651922751));
#27050=CARTESIAN_POINT('Origin',(-7.7,0.,0.));
#27051=CARTESIAN_POINT('',(-14.0201303078758,-1.9530433091271,-0.00171791376288949));
#27052=CARTESIAN_POINT('',(-14.1218696921242,-1.95325151398278,-0.00174533096842624));
#27053=CARTESIAN_POINT('',(-7.7,-1.954,-2.39295984553393E-16));
#27054=CARTESIAN_POINT('Ctrl Pts',(-14.0201303078758,-1.9530433091271,-0.00171791376288949));
#27055=CARTESIAN_POINT('Ctrl Pts',(-14.0466635815875,-1.94908819668861,
0.464092547322558));
#27056=CARTESIAN_POINT('Ctrl Pts',(-14.0731968552992,-1.78205766518633,
0.932451059956011));
#27057=CARTESIAN_POINT('Ctrl Pts',(-14.0997301290109,-1.4785191386022,1.28240795655502));
#27058=CARTESIAN_POINT('Ctrl Pts',(-14.1367372947038,-1.05516012645965,
1.770508784163));
#27059=CARTESIAN_POINT('Ctrl Pts',(-14.1737444603967,-0.36625003980843,
2.02828115120971));
#27060=CARTESIAN_POINT('Ctrl Pts',(-14.2107516260897,0.273532057131348,
1.93798058286632));
#27061=CARTESIAN_POINT('Ctrl Pts',(-14.2477587917826,0.913314154071121,
1.84768001452293));
#27062=CARTESIAN_POINT('Ctrl Pts',(-14.2847659574756,1.50396826129945,1.40930651078944));
#27063=CARTESIAN_POINT('Ctrl Pts',(-14.3217731231685,1.77569634071135,0.823098916020689));
#27064=CARTESIAN_POINT('Ctrl Pts',(-14.3587802888615,2.04742442012326,0.236891321251938));
#27065=CARTESIAN_POINT('Ctrl Pts',(-14.3957874545544,2.00022647171874,-0.497150364552078));
#27066=CARTESIAN_POINT('Ctrl Pts',(-14.4327946202473,1.65566169603906,-1.04373070318105));
#27067=CARTESIAN_POINT('Ctrl Pts',(-14.4698017859403,1.31109692035938,-1.59031104181003));
#27068=CARTESIAN_POINT('Ctrl Pts',(-14.5068089516332,0.66916531740454,-1.94943003326396));
#27069=CARTESIAN_POINT('Ctrl Pts',(-14.5438161173262,0.0230868684858276,
-1.95705220165554));
#27070=CARTESIAN_POINT('Ctrl Pts',(-14.5808232830191,-0.622991580432885,
-1.96467437004712));
#27071=CARTESIAN_POINT('Ctrl Pts',(-14.617830448712,-1.27321687531547,-1.62079971537635));
#27072=CARTESIAN_POINT('Ctrl Pts',(-14.654837614405,-1.63057951982903,-1.08249839438246));
#27073=CARTESIAN_POINT('Ctrl Pts',(-14.6766018455619,-1.84074755232787,
-0.765918776278231));
#27074=CARTESIAN_POINT('Ctrl Pts',(-14.6983660767188,-1.94962268626342,
-0.38209247934674));
#27075=CARTESIAN_POINT('Ctrl Pts',(-14.7201303078758,-1.95121230271199,
0.000898656016518479));
#27076=CARTESIAN_POINT('Ctrl Pts',(-14.8218696921242,-1.95111217225575,
0.000805047651922751));
#27077=CARTESIAN_POINT('Ctrl Pts',(-14.800522469206,-1.94974347955955,-0.374899554732456));
#27078=CARTESIAN_POINT('Ctrl Pts',(-14.7791752462877,-1.8452747003299,-0.751314904469925));
#27079=CARTESIAN_POINT('Ctrl Pts',(-14.7578280233694,-1.64263463153156,
-1.06412750934765));
#27080=CARTESIAN_POINT('Ctrl Pts',(-14.7208208576765,-1.2913414150436,-1.60641387342718));
#27081=CARTESIAN_POINT('Ctrl Pts',(-14.6838136919835,-0.645013310489882,
-1.95755444740034));
#27082=CARTESIAN_POINT('Ctrl Pts',(-14.6468065262906,0.00111119976138999,
-1.95718427626721));
#27083=CARTESIAN_POINT('Ctrl Pts',(-14.6097993605976,0.647235710012662,
-1.95681410513408));
#27084=CARTESIAN_POINT('Ctrl Pts',(-14.5727921949047,1.29315662596149,-1.60493318889466));
#27085=CARTESIAN_POINT('Ctrl Pts',(-14.5357850292117,1.64383653694154,-1.06225813541516));
#27086=CARTESIAN_POINT('Ctrl Pts',(-14.4987778635188,1.9945164479216,-0.519583081935655));
#27087=CARTESIAN_POINT('Ctrl Pts',(-14.4617706978259,2.04995535393287,0.21388610878393));
#27088=CARTESIAN_POINT('Ctrl Pts',(-14.4247635321329,1.78482724106282,0.803108842016717));
#27089=CARTESIAN_POINT('Ctrl Pts',(-14.38775636644,1.51969912819276,1.39233157524951));
#27090=CARTESIAN_POINT('Ctrl Pts',(-14.350749200747,0.934003996441376,1.8373078509955));
#27091=CARTESIAN_POINT('Ctrl Pts',(-14.3137420350541,0.295276058031193,
1.93478632229321));
#27092=CARTESIAN_POINT('Ctrl Pts',(-14.2767348693612,-0.34345188037899,
2.03226479359092));
#27093=CARTESIAN_POINT('Ctrl Pts',(-14.2397277036682,-1.03521262544797,
1.78224546044036));
#27094=CARTESIAN_POINT('Ctrl Pts',(-14.2027205379753,-1.46402569115998,
1.29892954146499));
#27095=CARTESIAN_POINT('Ctrl Pts',(-14.1757702560249,-1.77630664563288,
0.946957158722955));
#27096=CARTESIAN_POINT('Ctrl Pts',(-14.1488199740746,-1.94913573752573,
0.471258095804866));
#27097=CARTESIAN_POINT('Ctrl Pts',(-14.1218696921242,-1.95325151398278,
-0.00174533096842624));
#27098=CARTESIAN_POINT('Origin',(-7.7,0.,0.));
#27099=CARTESIAN_POINT('',(-13.3201303078758,-1.95714464087111,0.00026399773373942));
#27100=CARTESIAN_POINT('',(-13.4218696921242,-1.95708965070517,0.000396557255078462));
#27101=CARTESIAN_POINT('',(-7.7,-1.954,-2.39295984553393E-16));
#27102=CARTESIAN_POINT('Ctrl Pts',(-13.3201303078758,-1.95714464087111,
0.00026399773373942));
#27103=CARTESIAN_POINT('Ctrl Pts',(-13.3209467550702,-1.95717172753317,
0.0145195559070077));
#27104=CARTESIAN_POINT('Ctrl Pts',(-13.3217632022646,-1.95702941419436,
0.0287745591326669));
#27105=CARTESIAN_POINT('Ctrl Pts',(-13.3225796494591,-1.95671604674699,
0.0430258010876729));
#27106=CARTESIAN_POINT('Ctrl Pts',(-13.359586815152,-1.94251201600704,0.688992957266154));
#27107=CARTESIAN_POINT('Ctrl Pts',(-13.396593980845,-1.57686979233981,1.32723241737986));
#27108=CARTESIAN_POINT('Ctrl Pts',(-13.4336011465379,-1.02680677935604,
1.66621029520631));
#27109=CARTESIAN_POINT('Ctrl Pts',(-13.4706083122308,-0.476743766372259,
2.00518817303275));
#27110=CARTESIAN_POINT('Ctrl Pts',(-13.5076154779238,0.257740035928053,
2.04490446857193));
#27111=CARTESIAN_POINT('Ctrl Pts',(-13.5446226436167,0.841148427119235,
1.76721765005178));
#27112=CARTESIAN_POINT('Ctrl Pts',(-13.5816298093097,1.42455681831042,1.48953083153163));
#27113=CARTESIAN_POINT('Ctrl Pts',(-13.6186369750026,1.85688979839247,0.894440898952159));
#27114=CARTESIAN_POINT('Ctrl Pts',(-13.6556441406956,1.94066707730226,0.253771957552514));
#27115=CARTESIAN_POINT('Ctrl Pts',(-13.6926513063885,2.02444435621205,-0.386896983847131));
#27116=CARTESIAN_POINT('Ctrl Pts',(-13.7296584720814,1.75966593394958,-1.07314493406695));
#27117=CARTESIAN_POINT('Ctrl Pts',(-13.7666656377744,1.26727683046446,-1.49150875303897));
#27118=CARTESIAN_POINT('Ctrl Pts',(-13.8036728034673,0.774887726979341,
-1.90987257201099));
#27119=CARTESIAN_POINT('Ctrl Pts',(-13.8406799691603,0.0548879422715688,
-2.06035225973521));
#27120=CARTESIAN_POINT('Ctrl Pts',(-13.8776871348532,-0.563842314011695,
-1.87421202025266));
#27121=CARTESIAN_POINT('Ctrl Pts',(-13.9146943005461,-1.18257257029496,
-1.68807178077012));
#27122=CARTESIAN_POINT('Ctrl Pts',(-13.9517014662391,-1.70003329815372,
-1.1653116140808));
#27123=CARTESIAN_POINT('Ctrl Pts',(-13.988708631932,-1.87985969326617,-0.544716886651509));
#27124=CARTESIAN_POINT('Ctrl Pts',(-13.9991825239133,-1.93075476189727,
-0.369074088357832));
#27125=CARTESIAN_POINT('Ctrl Pts',(-14.0096564158945,-1.9546045722002,-0.185594524925036));
#27126=CARTESIAN_POINT('Ctrl Pts',(-14.0201303078758,-1.9530433091271,-0.00171791376288949));
#27127=CARTESIAN_POINT('Ctrl Pts',(-14.1218696921242,-1.95325151398278,
-0.00174533096842624));
#27128=CARTESIAN_POINT('Ctrl Pts',(-14.1118128083816,-1.95478737492165,
-0.178253334917205));
#27129=CARTESIAN_POINT('Ctrl Pts',(-14.101755924639,-1.9328296346151,-0.354385967185775));
#27130=CARTESIAN_POINT('Ctrl Pts',(-14.0916990408964,-1.88585775871412,
-0.523573852172993));
#27131=CARTESIAN_POINT('Ctrl Pts',(-14.0546918752035,-1.7130113742012,-1.14614882203543));
#27132=CARTESIAN_POINT('Ctrl Pts',(-14.0176847095106,-1.20145321882029,
-1.67468625696012));
#27133=CARTESIAN_POINT('Ctrl Pts',(-13.9806775438176,-0.584852122809202,
-1.86776236812173));
#27134=CARTESIAN_POINT('Ctrl Pts',(-13.9436703781247,0.0317489732018875,
-2.06083847928334));
#27135=CARTESIAN_POINT('Ctrl Pts',(-13.9066632124317,0.753393009843159,
-1.91845326668187));
#27136=CARTESIAN_POINT('Ctrl Pts',(-13.8696560467388,1.25044882013409,-1.50564487944031));
#27137=CARTESIAN_POINT('Ctrl Pts',(-13.8326488810459,1.74750463042501,-1.09283649219875));
#27138=CARTESIAN_POINT('Ctrl Pts',(-13.7956417153529,2.0199722143656,-0.409604930317106));
#27139=CARTESIAN_POINT('Ctrl Pts',(-13.75863454966,1.94339425729846,0.231964346352179));
#27140=CARTESIAN_POINT('Ctrl Pts',(-13.721627383967,1.86681630023132,0.873533623021462));
#27141=CARTESIAN_POINT('Ctrl Pts',(-13.6846202182741,1.44119280215647,1.47344061447839));
#27142=CARTESIAN_POINT('Ctrl Pts',(-13.6476130525811,0.860939335837695,
1.75766096163323));
#27143=CARTESIAN_POINT('Ctrl Pts',(-13.6106058868882,0.280685869518923,
2.04188130878808));
#27144=CARTESIAN_POINT('Ctrl Pts',(-13.5735987211953,-0.454197565043769,
2.01041501164085));
#27145=CARTESIAN_POINT('Ctrl Pts',(-13.5365915555023,-1.00803223878929,
1.67763514366989));
#27146=CARTESIAN_POINT('Ctrl Pts',(-13.4995843898094,-1.56186691253481,
1.34485527569892));
#27147=CARTESIAN_POINT('Ctrl Pts',(-13.4625772241164,-1.93465282546315,
0.710761836904218));
#27148=CARTESIAN_POINT('Ctrl Pts',(-13.4255700584235,-1.95610948460737,
0.0649949216400037));
#27149=CARTESIAN_POINT('Ctrl Pts',(-13.4243366029904,-1.95682463888362,
0.0434713951763571));
#27150=CARTESIAN_POINT('Ctrl Pts',(-13.4231031475573,-1.9571495012145,0.0219349006384856));
#27151=CARTESIAN_POINT('Ctrl Pts',(-13.4218696921242,-1.95708965070517,
0.000396557255078462));
#27152=CARTESIAN_POINT('Origin',(-7.7,0.,0.));
#27153=CARTESIAN_POINT('',(-12.6201303078758,-1.95228596855585,0.00153407439264161));
#27154=CARTESIAN_POINT('',(-12.7218696921242,-1.95211097167562,0.00146895452558163));
#27155=CARTESIAN_POINT('',(-7.7,-1.954,-2.39295984553393E-16));
#27156=CARTESIAN_POINT('Ctrl Pts',(-12.6201303078758,-1.95228596855585,
0.00153407439264161));
#27157=CARTESIAN_POINT('Ctrl Pts',(-12.6322370942459,-1.95385293866565,
0.214285889020126));
#27158=CARTESIAN_POINT('Ctrl Pts',(-12.644343880616,-1.92179605864578,0.426578482544302));
#27159=CARTESIAN_POINT('Ctrl Pts',(-12.6564506669861,-1.85409897528216,
0.626822061414732));
#27160=CARTESIAN_POINT('Ctrl Pts',(-12.6934578326791,-1.64716733344281,
1.23891242756645));
#27161=CARTESIAN_POINT('Ctrl Pts',(-12.730464998372,-1.10722815379444,1.73842171037899));
#27162=CARTESIAN_POINT('Ctrl Pts',(-12.767472164065,-0.480913892112206,
1.89718495020391));
#27163=CARTESIAN_POINT('Ctrl Pts',(-12.8044793297579,0.145400369570025,
2.05594819002883));
#27164=CARTESIAN_POINT('Ctrl Pts',(-12.8414864954508,0.858089713286118,
1.87396538686614));
#27165=CARTESIAN_POINT('Ctrl Pts',(-12.8784936611438,1.331613171372,1.43436232121203));
#27166=CARTESIAN_POINT('Ctrl Pts',(-12.9155008268367,1.80513662945789,0.994759255557927));
#27167=CARTESIAN_POINT('Ctrl Pts',(-12.9525079925297,2.03949420191357,0.297535927412401));
#27168=CARTESIAN_POINT('Ctrl Pts',(-12.9895151582226,1.92763645460712,-0.338831234827492));
#27169=CARTESIAN_POINT('Ctrl Pts',(-13.0265223239155,1.81577870730067,-0.975198397067393));
#27170=CARTESIAN_POINT('Ctrl Pts',(-13.0635294896085,1.35770564023208,-1.55070939340166));
#27171=CARTESIAN_POINT('Ctrl Pts',(-13.1005366553014,0.762655052318492,
-1.80248333654236));
#27172=CARTESIAN_POINT('Ctrl Pts',(-13.1375438209944,0.167604464404906,
-2.05425727968306));
#27173=CARTESIAN_POINT('Ctrl Pts',(-13.1745509866873,-0.564423644353677,
-1.98229416963019));
#27174=CARTESIAN_POINT('Ctrl Pts',(-13.2115581523803,-1.09905477982664,
-1.61946518848213));
#27175=CARTESIAN_POINT('Ctrl Pts',(-13.2477488708788,-1.62189095390655,
-1.26464089232335));
#27176=CARTESIAN_POINT('Ctrl Pts',(-13.2839395893773,-1.95594396828844,
-0.631643241833467));
#27177=CARTESIAN_POINT('Ctrl Pts',(-13.3201303078758,-1.95714464087111,
0.00026399773373942));
#27178=CARTESIAN_POINT('Ctrl Pts',(-13.4218696921242,-1.95708965070517,
0.000396557255078462));
#27179=CARTESIAN_POINT('Ctrl Pts',(-13.3860959818644,-1.95535381597439,
-0.624276564294844));
#27180=CARTESIAN_POINT('Ctrl Pts',(-13.3503222716045,-1.63001111528494,
-1.25050486946977));
#27181=CARTESIAN_POINT('Ctrl Pts',(-13.3145485613447,-1.11717032068386,
-1.60702181624921));
#27182=CARTESIAN_POINT('Ctrl Pts',(-13.2775413956517,-0.58664709225607,
-1.97583124714049));
#27183=CARTESIAN_POINT('Ctrl Pts',(-13.2405342299588,0.1445267699596,-2.05600971718931));
#27184=CARTESIAN_POINT('Ctrl Pts',(-13.2035270642658,0.742366975175223,
-1.81093344118442));
#27185=CARTESIAN_POINT('Ctrl Pts',(-13.1665198985729,1.34020718039085,-1.56585716517953));
#27186=CARTESIAN_POINT('Ctrl Pts',(-13.12951273288,1.80471372860643,-0.995526143120937));
#27187=CARTESIAN_POINT('Ctrl Pts',(-13.092505567187,1.92371014573817,-0.36045516583733));
#27188=CARTESIAN_POINT('Ctrl Pts',(-13.0554984014941,2.04270656286991,0.274615811446275));
#27189=CARTESIAN_POINT('Ctrl Pts',(-13.0184912358011,1.8161928489178,0.974426743954891));
#27190=CARTESIAN_POINT('Ctrl Pts',(-12.9814840701082,1.34763553490042,1.41931924353683));
#27191=CARTESIAN_POINT('Ctrl Pts',(-12.9444769044152,0.87907822088303,1.86421174311878));
#27192=CARTESIAN_POINT('Ctrl Pts',(-12.9074697387223,0.168477306800354,
2.05418580977404));
#27193=CARTESIAN_POINT('Ctrl Pts',(-12.8704625730294,-0.459580189156903,
1.90246542710088));
#27194=CARTESIAN_POINT('Ctrl Pts',(-12.8334554073364,-1.08763768511415,
1.75074504442773));
#27195=CARTESIAN_POINT('Ctrl Pts',(-12.7964482416435,-1.63315176294599,
1.25733021242617));
#27196=CARTESIAN_POINT('Ctrl Pts',(-12.7594410759505,-1.84694347466266,
0.647602078798446));
#27197=CARTESIAN_POINT('Ctrl Pts',(-12.7469172813418,-1.91929388130583,
0.441260691400759));
#27198=CARTESIAN_POINT('Ctrl Pts',(-12.734393486733,-1.95365379066715,0.221598525482708));
#27199=CARTESIAN_POINT('Ctrl Pts',(-12.7218696921242,-1.95211097167562,
0.00146895452558163));
#27200=CARTESIAN_POINT('Origin',(-7.7,0.,0.));
#27201=CARTESIAN_POINT('',(-11.9201303078758,-1.95169843653047,-0.00126854855504954));
#27202=CARTESIAN_POINT('',(-12.0218696921242,-1.9518489925303,-0.00135048404527946));
#27203=CARTESIAN_POINT('',(-7.7,-1.954,-2.39295984553393E-16));
#27204=CARTESIAN_POINT('Ctrl Pts',(-11.9201303078758,-1.95169843653047,
-0.00126854855504954));
#27205=CARTESIAN_POINT('Ctrl Pts',(-11.9435274334216,-1.94924301286788,
0.410199212160575));
#27206=CARTESIAN_POINT('Ctrl Pts',(-11.9669245589674,-1.82209832848306,
0.823054588837745));
#27207=CARTESIAN_POINT('Ctrl Pts',(-11.9903216845132,-1.58142069241171,
1.15312510181565));
#27208=CARTESIAN_POINT('Ctrl Pts',(-12.0273288502061,-1.20074157269491,
1.67519667595913));
#27209=CARTESIAN_POINT('Ctrl Pts',(-12.0643360158991,-0.53602960573929,
1.99015991551352));
#27210=CARTESIAN_POINT('Ctrl Pts',(-12.101343181592,0.109089261378069,1.95414647349669));
#27211=CARTESIAN_POINT('Ctrl Pts',(-12.1383503472849,0.75420812849542,1.91813303147986));
#27212=CARTESIAN_POINT('Ctrl Pts',(-12.1753575129779,1.3797338957745,1.53114290789182));
#27213=CARTESIAN_POINT('Ctrl Pts',(-12.2123646786708,1.69994001855784,0.969944761380266));
#27214=CARTESIAN_POINT('Ctrl Pts',(-12.2493718443638,2.02014614134118,0.408746614868707));
#27215=CARTESIAN_POINT('Ctrl Pts',(-12.2863790100567,2.03503261962877,-0.326659554566366));
#27216=CARTESIAN_POINT('Ctrl Pts',(-12.3233861757497,1.73779963441016,-0.900356228093971));
#27217=CARTESIAN_POINT('Ctrl Pts',(-12.3603933414426,1.44056664919155,-1.47405290162158));
#27218=CARTESIAN_POINT('Ctrl Pts',(-12.3974005071355,0.831214200466734,
-1.88604007924171));
#27219=CARTESIAN_POINT('Ctrl Pts',(-12.4344076728285,0.18808121328365,-1.94813099252794));
#27220=CARTESIAN_POINT('Ctrl Pts',(-12.4714148385214,-0.455051773899431,
-2.01022190581416));
#27221=CARTESIAN_POINT('Ctrl Pts',(-12.5084220042144,-1.13196529954078,
-1.72241655476647));
#27222=CARTESIAN_POINT('Ctrl Pts',(-12.5454291699073,-1.5334600103463,-1.21617815449718));
#27223=CARTESIAN_POINT('Ctrl Pts',(-12.5703295492301,-1.80360689698215,
-0.875554171048228));
#27224=CARTESIAN_POINT('Ctrl Pts',(-12.5952299285529,-1.94906313559845,
-0.43603876483078));
#27225=CARTESIAN_POINT('Ctrl Pts',(-12.6201303078758,-1.95228596855585,
0.00153407439264161));
#27226=CARTESIAN_POINT('Ctrl Pts',(-12.7218696921242,-1.95211097167562,
0.00146895452558163));
#27227=CARTESIAN_POINT('Ctrl Pts',(-12.6973863210401,-1.94909484029808,
-0.428872977828815));
#27228=CARTESIAN_POINT('Ctrl Pts',(-12.6729029499559,-1.80886483995233,
-0.86100124945961));
#27229=CARTESIAN_POINT('Ctrl Pts',(-12.6484195788717,-1.54701966560394,
-1.19888231497363));
#27230=CARTESIAN_POINT('Ctrl Pts',(-12.6114124131788,-1.15123479922702,
-1.7095971398641));
#27231=CARTESIAN_POINT('Ctrl Pts',(-12.5744052474858,-0.477595720871672,
-2.00498535439116));
#27232=CARTESIAN_POINT('Ctrl Pts',(-12.5373980817929,0.166193912405789,
-1.95012005646431));
#27233=CARTESIAN_POINT('Ctrl Pts',(-12.5003909160999,0.809983545683245,
-1.89525475853747));
#27234=CARTESIAN_POINT('Ctrl Pts',(-12.463383750407,1.42392373388281,-1.49013594815671));
#27235=CARTESIAN_POINT('Ctrl Pts',(-12.4263765847141,1.7275799724757,-0.919813073269506));
#27236=CARTESIAN_POINT('Ctrl Pts',(-12.3893694190211,2.0312362110686,-0.349490198382288));
#27237=CARTESIAN_POINT('Ctrl Pts',(-12.3523622533282,2.02460850005481,0.386036741011393));
#27238=CARTESIAN_POINT('Ctrl Pts',(-12.3153550876352,1.71072423346732,0.950795061026896));
#27239=CARTESIAN_POINT('Ctrl Pts',(-12.2783479219423,1.39683996687984,1.51555338104239));
#27240=CARTESIAN_POINT('Ctrl Pts',(-12.2413407562494,0.775699144718677,
1.90954308167971));
#27241=CARTESIAN_POINT('Ctrl Pts',(-12.2043335905564,0.131025364222244,
1.95279824994973));
#27242=CARTESIAN_POINT('Ctrl Pts',(-12.1673264248635,-0.513648416274196,
1.99605341821975));
#27243=CARTESIAN_POINT('Ctrl Pts',(-12.1303192591705,-1.1818551551059,1.68857405412246));
#27244=CARTESIAN_POINT('Ctrl Pts',(-12.0933120934776,-1.56837256952603,
1.17081003336157));
#27245=CARTESIAN_POINT('Ctrl Pts',(-12.0694979596931,-1.81709676238617,
0.837628568953355));
#27246=CARTESIAN_POINT('Ctrl Pts',(-12.0456838259087,-1.94917536710479,
0.417369692204787));
#27247=CARTESIAN_POINT('Ctrl Pts',(-12.0218696921242,-1.9518489925303,-0.00135048404527946));
#27248=CARTESIAN_POINT('Origin',(-7.7,0.,0.));
#27249=CARTESIAN_POINT('',(-11.2201303078758,-1.95685610654859,-0.000727346471807722));
#27250=CARTESIAN_POINT('',(-11.3218696921242,-1.9569602541593,-0.00060337692984129));
#27251=CARTESIAN_POINT('',(-7.7,-1.954,-2.39295984553393E-16));
#27252=CARTESIAN_POINT('Ctrl Pts',(-11.2201303078758,-1.95685610654859,
-0.000727346471807722));
#27253=CARTESIAN_POINT('Ctrl Pts',(-11.2548177725973,-1.95395813312852,
0.60517099785977));
#27254=CARTESIAN_POINT('Ctrl Pts',(-11.2895052373187,-1.65063759095734,
1.21357459286489));
#27255=CARTESIAN_POINT('Ctrl Pts',(-11.3241927020402,-1.16369172863257,
1.57366148441711));
#27256=CARTESIAN_POINT('Ctrl Pts',(-11.3611998677332,-0.644181687894853,
1.95782894567513));
#27257=CARTESIAN_POINT('Ctrl Pts',(-11.3982070334261,0.0843345183607735,
2.0593571609984));
#27258=CARTESIAN_POINT('Ctrl Pts',(-11.435214199119,0.689086556393739,1.83187025321751));
#27259=CARTESIAN_POINT('Ctrl Pts',(-11.472221364812,1.29383859442671,1.60438334543661));
#27260=CARTESIAN_POINT('Ctrl Pts',(-11.5092285305049,1.77482646423702,1.04788131455156));
#27261=CARTESIAN_POINT('Ctrl Pts',(-11.5462356961979,1.91234538425969,0.416562165980472));
#27262=CARTESIAN_POINT('Ctrl Pts',(-11.5832428618908,2.04986430428237,-0.214756982590612));
#27263=CARTESIAN_POINT('Ctrl Pts',(-11.6202500275838,1.84391427451741,-0.92089324884772));
#27264=CARTESIAN_POINT('Ctrl Pts',(-11.6572571932767,1.38856878234954,-1.37929896813924));
#27265=CARTESIAN_POINT('Ctrl Pts',(-11.6942643589696,0.933223290181664,
-1.83770468743075));
#27266=CARTESIAN_POINT('Ctrl Pts',(-11.7312715246626,0.228482335610874,
-2.04837985975668));
#27267=CARTESIAN_POINT('Ctrl Pts',(-11.7682786903555,-0.403743764695274,
-1.91509265553802));
#27268=CARTESIAN_POINT('Ctrl Pts',(-11.8052858560485,-1.03596986500142,
-1.78180545131937));
#27269=CARTESIAN_POINT('Ctrl Pts',(-11.8422930217414,-1.59568111104292,
-1.30455587055615));
#27270=CARTESIAN_POINT('Ctrl Pts',(-11.8793001874343,-1.82721359782469,
-0.701341125808267));
#27271=CARTESIAN_POINT('Ctrl Pts',(-11.8929102275815,-1.91236376756786,
-0.479498227557532));
#27272=CARTESIAN_POINT('Ctrl Pts',(-11.9065202677286,-1.9531267493615,-0.240618152917035));
#27273=CARTESIAN_POINT('Ctrl Pts',(-11.9201303078758,-1.95169843653047,
-0.00126854855504954));
#27274=CARTESIAN_POINT('Ctrl Pts',(-12.0218696921242,-1.9518489925303,-0.00135048404527946));
#27275=CARTESIAN_POINT('Ctrl Pts',(-12.0086766602157,-1.95333018121721,
-0.233321493194773));
#27276=CARTESIAN_POINT('Ctrl Pts',(-11.9954836283072,-1.9150949004906,-0.464820250413784));
#27277=CARTESIAN_POINT('Ctrl Pts',(-11.9822905963988,-1.8349736515092,-0.680779222162789));
#27278=CARTESIAN_POINT('Ctrl Pts',(-11.9452834307058,-1.6102292290637,-1.28655577950177));
#27279=CARTESIAN_POINT('Ctrl Pts',(-11.9082762650129,-1.05591229416418,
-1.77006021675525));
#27280=CARTESIAN_POINT('Ctrl Pts',(-11.8712690993199,-0.425222747979457,
-1.91043823916569));
#27281=CARTESIAN_POINT('Ctrl Pts',(-11.834261933627,0.205466798205275,-2.05081626157613));
#27282=CARTESIAN_POINT('Ctrl Pts',(-11.797254767934,0.912528955675209,-1.84806786914353));
#27283=CARTESIAN_POINT('Ctrl Pts',(-11.7602476022411,1.37299313284074,-1.39480411106204));
#27284=CARTESIAN_POINT('Ctrl Pts',(-11.7232404365482,1.83345731000627,-0.941540352980555));
#27285=CARTESIAN_POINT('Ctrl Pts',(-11.6862332708552,2.04732350686741,-0.237761229250197));
#27286=CARTESIAN_POINT('Ctrl Pts',(-11.6492261051623,1.91690230334813,0.395062286838669));
#27287=CARTESIAN_POINT('Ctrl Pts',(-11.6122189394693,1.78648109982885,1.02788580292753));
#27288=CARTESIAN_POINT('Ctrl Pts',(-11.5752117737764,1.31177249592916,1.5897537113749));
#27289=CARTESIAN_POINT('Ctrl Pts',(-11.5382046080835,0.709613041327233,
1.82401699077679));
#27290=CARTESIAN_POINT('Ctrl Pts',(-11.5011974423905,0.107453586725291,
2.05828027017869));
#27291=CARTESIAN_POINT('Ctrl Pts',(-11.4641902766976,-0.622156718578892,
1.96493892053509));
#27292=CARTESIAN_POINT('Ctrl Pts',(-11.4271831110046,-1.14594778023205,
1.58662923710771));
#27293=CARTESIAN_POINT('Ctrl Pts',(-11.3920786380445,-1.64280855884786,
1.2277700323088));
#27294=CARTESIAN_POINT('Ctrl Pts',(-11.3569741650844,-1.95447007917529,
0.612492024699057));
#27295=CARTESIAN_POINT('Ctrl Pts',(-11.3218696921242,-1.9569602541593,-0.00060337692984129));
#27296=CARTESIAN_POINT('Origin',(-7.7,0.,0.));
#27297=CARTESIAN_POINT('',(-10.5201303078758,-1.95381282533802,0.00177708690787488));
#27298=CARTESIAN_POINT('',(-10.6218696921242,-1.95359472300144,0.00177181249679811));
#27299=CARTESIAN_POINT('',(-7.7,-1.954,-2.39295984553393E-16));
#27300=CARTESIAN_POINT('Ctrl Pts',(-10.5201303078758,-1.95381282533802,
0.00177708690787488));
#27301=CARTESIAN_POINT('Ctrl Pts',(-10.52910094608,-1.95524187263722,0.159105178249771));
#27302=CARTESIAN_POINT('Ctrl Pts',(-10.5380715842842,-1.93783046980655,
0.316120934930408));
#27303=CARTESIAN_POINT('Ctrl Pts',(-10.5470422224884,-1.90036359504,0.468195593179135));
#27304=CARTESIAN_POINT('Ctrl Pts',(-10.5840493881814,-1.74579902439106,
1.09555921518542));
#27305=CARTESIAN_POINT('Ctrl Pts',(-10.6210565538743,-1.24991750672224,
1.63883203957322));
#27306=CARTESIAN_POINT('Ctrl Pts',(-10.6580637195673,-0.639226917511803,
1.84985887428044));
#27307=CARTESIAN_POINT('Ctrl Pts',(-10.6950708852602,-0.0285363283013634,
2.06088570898765));
#27308=CARTESIAN_POINT('Ctrl Pts',(-10.7320780509531,0.696963332450705,
1.93966655401429));
#27309=CARTESIAN_POINT('Ctrl Pts',(-10.7690852166461,1.20587962328041,1.54157167883392));
#27310=CARTESIAN_POINT('Ctrl Pts',(-10.806092382339,1.71479591411012,1.14347680365354));
#27311=CARTESIAN_POINT('Ctrl Pts',(-10.843099548032,2.00712883501746,0.468506208266162));
#27312=CARTESIAN_POINT('Ctrl Pts',(-10.8801067137249,1.94934707562338,-0.175028242247616));
#27313=CARTESIAN_POINT('Ctrl Pts',(-10.9171138794179,1.89156531622931,-0.81856269276138));
#27314=CARTESIAN_POINT('Ctrl Pts',(-10.9541210451108,1.48366887653383,-1.43066099840154));
#27315=CARTESIAN_POINT('Ctrl Pts',(-10.9911282108037,0.911975964976942,
-1.73172998649619));
#27316=CARTESIAN_POINT('Ctrl Pts',(-11.0281353764967,0.340283053420042,
-2.03279897459085));
#27317=CARTESIAN_POINT('Ctrl Pts',(-11.0651425421896,-0.395206329998278,
-2.02283864513999));
#27318=CARTESIAN_POINT('Ctrl Pts',(-11.1021497078826,-0.958536656106322,
-1.70639865967078));
#27319=CARTESIAN_POINT('Ctrl Pts',(-11.1391568735755,-1.52186698221436,
-1.38995867420158));
#27320=CARTESIAN_POINT('Ctrl Pts',(-11.1761640392684,-1.91303825101214,
-0.767039032714035));
#27321=CARTESIAN_POINT('Ctrl Pts',(-11.2131712049614,-1.95337194780112,
-0.122175858373872));
#27322=CARTESIAN_POINT('Ctrl Pts',(-11.2154909059329,-1.95590016399579,
-0.0817542345081737));
#27323=CARTESIAN_POINT('Ctrl Pts',(-11.2178106069043,-1.95704990658016,
-0.0412463924510177));
#27324=CARTESIAN_POINT('Ctrl Pts',(-11.2201303078758,-1.95685610654859,
-0.000727346471807722));
#27325=CARTESIAN_POINT('Ctrl Pts',(-11.3218696921242,-1.9569602541593,-0.00060337692984129));
#27326=CARTESIAN_POINT('Ctrl Pts',(-11.3199669993914,-1.95709522379268,
-0.0338336768556207));
#27327=CARTESIAN_POINT('Ctrl Pts',(-11.3180643066586,-1.9563219303891,-0.0670575648665623));
#27328=CARTESIAN_POINT('Ctrl Pts',(-11.3161616139258,-1.95462063415894,
-0.100233864456555));
#27329=CARTESIAN_POINT('Ctrl Pts',(-11.2791544482329,-1.92153060843055,
-0.745509265382321));
#27330=CARTESIAN_POINT('Ctrl Pts',(-11.2421472825399,-1.53737873897162,
-1.3727820500227));
#27331=CARTESIAN_POINT('Ctrl Pts',(-11.205140116847,-0.977637231766315,
-1.69552767424427));
#27332=CARTESIAN_POINT('Ctrl Pts',(-11.168132951154,-0.41789572456102,-2.01827329846583));
#27333=CARTESIAN_POINT('Ctrl Pts',(-11.1311257854611,0.31743542039065,-2.0364917622686));
#27334=CARTESIAN_POINT('Ctrl Pts',(-11.0941186197681,0.892472953801631,
-1.7418612682405));
#27335=CARTESIAN_POINT('Ctrl Pts',(-11.0571114540752,1.46751048721262,-1.44723077421241));
#27336=CARTESIAN_POINT('Ctrl Pts',(-11.0201042883823,1.88225440908292,-0.839751322353458));
#27337=CARTESIAN_POINT('Ctrl Pts',(-10.9830971226893,1.94725873027388,-0.196906293540815));
#27338=CARTESIAN_POINT('Ctrl Pts',(-10.9460899569964,2.01226305146485,0.445938735271831));
#27339=CARTESIAN_POINT('Ctrl Pts',(-10.9090827913034,1.72752777197646,1.12414934103816));
#27340=CARTESIAN_POINT('Ctrl Pts',(-10.8720756256105,1.2231137650871,1.52793369251362));
#27341=CARTESIAN_POINT('Ctrl Pts',(-10.8350684599176,0.718699758197757,
1.93171804398907));
#27342=CARTESIAN_POINT('Ctrl Pts',(-10.7980612942246,-0.0053929760925614,
2.06107614117366));
#27343=CARTESIAN_POINT('Ctrl Pts',(-10.7610541285317,-0.618414649680478,
1.85692002308242));
#27344=CARTESIAN_POINT('Ctrl Pts',(-10.7240469628387,-1.23143632326841,
1.65276390499117));
#27345=CARTESIAN_POINT('Ctrl Pts',(-10.6870397971458,-1.73338693615394,
1.11509357162407));
#27346=CARTESIAN_POINT('Ctrl Pts',(-10.6500326314528,-1.89498638236701,
0.48950511918408));
#27347=CARTESIAN_POINT('Ctrl Pts',(-10.64064498501,-1.9359794829735,0.330811441884507));
#27348=CARTESIAN_POINT('Ctrl Pts',(-10.6312573385671,-1.95507132644295,
0.166460321563234));
#27349=CARTESIAN_POINT('Ctrl Pts',(-10.6218696921242,-1.95359472300144,
0.00177181249679811));
#27350=CARTESIAN_POINT('Origin',(-7.7,0.,0.));
#27351=CARTESIAN_POINT('',(-9.82013030787577,-1.95092775659677,-0.000499046442109796));
#27352=CARTESIAN_POINT('',(-9.92186969212424,-1.950990226885,-0.00061315819592252));
#27353=CARTESIAN_POINT('',(-7.7,-1.954,-2.39295984553393E-16));
#27354=CARTESIAN_POINT('Ctrl Pts',(-9.82013030787577,-1.95092775659677,
-0.000499046442109796));
#27355=CARTESIAN_POINT('Ctrl Pts',(-9.84039128525567,-1.95011071406785,
0.356168159601569));
#27356=CARTESIAN_POINT('Ctrl Pts',(-9.86065226263557,-1.85661555206154,
0.713234132722242));
#27357=CARTESIAN_POINT('Ctrl Pts',(-9.88091324001548,-1.67305055867318,
1.01562332335817));
#27358=CARTESIAN_POINT('Ctrl Pts',(-9.91792040570842,-1.33776465422886,
1.56794450075198));
#27359=CARTESIAN_POINT('Ctrl Pts',(-9.95492757140137,-0.701988617061191,
1.93785350557233));
#27360=CARTESIAN_POINT('Ctrl Pts',(-9.99193473709431,-0.0561310918315319,
1.95638396214944));
#27361=CARTESIAN_POINT('Ctrl Pts',(-10.0289419027873,0.589726433398127,
1.97491441872654));
#27362=CARTESIAN_POINT('Ctrl Pts',(-10.0659490684802,1.24566544668979,1.64206632706039));
#27363=CARTESIAN_POINT('Ctrl Pts',(-10.1029562341731,1.61206729509896,1.10987744499024));
#27364=CARTESIAN_POINT('Ctrl Pts',(-10.1399633998661,1.97846914350813,0.577688562920078));
#27365=CARTESIAN_POINT('Ctrl Pts',(-10.176970565559,2.05533382703483,-0.15384110955408));
#27366=CARTESIAN_POINT('Ctrl Pts',(-10.213977731252,1.80755123258835,-0.750564752965431));
#27367=CARTESIAN_POINT('Ctrl Pts',(-10.2509848969449,1.55976863814187,-1.34728839637677));
#27368=CARTESIAN_POINT('Ctrl Pts',(-10.2879920626378,0.987338765722227,
-1.8092060107253));
#27369=CARTESIAN_POINT('Ctrl Pts',(-10.3249992283308,0.351735111804125,
-1.92532369173338));
#27370=CARTESIAN_POINT('Ctrl Pts',(-10.3620063940237,-0.283868542113976,
-2.04144137274146));
#27371=CARTESIAN_POINT('Ctrl Pts',(-10.3990135597167,-0.982645977530532,
-1.81175912040909));
#27372=CARTESIAN_POINT('Ctrl Pts',(-10.4360207254096,-1.42541088342427,
-1.34119078443052));
#27373=CARTESIAN_POINT('Ctrl Pts',(-10.4640572528983,-1.76084836486043,
-0.984689500423752));
#27374=CARTESIAN_POINT('Ctrl Pts',(-10.492093780387,-1.94934652952108,-0.489930777932722));
#27375=CARTESIAN_POINT('Ctrl Pts',(-10.5201303078758,-1.95381282533802,
0.00177708690787488));
#27376=CARTESIAN_POINT('Ctrl Pts',(-10.6218696921242,-1.95359472300144,
0.00177181249679811));
#27377=CARTESIAN_POINT('Ctrl Pts',(-10.5942501728742,-1.94925038840961,
-0.48276043678513));
#27378=CARTESIAN_POINT('Ctrl Pts',(-10.5666306536241,-1.76686494916673,
-0.970213133349514));
#27379=CARTESIAN_POINT('Ctrl Pts',(-10.539011134374,-1.4403811131439,-1.3251003358094));
#27380=CARTESIAN_POINT('Ctrl Pts',(-10.5020039686811,-1.0029281181671,-1.80061076685003));
#27381=CARTESIAN_POINT('Ctrl Pts',(-10.4649968029881,-0.306773848672879,
-2.03812505741843));
#27382=CARTESIAN_POINT('Ctrl Pts',(-10.4279896372952,0.330093589370354,
-1.92915185335951));
#27383=CARTESIAN_POINT('Ctrl Pts',(-10.3909824716023,0.966961027413597,
-1.82017864930059));
#27384=CARTESIAN_POINT('Ctrl Pts',(-10.3539753059093,1.54454163400586,-1.36471795061433));
#27385=CARTESIAN_POINT('Ctrl Pts',(-10.3169681402164,1.79900916950086,-0.770814283154929));
#27386=CARTESIAN_POINT('Ctrl Pts',(-10.2799609745234,2.05347670499587,-0.176910615695531));
#27387=CARTESIAN_POINT('Ctrl Pts',(-10.2429538088305,1.98483116939363,0.555436020537005));
#27388=CARTESIAN_POINT('Ctrl Pts',(-10.2059466431375,1.62442834805074,1.09170563482698));
#27389=CARTESIAN_POINT('Ctrl Pts',(-10.1689394774446,1.26402552670786,1.62797524911695));
#27390=CARTESIAN_POINT('Ctrl Pts',(-10.1319323117517,0.611865419624326,
1.96816784146434));
#27391=CARTESIAN_POINT('Ctrl Pts',(-10.0949251460587,-0.0341594422952981,
1.95689084610407));
#27392=CARTESIAN_POINT('Ctrl Pts',(-10.0579179803658,-0.680184304214917,
1.9456138507438));
#27393=CARTESIAN_POINT('Ctrl Pts',(-10.0209108146728,-1.32007392097063,
1.58286726767587));
#27394=CARTESIAN_POINT('Ctrl Pts',(-9.98390364897989,-1.66154065435141,
1.03434583433266));
#27395=CARTESIAN_POINT('Ctrl Pts',(-9.96322566336134,-1.85233733034239,
0.727856047888396));
#27396=CARTESIAN_POINT('Ctrl Pts',(-9.94254767774279,-1.9499638271078,0.363365762621769));
#27397=CARTESIAN_POINT('Ctrl Pts',(-9.92186969212424,-1.950990226885,-0.00061315819592252));
#27398=CARTESIAN_POINT('Origin',(-7.7,0.,0.));
#27399=CARTESIAN_POINT('',(-9.12013030787577,-1.95563441709699,-0.00147295684208459));
#27400=CARTESIAN_POINT('',(-9.22186969212424,-1.95583091145133,-0.00139679566445557));
#27401=CARTESIAN_POINT('',(-7.7,-1.954,-2.39295984553393E-16));
#27402=CARTESIAN_POINT('Ctrl Pts',(-9.12013030787577,-1.95563441709699,
-0.00147295684208459));
#27403=CARTESIAN_POINT('Ctrl Pts',(-9.15168162443136,-1.95100144064053,
0.550550385164461));
#27404=CARTESIAN_POINT('Ctrl Pts',(-9.18323294098694,-1.70599712346534,
1.10617250200022));
#27405=CARTESIAN_POINT('Ctrl Pts',(-9.21478425754253,-1.29228238927443,
1.46989630015075));
#27406=CARTESIAN_POINT('Ctrl Pts',(-9.25179142323547,-0.807028162534314,
1.89651516535433));
#27407=CARTESIAN_POINT('Ctrl Pts',(-9.28879858892841,-0.0896720996266766,
2.05913164758619));
#27408=CARTESIAN_POINT('Ctrl Pts',(-9.32580575462135,0.53211317608774,1.88346608003955));
#27409=CARTESIAN_POINT('Ctrl Pts',(-9.3628129203143,1.15389845180216,1.70780051249291));
#27410=CARTESIAN_POINT('Ctrl Pts',(-9.39982008600724,1.68011294032337,1.19385289516776));
#27411=CARTESIAN_POINT('Ctrl Pts',(-9.43682725170018,1.87039332583119,0.5763833043313));
#27412=CARTESIAN_POINT('Ctrl Pts',(-9.47383441739312,2.06067371133901,-0.0410862865051484));
#27413=CARTESIAN_POINT('Ctrl Pts',(-9.51084158308607,1.91501999383345,-0.762077850852902));
#27414=CARTESIAN_POINT('Ctrl Pts',(-9.54784874877901,1.49996361869444,-1.25725814748555));
#27415=CARTESIAN_POINT('Ctrl Pts',(-9.58485591447195,1.08490724355543,-1.7524384441182));
#27416=CARTESIAN_POINT('Ctrl Pts',(-9.62186308016489,0.400448210782955,
-2.02180747303574));
#27417=CARTESIAN_POINT('Ctrl Pts',(-9.65887024585783,-0.240767503031595,
-1.94232332949735));
#27418=CARTESIAN_POINT('Ctrl Pts',(-9.69587741155078,-0.881983216846153,
-1.86283918595894));
#27419=CARTESIAN_POINT('Ctrl Pts',(-9.73288457724372,-1.47995561170279,
-1.43450186996459));
#27420=CARTESIAN_POINT('Ctrl Pts',(-9.76989174293666,-1.76154392327062,
-0.852966536983759));
#27421=CARTESIAN_POINT('Ctrl Pts',(-9.7866379312497,-1.88896602663815,-0.589814792870613));
#27422=CARTESIAN_POINT('Ctrl Pts',(-9.80338411956273,-1.95160306202713,
-0.295293126979237));
#27423=CARTESIAN_POINT('Ctrl Pts',(-9.82013030787577,-1.95092775659677,
-0.000499046442109796));
#27424=CARTESIAN_POINT('Ctrl Pts',(-9.92186969212424,-1.950990226885,-0.00061315819592252));
#27425=CARTESIAN_POINT('Ctrl Pts',(-9.90554051204985,-1.95180076361229,
-0.288043348493711));
#27426=CARTESIAN_POINT('Ctrl Pts',(-9.88921133197546,-1.8923706209308,-0.57515464737431));
#27427=CARTESIAN_POINT('Ctrl Pts',(-9.87288215190107,-1.77101071131092,
-0.833132469350365));
#27428=CARTESIAN_POINT('Ctrl Pts',(-9.83587498620812,-1.49597018488382,
-1.4177930560717));
#27429=CARTESIAN_POINT('Ctrl Pts',(-9.79886782051518,-0.902845282023798,
-1.85281794589588));
#27430=CARTESIAN_POINT('Ctrl Pts',(-9.76186065482224,-0.262562538310644,
-1.93949724530346));
#27431=CARTESIAN_POINT('Ctrl Pts',(-9.7248534891293,0.377720205402501,-2.02617654471103));
#27432=CARTESIAN_POINT('Ctrl Pts',(-9.68784632343636,1.06516078996877,-1.76451025370202));
#27433=CARTESIAN_POINT('Ctrl Pts',(-9.65083915774341,1.48575133088456,-1.27402183412946));
#27434=CARTESIAN_POINT('Ctrl Pts',(-9.61383199205047,1.90634187180036,-0.783533414556894));
#27435=CARTESIAN_POINT('Ctrl Pts',(-9.57682482635753,2.06008236906566,-0.0642228664207834));
#27436=CARTESIAN_POINT('Ctrl Pts',(-9.53981766066459,1.87674751246072,0.555344420640338));
#27437=CARTESIAN_POINT('Ctrl Pts',(-9.50281049497165,1.69341265585578,1.17491170770145));
#27438=CARTESIAN_POINT('Ctrl Pts',(-9.4658033292787,1.17300244538061,1.69473573368758));
#27439=CARTESIAN_POINT('Ctrl Pts',(-9.42879616358576,0.553228929078587,
1.87737220686107));
#27440=CARTESIAN_POINT('Ctrl Pts',(-9.39178899789282,-0.0665445872234321,
2.06000868003456));
#27441=CARTESIAN_POINT('Ctrl Pts',(-9.35478183219989,-0.785681409352301,
1.90545760039541));
#27442=CARTESIAN_POINT('Ctrl Pts',(-9.31777466650694,-1.27569550192533,
1.48431453453482));
#27443=CARTESIAN_POINT('Ctrl Pts',(-9.28580634171271,-1.6989900010259,1.12051368509993));
#27444=CARTESIAN_POINT('Ctrl Pts',(-9.25383801691847,-1.95130805500872,
0.557776003036592));
#27445=CARTESIAN_POINT('Ctrl Pts',(-9.22186969212424,-1.95583091145133,
-0.00139679566445557));
#27446=CARTESIAN_POINT('Origin',(-7.7,0.,0.));
#27447=CARTESIAN_POINT('',(-8.42013030787577,-1.95544987894172,0.00153511913569427));
#27448=CARTESIAN_POINT('',(-8.52186969212424,-1.95524099021,0.00159565242000603));
#27449=CARTESIAN_POINT('',(-7.7,-1.954,-2.39295984553393E-16));
#27450=CARTESIAN_POINT('Ctrl Pts',(-8.42013030787577,-1.95544987894172,
0.00153511913569427));
#27451=CARTESIAN_POINT('Ctrl Pts',(-8.4259647979141,-1.95633055877726,0.103640688502044));
#27452=CARTESIAN_POINT('Ctrl Pts',(-8.43179928795242,-1.94902185525376,
0.205619918324635));
#27453=CARTESIAN_POINT('Ctrl Pts',(-8.43763377799075,-1.93308324972855,
0.306232030402798));
#27454=CARTESIAN_POINT('Ctrl Pts',(-8.47464094368369,-1.83198741929417,
0.944397333271522));
#27455=CARTESIAN_POINT('Ctrl Pts',(-8.51164810937664,-1.38369799135314,
1.5275614869025));
#27456=CARTESIAN_POINT('Ctrl Pts',(-8.54865527506958,-0.792983811495096,
1.78934780898864));
#27457=CARTESIAN_POINT('Ctrl Pts',(-8.58566244076252,-0.202269631637063,
2.05113413107477));
#27458=CARTESIAN_POINT('Ctrl Pts',(-8.62266960645546,0.530869300137978,
1.99154262161609));
#27459=CARTESIAN_POINT('Ctrl Pts',(-8.6596767721484,1.07155108976907,1.63779338405076));
#27460=CARTESIAN_POINT('Ctrl Pts',(-8.69668393784134,1.61223287940017,1.28404414648543));
#27461=CARTESIAN_POINT('Ctrl Pts',(-8.73369110353428,1.96045752688732,0.636137180813462));
#27462=CARTESIAN_POINT('Ctrl Pts',(-8.77069826922723,1.95716359863995,-0.00997772441117081));
#27463=CARTESIAN_POINT('Ctrl Pts',(-8.80770543492017,1.95386967039258,-0.656092629635813));
#27464=CARTESIAN_POINT('Ctrl Pts',(-8.84471260061312,1.59905716641068,-1.30041547441312));
#27465=CARTESIAN_POINT('Ctrl Pts',(-8.88171976630606,1.05479670962828,-1.64863361854084));
#27466=CARTESIAN_POINT('Ctrl Pts',(-8.918726931999,0.510536252845885,-1.99685176266856));
#27467=CARTESIAN_POINT('Ctrl Pts',(-8.95573409769193,-0.22317215673701,
-2.0489652061467));
#27468=CARTESIAN_POINT('Ctrl Pts',(-8.99274126338488,-0.811186500001768,
-1.7811696631822));
#27469=CARTESIAN_POINT('Ctrl Pts',(-9.02974842907782,-1.39920084326652,
-1.5133741202177));
#27470=CARTESIAN_POINT('Ctrl Pts',(-9.06675559477076,-1.84152112021314,
-0.925669590810556));
#27471=CARTESIAN_POINT('Ctrl Pts',(-9.10376276046371,-1.93610506340016,
-0.286506702019341));
#27472=CARTESIAN_POINT('Ctrl Pts',(-9.10921860960106,-1.95004927434369,
-0.192276943264637));
#27473=CARTESIAN_POINT('Ctrl Pts',(-9.11467445873842,-1.95643555072192,
-0.0969287540345871));
#27474=CARTESIAN_POINT('Ctrl Pts',(-9.12013030787577,-1.95563441709699,
-0.00147295684208459));
#27475=CARTESIAN_POINT('Ctrl Pts',(-9.22186969212424,-1.95583091145133,
-0.00139679566445557));
#27476=CARTESIAN_POINT('Ctrl Pts',(-9.21683085122553,-1.95654380317051,
-0.0895334992820675));
#27477=CARTESIAN_POINT('Ctrl Pts',(-9.21179201032682,-1.95110047081772,
-0.177581636934776));
#27478=CARTESIAN_POINT('Ctrl Pts',(-9.20675316942811,-1.93920009935021,
-0.264748230860875));
#27479=CARTESIAN_POINT('Ctrl Pts',(-9.16974600373516,-1.85179924118489,
-0.904932878313924));
#27480=CARTESIAN_POINT('Ctrl Pts',(-9.13273883804223,-1.41610616183707,
-1.49756712113799));
#27481=CARTESIAN_POINT('Ctrl Pts',(-9.09573167234929,-0.831135969245425,
-1.77194854656965));
#27482=CARTESIAN_POINT('Ctrl Pts',(-9.05872450665635,-0.246165776653769,
-2.04632997200132));
#27483=CARTESIAN_POINT('Ctrl Pts',(-9.0217173409634,0.488081529181725,-2.00245858004057));
#27484=CARTESIAN_POINT('Ctrl Pts',(-8.98471017527046,1.03621777307301,-1.66037386688404));
#27485=CARTESIAN_POINT('Ctrl Pts',(-8.94770300957752,1.58435401696429,-1.31828915372751));
#27486=CARTESIAN_POINT('Ctrl Pts',(-8.91069584388458,1.94637919891136,-0.677991119375211));
#27487=CARTESIAN_POINT('Ctrl Pts',(-8.87368867819164,1.95692810179956,-0.0319539582997181));
#27488=CARTESIAN_POINT('Ctrl Pts',(-8.8366815124987,1.96747700468776,0.61408320277577));
#27489=CARTESIAN_POINT('Ctrl Pts',(-8.79967434680575,1.62654962851709,1.26585949057444));
#27490=CARTESIAN_POINT('Ctrl Pts',(-8.76266718111281,1.0898741722973,1.62565769448033));
#27491=CARTESIAN_POINT('Ctrl Pts',(-8.72566001541987,0.553198716077507,
1.98545589838623));
#27492=CARTESIAN_POINT('Ctrl Pts',(-8.68865284972692,-0.179224820191409,
2.05327601839933));
#27493=CARTESIAN_POINT('Ctrl Pts',(-8.65164568403398,-0.772841319532216,
1.79813930102413));
#27494=CARTESIAN_POINT('Ctrl Pts',(-8.61463851834104,-1.36645781887302,
1.54300258364892));
#27495=CARTESIAN_POINT('Ctrl Pts',(-8.5776313526481,-1.82126728128571,0.964909028885417));
#27496=CARTESIAN_POINT('Ctrl Pts',(-8.54062418695516,-1.92952265146001,
0.32791917993094));
#27497=CARTESIAN_POINT('Ctrl Pts',(-8.53437268867819,-1.94780987360863,
0.220314588532923));
#27498=CARTESIAN_POINT('Ctrl Pts',(-8.52812119040122,-1.95620774879912,
0.111029318993031));
#27499=CARTESIAN_POINT('Ctrl Pts',(-8.52186969212424,-1.95524099021,0.00159565242000603));
#27500=CARTESIAN_POINT('Origin',(-7.7,0.,0.));
#27501=CARTESIAN_POINT('',(-7.72013030787577,-1.9508822561445,0.000393506593624193));
#27502=CARTESIAN_POINT('',(-7.82186969212424,-1.95084466165673,0.000275628296667681));
#27503=CARTESIAN_POINT('',(-7.7,-1.954,-2.39295984553393E-16));
#27504=CARTESIAN_POINT('Ctrl Pts',(-7.72013030787577,-1.9508822561445,0.000393506593624193));
#27505=CARTESIAN_POINT('Ctrl Pts',(-7.73725513708977,-1.95142606804339,
0.301870604817531));
#27506=CARTESIAN_POINT('Ctrl Pts',(-7.75437996630378,-1.88579578422546,
0.60312340631659));
#27507=CARTESIAN_POINT('Ctrl Pts',(-7.77150479551779,-1.75275564830829,
0.870882623634832));
#27508=CARTESIAN_POINT('Ctrl Pts',(-7.80851196121073,-1.46525273121817,
1.44951669917947));
#27509=CARTESIAN_POINT('Ctrl Pts',(-7.84551912690368,-0.862944158876693,
1.87173491878606));
#27510=CARTESIAN_POINT('Ctrl Pts',(-7.88252629259662,-0.220951367034791,
1.94467719692271));
#27511=CARTESIAN_POINT('Ctrl Pts',(-7.91953345828957,0.421041424807139,
2.01761947505937));
#27512=CARTESIAN_POINT('Ctrl Pts',(-7.95654062398251,1.10271843614949,1.74128581172607));
#27513=CARTESIAN_POINT('Ctrl Pts',(-7.99354778967545,1.51270445718934,1.24189940495405));
#27514=CARTESIAN_POINT('Ctrl Pts',(-8.03055495536839,1.92269047822918,0.742512998182048));
#27515=CARTESIAN_POINT('Ctrl Pts',(-8.06756212106133,2.06098550896654,0.020073847971333));
#27516=CARTESIAN_POINT('Ctrl Pts',(-8.10456928675427,1.86441939184286,-0.595423578762236));
#27517=CARTESIAN_POINT('Ctrl Pts',(-8.14157645244722,1.66785327471917,-1.21092100549583));
#27518=CARTESIAN_POINT('Ctrl Pts',(-8.17858361814016,1.13642600973442,-1.71947670875229));
#27519=CARTESIAN_POINT('Ctrl Pts',(-8.2155907838331,0.512881995447341,-1.88879352115886));
#27520=CARTESIAN_POINT('Ctrl Pts',(-8.25259794952604,-0.110662018839707,
-2.05811033356542));
#27521=CARTESIAN_POINT('Ctrl Pts',(-8.28960511521899,-0.826322782429062,
-1.88818825512213));
#27522=CARTESIAN_POINT('Ctrl Pts',(-8.32661228091193,-1.30720204775987,
-1.45664398984725));
#27523=CARTESIAN_POINT('Ctrl Pts',(-8.35778495656654,-1.71226666393624,
-1.0931362972117));
#27524=CARTESIAN_POINT('Ctrl Pts',(-8.38895763222116,-1.95074455822154,
-0.543997356792516));
#27525=CARTESIAN_POINT('Ctrl Pts',(-8.42013030787577,-1.95544987894172,
0.00153511913569427));
#27526=CARTESIAN_POINT('Ctrl Pts',(-8.52186969212424,-1.95524099021,0.00159565242000603));
#27527=CARTESIAN_POINT('Ctrl Pts',(-8.49111402470827,-1.95048480148194,
-0.536788156406736));
#27528=CARTESIAN_POINT('Ctrl Pts',(-8.4603583572923,-1.71906965971708,-1.07876372514158));
#27529=CARTESIAN_POINT('Ctrl Pts',(-8.42960268987633,-1.3234761506427,-1.44187361781254));
#27530=CARTESIAN_POINT('Ctrl Pts',(-8.39259552418339,-0.847473001715219,
-1.87879042345607));
#27531=CARTESIAN_POINT('Ctrl Pts',(-8.35558835849045,-0.133765425924392,
-2.05673789159769));
#27532=CARTESIAN_POINT('Ctrl Pts',(-8.31858119279751,0.491640502808977,
-1.89443349502208));
#27533=CARTESIAN_POINT('Ctrl Pts',(-8.28157402710457,1.11704643154235,-1.73212909844647));
#27534=CARTESIAN_POINT('Ctrl Pts',(-8.24456686141163,1.65415071321825,-1.22957283715362));
#27535=CARTESIAN_POINT('Ctrl Pts',(-8.20755969571868,1.85761581171597,-0.616321464113222));
#27536=CARTESIAN_POINT('Ctrl Pts',(-8.17055253002574,2.06108091021368,-0.00307009107281909));
#27537=CARTESIAN_POINT('Ctrl Pts',(-8.1335453643328,1.9309068255332,0.72087639371516));
#27538=CARTESIAN_POINT('Ctrl Pts',(-8.09653819863986,1.52655424397296,1.22483500573424));
#27539=CARTESIAN_POINT('Ctrl Pts',(-8.05953103294691,1.12220166241272,1.72879361775331));
#27540=CARTESIAN_POINT('Ctrl Pts',(-8.02252386725398,0.443670583972736,
2.01276435700351));
#27541=CARTESIAN_POINT('Ctrl Pts',(-7.98551670156103,-0.199100775166,1.94703557553326));
#27542=CARTESIAN_POINT('Ctrl Pts',(-7.94850953586809,-0.841872134304755,
1.88130679406301));
#27543=CARTESIAN_POINT('Ctrl Pts',(-7.91150237017514,-1.44888377414225,
1.46587849187229));
#27544=CARTESIAN_POINT('Ctrl Pts',(-7.8744952044822,-1.74286600014233,0.89050926812229));
#27545=CARTESIAN_POINT('Ctrl Pts',(-7.85695336702955,-1.88221707785663,
0.61777740094752));
#27546=CARTESIAN_POINT('Ctrl Pts',(-7.83941152957689,-1.95123442335438,
0.309108840765172));
#27547=CARTESIAN_POINT('Ctrl Pts',(-7.82186969212424,-1.95084466165673,
0.000275628296667681));
#27548=CARTESIAN_POINT('Origin',(-7.7,0.,0.));
#27549=CARTESIAN_POINT('',(-7.02013030787577,-1.95401264958061,-0.00177430195079181));
#27550=CARTESIAN_POINT('',(-7.12186969212424,-1.95423380238351,-0.00176282217937467));
#27551=CARTESIAN_POINT('',(-7.7,-1.954,-2.39295984553393E-16));
#27552=CARTESIAN_POINT('Ctrl Pts',(-7.02013030787577,-1.95401264958061,
-0.00177430195079181));
#27553=CARTESIAN_POINT('Ctrl Pts',(-7.04854547626546,-1.9494508329156,0.496443956289582));
#27554=CARTESIAN_POINT('Ctrl Pts',(-7.07696064465515,-1.75529612755347,
0.997823441204779));
#27555=CARTESIAN_POINT('Ctrl Pts',(-7.10537581304484,-1.41166222317204,
1.35565433444322));
#27556=CARTESIAN_POINT('Ctrl Pts',(-7.14238297873778,-0.964122491478272,
1.82168384989498));
#27557=CARTESIAN_POINT('Ctrl Pts',(-7.17939014443073,-0.263039573894212,
2.04422953948621));
#27558=CARTESIAN_POINT('Ctrl Pts',(-7.21639731012367,0.371347124525088,
1.92163737992699));
#27559=CARTESIAN_POINT('Ctrl Pts',(-7.25340447581661,1.00573382294441,1.79904522036777));
#27560=CARTESIAN_POINT('Ctrl Pts',(-7.29041164150955,1.57342430219897,1.33131521165807));
#27561=CARTESIAN_POINT('Ctrl Pts',(-7.3274188072025,1.8151099173736,0.732096233208271));
#27562=CARTESIAN_POINT('Ctrl Pts',(-7.36442597289544,2.05679553254821,0.132877254758492));
#27563=CARTESIAN_POINT('Ctrl Pts',(-7.40143313858838,1.97247628364293,-0.597830693431359));
#27564=CARTESIAN_POINT('Ctrl Pts',(-7.43844030428132,1.60066736683049,-1.12625613764794));
#27565=CARTESIAN_POINT('Ctrl Pts',(-7.47544746997426,1.22885845001806,-1.65468158186452));
#27566=CARTESIAN_POINT('Ctrl Pts',(-7.5124546356672,0.569559865298466,-1.98082452210781));
#27567=CARTESIAN_POINT('Ctrl Pts',(-7.54946180136014,-0.0760751553371205,
-1.95570996765015));
#27568=CARTESIAN_POINT('Ctrl Pts',(-7.58646896705309,-0.721710175972735,
-1.93059541319249));
#27569=CARTESIAN_POINT('Ctrl Pts',(-7.62347613274604,-1.35368163252435,
-1.55422336403385));
#27570=CARTESIAN_POINT('Ctrl Pts',(-7.66048329843898,-1.68331872988077,
-0.998512373713166));
#27571=CARTESIAN_POINT('Ctrl Pts',(-7.68036563491791,-1.86041836890632,
-0.699953089647185));
#27572=CARTESIAN_POINT('Ctrl Pts',(-7.70024797139684,-1.9502508775176,-0.349628618162857));
#27573=CARTESIAN_POINT('Ctrl Pts',(-7.72013030787577,-1.9508822561445,0.000393506593624193));
#27574=CARTESIAN_POINT('Ctrl Pts',(-7.82186969212424,-1.95084466165673,
0.000275628296667681));
#27575=CARTESIAN_POINT('Ctrl Pts',(-7.80240436388396,-1.9504121619599,-0.342421644348059));
#27576=CARTESIAN_POINT('Ctrl Pts',(-7.78293903564367,-1.8645168377084,-0.685321657749648));
#27577=CARTESIAN_POINT('Ctrl Pts',(-7.76347370740338,-1.69442477712935,
-0.979547510697657));
#27578=CARTESIAN_POINT('Ctrl Pts',(-7.72646654171044,-1.37104851595361,
-1.53892492045839));
#27579=CARTESIAN_POINT('Ctrl Pts',(-7.68945937601749,-0.743343181439431,
-1.92236959467059));
#27580=CARTESIAN_POINT('Ctrl Pts',(-7.65245221032455,-0.0980308970802916,
-1.95473235873392));
#27581=CARTESIAN_POINT('Ctrl Pts',(-7.61544504463161,0.547281387278848,
-1.98709512279725));
#27582=CARTESIAN_POINT('Ctrl Pts',(-7.57843787893867,1.21020062148296,-1.6683759767117));
#27583=CARTESIAN_POINT('Ctrl Pts',(-7.54143071324573,1.58791973972498,-1.1441588837463));
#27584=CARTESIAN_POINT('Ctrl Pts',(-7.50442354755279,1.965638857967,-0.619941790780907));
#27585=CARTESIAN_POINT('Ctrl Pts',(-7.46741638185984,2.05815786024695,0.10977324906432));
#27586=CARTESIAN_POINT('Ctrl Pts',(-7.4304092161669,1.82321608166587,0.711668300979329));
#27587=CARTESIAN_POINT('Ctrl Pts',(-7.39340205047395,1.58827430308477,1.31356335289435));
#27588=CARTESIAN_POINT('Ctrl Pts',(-7.35639488478102,1.02587174364262,1.78763841687913));
#27589=CARTESIAN_POINT('Ctrl Pts',(-7.31938771908808,0.39290164167109,1.91734633048805));
#27590=CARTESIAN_POINT('Ctrl Pts',(-7.28238055339514,-0.240068460300431,
2.04705424409697));
#27591=CARTESIAN_POINT('Ctrl Pts',(-7.24537338770219,-0.943606104801338,
1.83239500733005));
#27592=CARTESIAN_POINT('Ctrl Pts',(-7.20836622200925,-1.39635062099231,
1.37142028361776));
#27593=CARTESIAN_POINT('Ctrl Pts',(-7.17953404538091,-1.74908257476143,
1.01227619877891));
#27594=CARTESIAN_POINT('Ctrl Pts',(-7.15070186875258,-1.94958502072792,
0.503620500146864));
#27595=CARTESIAN_POINT('Ctrl Pts',(-7.12186969212424,-1.95423380238351,
-0.00176282217937467));
#27596=CARTESIAN_POINT('Origin',(-7.7,0.,0.));
#27597=CARTESIAN_POINT('',(-6.32013030787576,-1.95674715409565,0.000835936956466929));
#27598=CARTESIAN_POINT('',(-6.42186969212424,-1.95661254207068,0.000950563181825557));
#27599=CARTESIAN_POINT('',(-7.7,-1.954,-2.39295984553393E-16));
#27600=CARTESIAN_POINT('Ctrl Pts',(-6.32013030787576,-1.95674715409565,
0.000835936956466929));
#27601=CARTESIAN_POINT('Ctrl Pts',(-6.3228286497482,-1.95700108945633,0.0479758079941679));
#27602=CARTESIAN_POINT('Ctrl Pts',(-6.32552699162063,-1.95544487187201,
0.0950986300560049));
#27603=CARTESIAN_POINT('Ctrl Pts',(-6.32822533349306,-1.95202472787979,
0.142085778920809));
#27604=CARTESIAN_POINT('Ctrl Pts',(-6.365232499186,-1.9051182047639,0.78650419796693));
#27605=CARTESIAN_POINT('Ctrl Pts',(-6.40223966487895,-1.50761607859282,
1.40540314042301));
#27606=CARTESIAN_POINT('Ctrl Pts',(-6.43924683057189,-0.941088661808038,
1.71608305085799));
#27607=CARTESIAN_POINT('Ctrl Pts',(-6.47625399626483,-0.374561245023235,
2.02676296129299));
#27608=CARTESIAN_POINT('Ctrl Pts',(-6.51326116195777,0.360991462375277,
2.02922383970686));
#27609=CARTESIAN_POINT('Ctrl Pts',(-6.55026832765071,0.929585006201032,
1.72234161044549));
#27610=CARTESIAN_POINT('Ctrl Pts',(-6.58727549334365,1.49817855002677,1.41545938118412));
#27611=CARTESIAN_POINT('Ctrl Pts',(-6.6242826590366,1.89981293027976,0.799234044247542));
#27612=CARTESIAN_POINT('Ctrl Pts',(-6.66128982472954,1.95103031086682,0.155143910304678));
#27613=CARTESIAN_POINT('Ctrl Pts',(-6.69829699042249,2.00224769145389,-0.488946223638195));
#27614=CARTESIAN_POINT('Ctrl Pts',(-6.73530415611543,1.70304807237501,-1.16090115458735));
#27615=CARTESIAN_POINT('Ctrl Pts',(-6.77231132180837,1.19009932215664,-1.55378650728729));
#27616=CARTESIAN_POINT('Ctrl Pts',(-6.80931848750131,0.677150571938273,
-1.94667185998723));
#27617=CARTESIAN_POINT('Ctrl Pts',(-6.84632565319425,-0.0495473094195792,
-2.06048763443796));
#27618=CARTESIAN_POINT('Ctrl Pts',(-6.88333281888719,-0.658054559381064,
-1.84324526412073));
#27619=CARTESIAN_POINT('Ctrl Pts',(-6.92033998458013,-1.26656180934255,
-1.62600289380351));
#27620=CARTESIAN_POINT('Ctrl Pts',(-6.95734715027308,-1.75687842790767,
-1.07770237871833));
#27621=CARTESIAN_POINT('Ctrl Pts',(-6.99435431596602,-1.90503846428849,
-0.448795450519591));
#27622=CARTESIAN_POINT('Ctrl Pts',(-7.00294631326927,-1.93943695466724,
-0.302781387299679));
#27623=CARTESIAN_POINT('Ctrl Pts',(-7.01153831057252,-1.95539202259527,
-0.152422359795286));
#27624=CARTESIAN_POINT('Ctrl Pts',(-7.02013030787577,-1.95401264958061,
-0.00177430195079181));
#27625=CARTESIAN_POINT('Ctrl Pts',(-7.12186969212424,-1.95423380238351,
-0.00176282217937467));
#27626=CARTESIAN_POINT('Ctrl Pts',(-7.11369470305964,-1.95555190402003,
-0.145057696746382));
#27627=CARTESIAN_POINT('Ctrl Pts',(-7.10551971399503,-1.94112469613282,
-0.288089494398315));
#27628=CARTESIAN_POINT('Ctrl Pts',(-7.09734472493042,-1.9099577897608,-0.427375587037744));
#27629=CARTESIAN_POINT('Ctrl Pts',(-7.06033755923749,-1.76886905445728,
-1.05790652332323));
#27630=CARTESIAN_POINT('Ctrl Pts',(-7.02333039354454,-1.28474019596922,
-1.61167818523655));
#27631=CARTESIAN_POINT('Ctrl Pts',(-6.9863232278516,-0.678710731069402,
-1.83573974043029));
#27632=CARTESIAN_POINT('Ctrl Pts',(-6.94931606215865,-0.0726812661695574,
-2.05980129562404));
#27633=CARTESIAN_POINT('Ctrl Pts',(-6.91230889646571,0.655248805142062,
-1.95415274409816));
#27634=CARTESIAN_POINT('Ctrl Pts',(-6.87530173077277,1.17257688279952,-1.56705204284606));
#27635=CARTESIAN_POINT('Ctrl Pts',(-6.83829456507983,1.68990496045699,-1.17995134159395));
#27636=CARTESIAN_POINT('Ctrl Pts',(-6.80128739938689,1.99663104446028,-0.511398490615602));
#27637=CARTESIAN_POINT('Ctrl Pts',(-6.76428023369395,1.95264934105456,0.133226130856597));
#27638=CARTESIAN_POINT('Ctrl Pts',(-6.72727306800101,1.90866763764884,0.777850752328768));
#27639=CARTESIAN_POINT('Ctrl Pts',(-6.69026590230807,1.51397814683413,1.3985471442948));
#27640=CARTESIAN_POINT('Ctrl Pts',(-6.65325873661513,0.948866430488816,
1.71179471554134));
#27641=CARTESIAN_POINT('Ctrl Pts',(-6.61625157092218,0.383754714143482,
2.02504228678789));
#27642=CARTESIAN_POINT('Ctrl Pts',(-6.57924440522924,-0.351779227732472,
2.03084103731494));
#27643=CARTESIAN_POINT('Ctrl Pts',(-6.54223723953629,-0.921759512634525,
1.72654222419598));
#27644=CARTESIAN_POINT('Ctrl Pts',(-6.50523007384335,-1.49173979753657,
1.42224341107702));
#27645=CARTESIAN_POINT('Ctrl Pts',(-6.46822290815041,-1.89616642546472,
0.807847034312071));
#27646=CARTESIAN_POINT('Ctrl Pts',(-6.43121574245747,-1.95030612241134,
0.16399597540392));
#27647=CARTESIAN_POINT('Ctrl Pts',(-6.4281003923464,-1.95486372923526,0.109795081324937));
#27648=CARTESIAN_POINT('Ctrl Pts',(-6.42498504223532,-1.9569389689582,0.0553854516995903));
#27649=CARTESIAN_POINT('Ctrl Pts',(-6.42186969212424,-1.95661254207068,
0.000950563181825557));
#27650=CARTESIAN_POINT('Origin',(-7.7,0.,0.));
#27651=CARTESIAN_POINT('',(-5.62013030787577,-1.95157062279887,0.00118915835141939));
#27652=CARTESIAN_POINT('',(-5.72186969212424,-1.95144011146387,0.00109661375529725));
#27653=CARTESIAN_POINT('',(-7.7,-1.954,-2.39295984553393E-16));
#27654=CARTESIAN_POINT('Ctrl Pts',(-5.62013030787577,-1.95157062279887,
0.00118915835141939));
#27655=CARTESIAN_POINT('Ctrl Pts',(-5.63411898892388,-1.95294121534163,
0.247238073111425));
#27656=CARTESIAN_POINT('Ctrl Pts',(-5.648107669972,-1.9098072184107,0.492824110420985));
#27657=CARTESIAN_POINT('Ctrl Pts',(-5.66209635102011,-1.8199678581088,0.719934651393151));
#27658=CARTESIAN_POINT('Ctrl Pts',(-5.69910351671305,-1.58229712410575,
1.32075737309663));
#27659=CARTESIAN_POINT('Ctrl Pts',(-5.73611068240599,-1.01774901009749,
1.79227541967969));
#27660=CARTESIAN_POINT('Ctrl Pts',(-5.77311784809893,-0.384196797004847,
1.9191096185463));
#27661=CARTESIAN_POINT('Ctrl Pts',(-5.81012501379187,0.249355416087819,
2.04594381741292));
#27662=CARTESIAN_POINT('Ctrl Pts',(-5.84713217948482,0.951911728264895,
1.82809416856304));
#27663=CARTESIAN_POINT('Ctrl Pts',(-5.88413934517776,1.40255971991618,1.36506964616989));
#27664=CARTESIAN_POINT('Ctrl Pts',(-5.92114651087071,1.85320771156745,0.902045123776732));
#27665=CARTESIAN_POINT('Ctrl Pts',(-5.95815367656364,2.05194738269297,0.1938457278403));
#27666=CARTESIAN_POINT('Ctrl Pts',(-5.99516084225658,1.90799878067116,-0.436038484291347));
#27667=CARTESIAN_POINT('Ctrl Pts',(-6.03216800794953,1.76405017864935,-1.065922696423));
#27668=CARTESIAN_POINT('Ctrl Pts',(-6.06917517364247,1.27741330348022,-1.61749172474984));
#27669=CARTESIAN_POINT('Ctrl Pts',(-6.10618233933541,0.670373279324294,
-1.83880085196677));
#27670=CARTESIAN_POINT('Ctrl Pts',(-6.14318950502836,0.0633332551683667,
-2.0601099791837));
#27671=CARTESIAN_POINT('Ctrl Pts',(-6.1801966707213,-0.664109917974376,
-1.95115920529068));
#27672=CARTESIAN_POINT('Ctrl Pts',(-6.21720383641424,-1.17967604451539,
-1.56171487052607));
#27673=CARTESIAN_POINT('Ctrl Pts',(-6.25151266023475,-1.65765016309781,
-1.20066649464673));
#27674=CARTESIAN_POINT('Ctrl Pts',(-6.28582148405525,-1.95351842179887,
-0.598537162085356));
#27675=CARTESIAN_POINT('Ctrl Pts',(-6.32013030787576,-1.95674715409565,
0.000835936956466929));
#27676=CARTESIAN_POINT('Ctrl Pts',(-6.42186969212424,-1.95661254207068,
0.000950563181825557));
#27677=CARTESIAN_POINT('Ctrl Pts',(-6.38797787654238,-1.95306135216312,
-0.591245221267486));
#27678=CARTESIAN_POINT('Ctrl Pts',(-6.35408606096051,-1.6652678890792,-1.1864304485344));
#27679=CARTESIAN_POINT('Ctrl Pts',(-6.32019424537865,-1.19713802583512,
-1.54836985186468));
#27680=CARTESIAN_POINT('Ctrl Pts',(-6.2831870796857,-0.685977466347171,
-1.94357887917377));
#27681=CARTESIAN_POINT('Ctrl Pts',(-6.24617991399276,0.0401964185938104,
-2.06069119274061));
#27682=CARTESIAN_POINT('Ctrl Pts',(-6.20917274829982,0.649683216600975,
-1.84621243878673));
#27683=CARTESIAN_POINT('Ctrl Pts',(-6.17216558260688,1.25917001460814,-1.63173368483286));
#27684=CARTESIAN_POINT('Ctrl Pts',(-6.13515841691393,1.75196972568149,-1.08566386335827));
#27685=CARTESIAN_POINT('Ctrl Pts',(-6.09815125122099,1.90298217646455,-0.457435773767298));
#27686=CARTESIAN_POINT('Ctrl Pts',(-6.06114408552805,2.05399462724761,0.170792315823676));
#27687=CARTESIAN_POINT('Ctrl Pts',(-6.02413691983511,1.86321981774039,0.881178673531042));
#27688=CARTESIAN_POINT('Ctrl Pts',(-5.98712975414217,1.41779952527589,1.34923428550837));
#27689=CARTESIAN_POINT('Ctrl Pts',(-5.95012258844923,0.972379232811401,
1.81728989748569));
#27690=CARTESIAN_POINT('Ctrl Pts',(-5.91311542275628,0.272313457389638,
2.04301476373299));
#27691=CARTESIAN_POINT('Ctrl Pts',(-5.87610825706334,-0.362623004317677,
1.92330268231588));
#27692=CARTESIAN_POINT('Ctrl Pts',(-5.8391010913704,-0.997559466024982,
1.80359060089877));
#27693=CARTESIAN_POINT('Ctrl Pts',(-5.80209392567746,-1.56736661401784,
1.33844157181727));
#27694=CARTESIAN_POINT('Ctrl Pts',(-5.76508675998452,-1.81176895520886,
0.740325539209087));
#27695=CARTESIAN_POINT('Ctrl Pts',(-5.75068107069776,-1.90690685951008,
0.507498367447963));
#27696=CARTESIAN_POINT('Ctrl Pts',(-5.736275381411,-1.9527364216002,0.254522807047113));
#27697=CARTESIAN_POINT('Ctrl Pts',(-5.72186969212424,-1.95144011146387,
0.00109661375529725));
#27698=CARTESIAN_POINT('Origin',(-7.7,0.,0.));
#27699=CARTESIAN_POINT('',(-4.92013030787577,-1.95245193048433,-0.00158706406638287));
#27700=CARTESIAN_POINT('',(-5.02186969212424,-1.95264185663859,-0.00163836777318162));
#27701=CARTESIAN_POINT('',(-7.7,-1.954,-2.39295984553393E-16));
#27702=CARTESIAN_POINT('Ctrl Pts',(-4.92013030787577,-1.95245193048433,
-0.00158706406638287));
#27703=CARTESIAN_POINT('Ctrl Pts',(-4.94540932809956,-1.94904718301888,
0.442544332783492));
#27704=CARTESIAN_POINT('Ctrl Pts',(-4.97068834832336,-1.79874664837135,
0.88876049721347));
#27705=CARTESIAN_POINT('Ctrl Pts',(-4.99596736854716,-1.52098034279809,
1.23174985433226));
#27706=CARTESIAN_POINT('Ctrl Pts',(-5.0329745342401,-1.11434497468405,1.73386836436301));
#27707=CARTESIAN_POINT('Ctrl Pts',(-5.06998169993304,-0.4345322164979,2.01475705244277));
#27708=CARTESIAN_POINT('Ctrl Pts',(-5.10698886562598,0.207934272190149,
1.94611208445826));
#27709=CARTESIAN_POINT('Ctrl Pts',(-5.14399603131892,0.850400760878179,
1.87746711647375));
#27710=CARTESIAN_POINT('Ctrl Pts',(-5.18100319701187,1.45552098006812,1.45928849242499));
#27711=CARTESIAN_POINT('Ctrl Pts',(-5.21801036270481,1.74688919497478,0.882591098587607));
#27712=CARTESIAN_POINT('Ctrl Pts',(-5.25501752839775,2.03825740988146,0.305893704750204));
#27713=CARTESIAN_POINT('Ctrl Pts',(-5.29202469409069,2.01587362050484,-0.42932245887581));
#27714=CARTESIAN_POINT('Ctrl Pts',(-5.32903185978363,1.68996225424583,-0.98722666396835));
#27715=CARTESIAN_POINT('Ctrl Pts',(-5.36603902547657,1.36405088798683,-1.54513086906087));
#27716=CARTESIAN_POINT('Ctrl Pts',(-5.40304619116952,0.734611944845429,
-1.92572311561991));
#27717=CARTESIAN_POINT('Ctrl Pts',(-5.44005335686246,0.0891594229728106,
-1.95515715586264));
#27718=CARTESIAN_POINT('Ctrl Pts',(-5.4770605225554,-0.556293098899808,
-1.98459119610536));
#27719=CARTESIAN_POINT('Ctrl Pts',(-5.51406768824834,-1.21775919950366,
-1.66286703003176));
#27720=CARTESIAN_POINT('Ctrl Pts',(-5.55107485394128,-1.59309557280667,
-1.13694124858302));
#27721=CARTESIAN_POINT('Ctrl Pts',(-5.57409333858611,-1.82655507676345,
-0.809815020515635));
#27722=CARTESIAN_POINT('Ctrl Pts',(-5.59711182323094,-1.94931530199406,
-0.40368626534284));
#27723=CARTESIAN_POINT('Ctrl Pts',(-5.62013030787577,-1.95157062279887,
0.00118915835141939));
#27724=CARTESIAN_POINT('Ctrl Pts',(-5.72186969212424,-1.95144011146387,
0.00109661375529725));
#27725=CARTESIAN_POINT('Ctrl Pts',(-5.69926821571806,-1.94940629535287,
-0.396510610333469));
#27726=CARTESIAN_POINT('Ctrl Pts',(-5.67666673931187,-1.8313706242534,-0.795227081822891));
#27727=CARTESIAN_POINT('Ctrl Pts',(-5.65406526290569,-1.60576172018975,
-1.11898076347947));
#27728=CARTESIAN_POINT('Ctrl Pts',(-5.61705809721275,-1.23635460959044,
-1.64908799742492));
#27729=CARTESIAN_POINT('Ctrl Pts',(-5.58005093151981,-0.578542854002666,
-1.97821942918092));
#27730=CARTESIAN_POINT('Ctrl Pts',(-5.54304376582687,0.0671994657422203,
-1.95603499019516));
#27731=CARTESIAN_POINT('Ctrl Pts',(-5.50603660013393,0.712941785487116,
-1.9338505512094));
#27732=CARTESIAN_POINT('Ctrl Pts',(-5.46902943444098,1.34661466938912,-1.56035024148186));
#27733=CARTESIAN_POINT('Ctrl Pts',(-5.43202226874804,1.6787701473856,-1.00614086653448));
#27734=CARTESIAN_POINT('Ctrl Pts',(-5.3950151030551,2.01092562538208,-0.451931491587115));
#27735=CARTESIAN_POINT('Ctrl Pts',(-5.35800793736216,2.04156369747304,0.282986948580081));
#27736=CARTESIAN_POINT('Ctrl Pts',(-5.32100077166922,1.75668955971682,0.862919719235671));
#27737=CARTESIAN_POINT('Ctrl Pts',(-5.28399360597628,1.4718154219606,1.44285248989126));
#27738=CARTESIAN_POINT('Ctrl Pts',(-5.24698644028333,0.871429074357163,
1.86779959103526));
#27739=CARTESIAN_POINT('Ctrl Pts',(-5.20997927459039,0.229773922269001,
1.94365444349271));
#27740=CARTESIAN_POINT('Ctrl Pts',(-5.17297210889745,-0.411881229819169,
2.01950929595016));
#27741=CARTESIAN_POINT('Ctrl Pts',(-5.13596494320451,-1.09480518639206,
1.74627189972109));
#27742=CARTESIAN_POINT('Ctrl Pts',(-5.09895777751157,-1.50705316022771,
1.24875114546955));
#27743=CARTESIAN_POINT('Ctrl Pts',(-5.07326174904912,-1.79329868784144,
0.903296225523015));
#27744=CARTESIAN_POINT('Ctrl Pts',(-5.04756572058668,-1.94904434446389,
0.449708515251178));
#27745=CARTESIAN_POINT('Ctrl Pts',(-5.02186969212424,-1.95264185663859,
-0.00163836777318162));
#27746=CARTESIAN_POINT('Origin',(-7.7,0.,0.));
#27747=CARTESIAN_POINT('',(-4.22013030787576,-1.95717603808304,-0.000142023995625407));
#27748=CARTESIAN_POINT('',(-4.32186969212423,-1.95718893672642,-6.75583561184207E-6));
#27749=CARTESIAN_POINT('',(-7.7,-1.954,-2.39295984553393E-16));
#27750=CARTESIAN_POINT('Ctrl Pts',(-4.22013030787576,-1.95717603808304,
-0.000142023995625407));
#27751=CARTESIAN_POINT('Ctrl Pts',(-4.25669966727524,-1.95650647305912,
0.638348883812147));
#27752=CARTESIAN_POINT('Ctrl Pts',(-4.29326902667472,-1.6144202457463,1.27745536120794));
#27753=CARTESIAN_POINT('Ctrl Pts',(-4.3298383860742,-1.08248584150121,1.63058679921527));
#27754=CARTESIAN_POINT('Ctrl Pts',(-4.36684555176715,-0.544183148784234,
1.98794590673933));
#27755=CARTESIAN_POINT('Ctrl Pts',(-4.40385271746009,0.188540634495529,
2.05244163295488));
#27756=CARTESIAN_POINT('Ctrl Pts',(-4.44085988315303,0.780993245066536,
1.79461373503777));
#27757=CARTESIAN_POINT('Ctrl Pts',(-4.47786704884597,1.37344585563752,1.53678583712066));
#27758=CARTESIAN_POINT('Ctrl Pts',(-4.51487421453891,1.82562729349976,0.956634315070912));
#27759=CARTESIAN_POINT('Ctrl Pts',(-4.55188138023185,1.93099092771133,0.319159746713509));
#27760=CARTESIAN_POINT('Ctrl Pts',(-4.5888885459248,2.03635456192291,-0.318314821643903));
#27761=CARTESIAN_POINT('Ctrl Pts',(-4.62589571161774,1.79490039248382,-1.01311243630897));
#27762=CARTESIAN_POINT('Ctrl Pts',(-4.66290287731068,1.31691942439483,-1.44786468168724));
#27763=CARTESIAN_POINT('Ctrl Pts',(-4.69991004300362,0.838938456305839,
-1.88261692706552));
#27764=CARTESIAN_POINT('Ctrl Pts',(-4.73691720869656,0.124430689566952,
-2.057323803157));
#27765=CARTESIAN_POINT('Ctrl Pts',(-4.77392437438951,-0.5002322921065,-1.89218301460498));
#27766=CARTESIAN_POINT('Ctrl Pts',(-4.81093154008245,-1.12489527377994,
-1.72704222605298));
#27767=CARTESIAN_POINT('Ctrl Pts',(-4.84793870577539,-1.65971347038795,
-1.22205377285749));
#27768=CARTESIAN_POINT('Ctrl Pts',(-4.88494587146833,-1.860393579671,-0.607885380268879));
#27769=CARTESIAN_POINT('Ctrl Pts',(-4.89667401693748,-1.92399222253827,
-0.413245879622015));
#27770=CARTESIAN_POINT('Ctrl Pts',(-4.90840216240662,-1.95403155553336,
-0.207640842399378));
#27771=CARTESIAN_POINT('Ctrl Pts',(-4.92013030787577,-1.95245193048433,
-0.00158706406638287));
#27772=CARTESIAN_POINT('Ctrl Pts',(-5.02186969212424,-1.95264185663859,
-0.00163836777318162));
#27773=CARTESIAN_POINT('Ctrl Pts',(-5.01055855489374,-1.9542254458674,-0.200316795449617));
#27774=CARTESIAN_POINT('Ctrl Pts',(-4.99924741766324,-1.92632769683691,
-0.398561024034741));
#27775=CARTESIAN_POINT('Ctrl Pts',(-4.98793628043274,-1.86710213185347,
-0.586956795933102));
#27776=CARTESIAN_POINT('Ctrl Pts',(-4.9509291147398,-1.67333113854519,-1.20333987081021));
#27777=CARTESIAN_POINT('Ctrl Pts',(-4.91392194904685,-1.14421716083023,
-1.71430190829039));
#27778=CARTESIAN_POINT('Ctrl Pts',(-4.87691478335391,-0.521447938032845,
-1.88644657994472));
#27779=CARTESIAN_POINT('Ctrl Pts',(-4.83990761766097,0.10132128476453,-2.05859125159905));
#27780=CARTESIAN_POINT('Ctrl Pts',(-4.80290045196803,0.817745752644318,
-1.89191855742752));
#27781=CARTESIAN_POINT('Ctrl Pts',(-4.76589328627509,1.30057837456157,-1.46256095349446));
#27782=CARTESIAN_POINT('Ctrl Pts',(-4.72888612058215,1.78341099647882,-1.0332033495614));
#27783=CARTESIAN_POINT('Ctrl Pts',(-4.6918789548892,2.03265177243352,-0.341160835866783));
#27784=CARTESIAN_POINT('Ctrl Pts',(-4.65487178919626,1.93445294518429,0.297456642103794));
#27785=CARTESIAN_POINT('Ctrl Pts',(-4.61786462350332,1.83625411793506,0.936074120074369));
#27786=CARTESIAN_POINT('Ctrl Pts',(-4.58085745781037,1.3906156874819,1.52126656232092));
#27787=CARTESIAN_POINT('Ctrl Pts',(-4.54385029211743,0.801095581508699,
1.785730808479));
#27788=CARTESIAN_POINT('Ctrl Pts',(-4.50684312642449,0.211575475535495,
2.05019505463709));
#27789=CARTESIAN_POINT('Ctrl Pts',(-4.46983596073155,-0.521826305957753,
1.99393110470671));
#27790=CARTESIAN_POINT('Ctrl Pts',(-4.43282879503861,-1.06410780488448,
1.6426391054178));
#27791=CARTESIAN_POINT('Ctrl Pts',(-4.39584242740049,-1.60608454120294,
1.2915445324954));
#27792=CARTESIAN_POINT('Ctrl Pts',(-4.35885605976236,-1.95715575407421,
0.645753429000468));
#27793=CARTESIAN_POINT('Ctrl Pts',(-4.32186969212423,-1.95718893672642,
-6.75583561184207E-6));
#27794=CARTESIAN_POINT('Origin',(-7.7,0.,0.));
#27795=CARTESIAN_POINT('',(-3.52013030787576,-1.95285875419799,0.00168591294888436));
#27796=CARTESIAN_POINT('',(-3.62186969212424,-1.95266119647961,0.00164306867381859));
#27797=CARTESIAN_POINT('',(-7.7,-1.954,-2.39295984553393E-16));
#27798=CARTESIAN_POINT('Ctrl Pts',(-3.52013030787576,-1.95285875419799,
0.00168591294888436));
#27799=CARTESIAN_POINT('Ctrl Pts',(-3.53098284075798,-1.95443499456628,
0.192255467216998));
#27800=CARTESIAN_POINT('Ctrl Pts',(-3.5418353736402,-1.9287959273972,0.382409993933235));
#27801=CARTESIAN_POINT('Ctrl Pts',(-3.55268790652243,-1.87420812867872,
0.56385529812026));
#27802=CARTESIAN_POINT('Ctrl Pts',(-3.58969507221537,-1.6880635913701,1.18258426297381));
#27803=CARTESIAN_POINT('Ctrl Pts',(-3.62670223790831,-1.1652997890823,1.70004136099891));
#27804=CARTESIAN_POINT('Ctrl Pts',(-3.66370940360125,-0.544703839327083,
1.87986346159656));
#27805=CARTESIAN_POINT('Ctrl Pts',(-3.70071656929419,0.0758921104281432,
2.05968556219421));
#27806=CARTESIAN_POINT('Ctrl Pts',(-3.73772373498713,0.794320207650795,
1.9018726653644));
#27807=CARTESIAN_POINT('Ctrl Pts',(-3.77473090068007,1.28241814705543,1.47851026473626));
#27808=CARTESIAN_POINT('Ctrl Pts',(-3.81173806637301,1.77051608646007,1.05514786410812));
#27809=CARTESIAN_POINT('Ctrl Pts',(-3.84874523206596,2.02828386804669,0.366235959681632));
#27810=CARTESIAN_POINT('Ctrl Pts',(-3.8857523977589,1.93797878414602,-0.27354549717586));
#27811=CARTESIAN_POINT('Ctrl Pts',(-3.92275956345184,1.84767370024536,-0.913326954033334));
#27812=CARTESIAN_POINT('Ctrl Pts',(-3.95976672914478,1.40929575085742,-1.50397796332182));
#27813=CARTESIAN_POINT('Ctrl Pts',(-3.99677389483772,0.823086434070165,
-1.77570201015686));
#27814=CARTESIAN_POINT('Ctrl Pts',(-4.03378106053066,0.236877117282891,
-2.04742605699191));
#27815=CARTESIAN_POINT('Ctrl Pts',(-4.07078822622361,-0.497163566903715,
-2.0002231413735));
#27816=CARTESIAN_POINT('Ctrl Pts',(-4.10779539191655,-1.04374182356972,
-1.65565452693409));
#27817=CARTESIAN_POINT('Ctrl Pts',(-4.14480255760949,-1.59032008023574,
-1.31108591249467));
#27818=CARTESIAN_POINT('Ctrl Pts',(-4.18180972330244,-1.94943590938115,
-0.669151599234243));
#27819=CARTESIAN_POINT('Ctrl Pts',(-4.21881688899538,-1.95705302287675,
-0.0230731981877537));
#27820=CARTESIAN_POINT('Ctrl Pts',(-4.21925469528884,-1.95714313570123,
-0.0154298895270845));
#27821=CARTESIAN_POINT('Ctrl Pts',(-4.2196925015823,-1.95718405407747,-0.00778600087535643));
#27822=CARTESIAN_POINT('Ctrl Pts',(-4.22013030787576,-1.95717603808304,
-0.000142023995625407));
#27823=CARTESIAN_POINT('Ctrl Pts',(-4.32186969212423,-1.95718893672642,
-6.75583561184207E-6));
#27824=CARTESIAN_POINT('Ctrl Pts',(-4.28484172837648,-1.95722215669696,
-0.646493184235486));
#27825=CARTESIAN_POINT('Ctrl Pts',(-4.24781376462872,-1.60524684540183,
-1.29294852331618));
#27826=CARTESIAN_POINT('Ctrl Pts',(-4.21078580088096,-1.06226722191928,
-1.64382997913402));
#27827=CARTESIAN_POINT('Ctrl Pts',(-4.17377863518802,-0.519592581990526,
-1.99451435007294));
#27828=CARTESIAN_POINT('Ctrl Pts',(-4.13677146949508,0.213871760525216,
-2.04995678343623));
#27829=CARTESIAN_POINT('Ctrl Pts',(-4.09976430380213,0.803095271029007,
-1.78483238336676));
#27830=CARTESIAN_POINT('Ctrl Pts',(-4.06275713810919,1.3923187815328,-1.51970798329728));
#27831=CARTESIAN_POINT('Ctrl Pts',(-4.02574997241625,1.83730146002465,-0.93401674979504));
#27832=CARTESIAN_POINT('Ctrl Pts',(-3.98874280672331,1.93478491203242,-0.295289680204818));
#27833=CARTESIAN_POINT('Ctrl Pts',(-3.95173564103036,2.03226836404019,0.343437389385403));
#27834=CARTESIAN_POINT('Ctrl Pts',(-3.91472847533742,1.7822525895639,1.03520029506359));
#27835=CARTESIAN_POINT('Ctrl Pts',(-3.87772130964448,1.29893934828762,1.46401681019524));
#27836=CARTESIAN_POINT('Ctrl Pts',(-3.84071414395154,0.815626107011349,
1.89283332532687));
#27837=CARTESIAN_POINT('Ctrl Pts',(-3.8037069782586,0.0990153989350884,
2.05870344991196));
#27838=CARTESIAN_POINT('Ctrl Pts',(-3.76669981256566,-0.523560614431006,
1.8858613241912));
#27839=CARTESIAN_POINT('Ctrl Pts',(-3.72969264687271,-1.14613662779711,
1.71301919847044));
#27840=CARTESIAN_POINT('Ctrl Pts',(-3.69268548117977,-1.67467794645305,
1.20146482244383));
#27841=CARTESIAN_POINT('Ctrl Pts',(-3.65567831548683,-1.86775840925908,
0.584865091884778));
#27842=CARTESIAN_POINT('Ctrl Pts',(-3.64440877436597,-1.92655589278652,
0.397096158800172));
#27843=CARTESIAN_POINT('Ctrl Pts',(-3.6331392332451,-1.95424461873575,0.199585908921427));
#27844=CARTESIAN_POINT('Ctrl Pts',(-3.62186969212424,-1.95266119647961,
0.00164306867381859));
#27845=CARTESIAN_POINT('Origin',(-7.7,0.,0.));
#27846=CARTESIAN_POINT('',(-2.82013030787576,-1.95130973680355,-0.000989162390181431));
#27847=CARTESIAN_POINT('',(-2.92186969212423,-1.95142771007674,-0.00108710473741568));
#27848=CARTESIAN_POINT('',(-7.7,-1.954,-2.39295984553393E-16));
#27849=CARTESIAN_POINT('Ctrl Pts',(-2.82013030787576,-1.95130973680355,
-0.000989162390181431));
#27850=CARTESIAN_POINT('Ctrl Pts',(-2.84227317993367,-1.94951961830664,
0.388615496325764));
#27851=CARTESIAN_POINT('Ctrl Pts',(-2.86441605199157,-1.83655492906094,
0.779176241682102));
#27852=CARTESIAN_POINT('Ctrl Pts',(-2.88655892404947,-1.61945757610167,
1.09906599712299));
#27853=CARTESIAN_POINT('Ctrl Pts',(-2.92356608974241,-1.25662489154953,
1.6336946194679));
#27854=CARTESIAN_POINT('Ctrl Pts',(-2.96057325543535,-0.602927702481477,
1.97092425351893));
#27855=CARTESIAN_POINT('Ctrl Pts',(-2.99758042112829,0.0430393547874399,
1.95671574855002));
#27856=CARTESIAN_POINT('Ctrl Pts',(-3.03458758682123,0.689006412056357,
1.9425072435811));
#27857=CARTESIAN_POINT('Ctrl Pts',(-3.07159475251418,1.32724333752614,1.57686059959224));
#27858=CARTESIAN_POINT('Ctrl Pts',(-3.10860191820712,1.66621740628167,1.02679523855085));
#27859=CARTESIAN_POINT('Ctrl Pts',(-3.14560908390006,2.00519147503719,0.476729877509469));
#27860=CARTESIAN_POINT('Ctrl Pts',(-3.18261624959301,2.04490268707848,-0.257754200584423));
#27861=CARTESIAN_POINT('Ctrl Pts',(-3.21962341528595,1.76721182581842,-0.841160668068887));
#27862=CARTESIAN_POINT('Ctrl Pts',(-3.25663058097889,1.48952096455835,-1.42456713555338));
#27863=CARTESIAN_POINT('Ctrl Pts',(-3.29363774667183,0.894428029996892,
-1.85689599242844));
#27864=CARTESIAN_POINT('Ctrl Pts',(-3.33064491236477,0.253758511702538,
-1.9406688343316));
#27865=CARTESIAN_POINT('Ctrl Pts',(-3.36765207805771,-0.386911006591771,
-2.02444167623475));
#27866=CARTESIAN_POINT('Ctrl Pts',(-3.40465924375065,-1.07315710861897,
-1.75965850316607));
#27867=CARTESIAN_POINT('Ctrl Pts',(-3.4416664094436,-1.49151752346787,-1.26726650079074));
#27868=CARTESIAN_POINT('Ctrl Pts',(-3.46782104225432,-1.78719169434882,
-0.919270868595652));
#27869=CARTESIAN_POINT('Ctrl Pts',(-3.49397567506504,-1.94906001076164,
-0.457587214428717));
#27870=CARTESIAN_POINT('Ctrl Pts',(-3.52013030787576,-1.95285875419799,
0.00168591294888436));
#27871=CARTESIAN_POINT('Ctrl Pts',(-3.62186969212424,-1.95266119647961,
0.00164306867381859));
#27872=CARTESIAN_POINT('Ctrl Pts',(-3.59613206755216,-1.94904494208819,
-0.450423120568937));
#27873=CARTESIAN_POINT('Ctrl Pts',(-3.57039444298008,-1.79274977675162,
-0.904745632987596));
#27874=CARTESIAN_POINT('Ctrl Pts',(-3.54465681840801,-1.50565349219501,
-1.250438408122));
#27875=CARTESIAN_POINT('Ctrl Pts',(-3.50764965271506,-1.09284850536878,
-1.74749709247825));
#27876=CARTESIAN_POINT('Ctrl Pts',(-3.47064248702212,-0.409618924760199,
-2.01996937609925));
#27877=CARTESIAN_POINT('Ctrl Pts',(-3.43363532132918,0.231950860004497,
-1.94339585509611));
#27878=CARTESIAN_POINT('Ctrl Pts',(-3.39662815563624,0.873520644769173,
-1.86682233409297));
#27879=CARTESIAN_POINT('Ctrl Pts',(-3.3596209899433,1.47343063368994,-1.44120300846573));
#27880=CARTESIAN_POINT('Ctrl Pts',(-3.32261382425036,1.75765501167821,-0.860951514885858));
#27881=CARTESIAN_POINT('Ctrl Pts',(-3.28560665855741,2.04187938966649,-0.280700021305966));
#27882=CARTESIAN_POINT('Ctrl Pts',(-3.24859949286447,2.0104181567222,0.454183640226572));
#27883=CARTESIAN_POINT('Ctrl Pts',(-3.21159232717153,1.67764211872612,1.00802062109485));
#27884=CARTESIAN_POINT('Ctrl Pts',(-3.17458516147858,1.34486608073004,1.56185760196311));
#27885=CARTESIAN_POINT('Ctrl Pts',(-3.13757799578564,0.710775237682206,
1.93464790216714));
#27886=CARTESIAN_POINT('Ctrl Pts',(-3.1005708300927,0.0650084742934215,
1.95610903308469));
#27887=CARTESIAN_POINT('Ctrl Pts',(-3.06356366439976,-0.580758289095362,
1.97757016400225));
#27888=CARTESIAN_POINT('Ctrl Pts',(-3.02655649870682,-1.23820097282508,
1.64770212563333));
#27889=CARTESIAN_POINT('Ctrl Pts',(-2.98954933301388,-1.6070140800778,1.11718145235604));
#27890=CARTESIAN_POINT('Ctrl Pts',(-2.96698945271733,-1.83184566054671,
0.79377157592061));
#27891=CARTESIAN_POINT('Ctrl Pts',(-2.94442957242078,-1.94941601300893,
0.395794677332603));
#27892=CARTESIAN_POINT('Ctrl Pts',(-2.92186969212423,-1.95142771007674,
-0.00108710473741568));
#27893=CARTESIAN_POINT('Origin',(-7.7,0.,0.));
#27894=CARTESIAN_POINT('',(-2.12013030787576,-1.95644854722993,-0.00106994229120638));
#27895=CARTESIAN_POINT('',(-2.22186969212423,-1.9565983335214,-0.000961690378010772));
#27896=CARTESIAN_POINT('',(-7.7,-1.954,-2.39295984553393E-16));
#27897=CARTESIAN_POINT('Ctrl Pts',(-2.12013030787576,-1.95644854722993,
-0.00106994229120638));
#27898=CARTESIAN_POINT('Ctrl Pts',(-2.15356351910935,-1.95259121241954,
0.583241937911522));
#27899=CARTESIAN_POINT('Ctrl Pts',(-2.18699673034293,-1.67351864357878,
1.17075110719598));
#27900=CARTESIAN_POINT('Ctrl Pts',(-2.22042994157651,-1.21616753078681,
1.53346843737484));
#27901=CARTESIAN_POINT('Ctrl Pts',(-2.25743710726946,-0.709926347650253,
1.93495964454155));
#27902=CARTESIAN_POINT('Ctrl Pts',(-2.2944442729624,0.0147459708435234,
2.06103051482065));
#27903=CARTESIAN_POINT('Ctrl Pts',(-2.33145143865534,0.626834902648891,
1.85409463186776));
#27904=CARTESIAN_POINT('Ctrl Pts',(-2.36845860434828,1.23892383445426,1.64715874891487));
#27905=CARTESIAN_POINT('Ctrl Pts',(-2.40546577004122,1.73842937957122,1.10721611272997));
#27906=CARTESIAN_POINT('Ctrl Pts',(-2.44247293573417,1.89718828178632,0.480900752167918));
#27907=CARTESIAN_POINT('Ctrl Pts',(-2.47948010142711,2.05594718400142,-0.145414608394115));
#27908=CARTESIAN_POINT('Ctrl Pts',(-2.51648726712005,1.87395944331467,-0.858102693333298));
#27909=CARTESIAN_POINT('Ctrl Pts',(-2.55349443281299,1.4343530975005,-1.33162310690643));
#27910=CARTESIAN_POINT('Ctrl Pts',(-2.59050159850593,0.994746751686315,
-1.80514352047958));
#27911=CARTESIAN_POINT('Ctrl Pts',(-2.62750876419887,0.297521800744686,
-2.03949626268667));
#27912=CARTESIAN_POINT('Ctrl Pts',(-2.66451592989182,-0.338844586481023,
-1.92763410739117));
#27913=CARTESIAN_POINT('Ctrl Pts',(-2.70152309558476,-0.975210973706731,
-1.81577195209567));
#27914=CARTESIAN_POINT('Ctrl Pts',(-2.7385302612777,-1.55071879721652,-1.35769489929758));
#27915=CARTESIAN_POINT('Ctrl Pts',(-2.77553742697064,-1.80248861895329,
-0.762642567579129));
#27916=CARTESIAN_POINT('Ctrl Pts',(-2.79040172060568,-1.90361445468435,
-0.523633920976263));
#27917=CARTESIAN_POINT('Ctrl Pts',(-2.80526601424072,-1.9525114258577,-0.262526962617265));
#27918=CARTESIAN_POINT('Ctrl Pts',(-2.82013030787576,-1.95130973680355,
-0.000989162390181431));
#27919=CARTESIAN_POINT('Ctrl Pts',(-2.92186969212423,-1.95142771007674,
-0.00108710473741568));
#27920=CARTESIAN_POINT('Ctrl Pts',(-2.90742240672784,-1.95271599535519,
-0.255249108206585));
#27921=CARTESIAN_POINT('Ctrl Pts',(-2.89297512133144,-1.90661267726525,
-0.508961994926469));
#27922=CARTESIAN_POINT('Ctrl Pts',(-2.87852783593505,-1.81093858213178,
-0.742354432122333));
#27923=CARTESIAN_POINT('Ctrl Pts',(-2.84152067024211,-1.56586644615734,
-1.34019633513771));
#27924=CARTESIAN_POINT('Ctrl Pts',(-2.80451350454917,-0.995538643432775,
-1.8047068329828));
#27925=CARTESIAN_POINT('Ctrl Pts',(-2.76750633885622,-0.360468490887422,
-1.92370764878637));
#27926=CARTESIAN_POINT('Ctrl Pts',(-2.73049917316328,0.274601661657948,
-2.04270846458994));
#27927=CARTESIAN_POINT('Ctrl Pts',(-2.69349200747034,0.974414164024119,
-1.81619959835197));
#27928=CARTESIAN_POINT('Ctrl Pts',(-2.6564848417774,1.41930990934805,-1.34764536592142));
#27929=CARTESIAN_POINT('Ctrl Pts',(-2.61947767608446,1.86420565467196,-0.879091133490892));
#27930=CARTESIAN_POINT('Ctrl Pts',(-2.58247051039151,2.05418464295365,-0.168491534867828));
#27931=CARTESIAN_POINT('Ctrl Pts',(-2.54546334469857,1.90246861029148,0.459567011909319));
#27932=CARTESIAN_POINT('Ctrl Pts',(-2.50845617900563,1.75075257762931,1.08762555868646));
#27933=CARTESIAN_POINT('Ctrl Pts',(-2.47144901331269,1.25734152402327,1.63314305361767));
#27934=CARTESIAN_POINT('Ctrl Pts',(-2.43444184761975,0.647614871484223,
1.84693898876838));
#27935=CARTESIAN_POINT('Ctrl Pts',(-2.39743468192681,0.0378882189451539,
2.06073492391911));
#27936=CARTESIAN_POINT('Ctrl Pts',(-2.36042751623386,-0.68815403252694,
1.94280929928931));
#27937=CARTESIAN_POINT('Ctrl Pts',(-2.32342035054092,-1.19887159918293,
1.54702797003394));
#27938=CARTESIAN_POINT('Ctrl Pts',(-2.28957013106869,-1.6660217144625,1.1850093012857));
#27939=CARTESIAN_POINT('Ctrl Pts',(-2.25571991159646,-1.95301731563171,
0.590518635644192));
#27940=CARTESIAN_POINT('Ctrl Pts',(-2.22186969212423,-1.9565983335214,-0.000961690378010772));
#27941=CARTESIAN_POINT('Origin',(-7.7,0.,0.));
#27942=CARTESIAN_POINT('',(-1.42013030787576,-1.95447741886037,0.00173992555780794));
#27943=CARTESIAN_POINT('',(-1.52186969212423,-1.95425590186397,0.00176118791910092));
#27944=CARTESIAN_POINT('',(-7.7,-1.954,-2.39295984553393E-16));
#27945=CARTESIAN_POINT('Ctrl Pts',(-1.42013030787576,-1.95447741886037,
0.00173992555780794));
#27946=CARTESIAN_POINT('Ctrl Pts',(-1.42784669259209,-1.95572105433507,
0.136952826586595));
#27947=CARTESIAN_POINT('Ctrl Pts',(-1.43556307730841,-1.94288272355423,
0.271931167846212));
#27948=CARTESIAN_POINT('Ctrl Pts',(-1.44327946202474,-1.915090057649,0.403756738132894));
#27949=CARTESIAN_POINT('Ctrl Pts',(-1.48028662771768,-1.78179864852216,
1.03598165971375));
#27950=CARTESIAN_POINT('Ctrl Pts',(-1.51729379341062,-1.30454480519379,
1.59569016586662));
#27951=CARTESIAN_POINT('Ctrl Pts',(-1.55430095910356,-0.701328365224583,
1.82721860873338));
#27952=CARTESIAN_POINT('Ctrl Pts',(-1.5913081247965,-0.098111925255361,
2.05874705160015));
#27953=CARTESIAN_POINT('Ctrl Pts',(-1.62831529048945,0.631067111354711,
1.96209543118079));
#27954=CARTESIAN_POINT('Ctrl Pts',(-1.66532245618239,1.15313600062339,1.58141262481102));
#27955=CARTESIAN_POINT('Ctrl Pts',(-1.70232962187533,1.67520488989206,1.20072981844126));
#27956=CARTESIAN_POINT('Ctrl Pts',(-1.73933678756827,1.99016363181935,0.536015826121098));
#27957=CARTESIAN_POINT('Ctrl Pts',(-1.77634395326121,1.95414574666676,-0.109102754469346));
#27958=CARTESIAN_POINT('Ctrl Pts',(-1.81335111895415,1.91812786151417,-0.754221335059817));
#27959=CARTESIAN_POINT('Ctrl Pts',(-1.8503582846471,1.53113334928168,-1.37974450392055));
#27960=CARTESIAN_POINT('Ctrl Pts',(-1.88736545034004,0.969932971601319,
-1.69994675904003));
#27961=CARTESIAN_POINT('Ctrl Pts',(-1.92437261603298,0.408732593920964,
-2.02014901415952));
#27962=CARTESIAN_POINT('Ctrl Pts',(-1.96137978172592,-0.326673649207257,
-2.03503035553774));
#27963=CARTESIAN_POINT('Ctrl Pts',(-1.99838694741886,-0.90036825696246,
-1.73779338639092));
#27964=CARTESIAN_POINT('Ctrl Pts',(-2.03539411311181,-1.47406286471766,
-1.4405564172441));
#27965=CARTESIAN_POINT('Ctrl Pts',(-2.07240127880475,-1.88604583709986,
-0.831201137572241));
#27966=CARTESIAN_POINT('Ctrl Pts',(-2.10940844449769,-1.94813229940127,
-0.188067725709169));
#27967=CARTESIAN_POINT('Ctrl Pts',(-2.11298239895705,-1.9541282784138,-0.125957334863212));
#27968=CARTESIAN_POINT('Ctrl Pts',(-2.11655635341641,-1.95686088988079,
-0.0635319066928876));
#27969=CARTESIAN_POINT('Ctrl Pts',(-2.12013030787576,-1.95644854722993,
-0.00106994229120638));
#27970=CARTESIAN_POINT('Ctrl Pts',(-2.22186969212423,-1.9565983335214,-0.000961690378010772));
#27971=CARTESIAN_POINT('Ctrl Pts',(-2.21871274590352,-1.95693230715789,
-0.056124451771436));
#27972=CARTESIAN_POINT('Ctrl Pts',(-2.21555579968281,-1.95480118623589,
-0.111261029713999));
#27973=CARTESIAN_POINT('Ctrl Pts',(-2.2123988534621,-1.95012120828141,-0.166180405709922));
#27974=CARTESIAN_POINT('Ctrl Pts',(-2.17539168776915,-1.89526036888401,
-0.809970418317528));
#27975=CARTESIAN_POINT('Ctrl Pts',(-2.13838452207621,-1.4901458082493,-1.42391340965182));
#27976=CARTESIAN_POINT('Ctrl Pts',(-2.10137735638327,-0.919825037899834,
-1.72757359987075));
#27977=CARTESIAN_POINT('Ctrl Pts',(-2.06437019069033,-0.349504267550385,
-2.03123379008967));
#27978=CARTESIAN_POINT('Ctrl Pts',(-2.02736302499739,0.386022712513811,
-2.02461117919323));
#27979=CARTESIAN_POINT('Ctrl Pts',(-1.99035585930445,0.950783209002053,
-1.7107308219266));
#27980=CARTESIAN_POINT('Ctrl Pts',(-1.9533486936115,1.51554370549031,-1.39685046465995));
#27981=CARTESIAN_POINT('Ctrl Pts',(-1.91634152791856,1.9095377184026,-0.775712361023085));
#27982=CARTESIAN_POINT('Ctrl Pts',(-1.87933436222562,1.95279734749102,-0.131038884865799));
#27983=CARTESIAN_POINT('Ctrl Pts',(-1.84232719653268,1.99605697657943,0.513634591291487));
#27984=CARTESIAN_POINT('Ctrl Pts',(-1.80532003083973,1.68858222184396,1.18184343996919));
#27985=CARTESIAN_POINT('Ctrl Pts',(-1.76831286514679,1.17082088687201,1.56836444964375));
#27986=CARTESIAN_POINT('Ctrl Pts',(-1.73130569945385,0.653059551900069,
1.9548854593183));
#27987=CARTESIAN_POINT('Ctrl Pts',(-1.69429853376091,-0.0749883633083459,
2.05971862998971));
#27988=CARTESIAN_POINT('Ctrl Pts',(-1.65729136806797,-0.680766493625946,
1.83497838636739));
#27989=CARTESIAN_POINT('Ctrl Pts',(-1.62028420237503,-1.28654462394356,
1.61023814274506));
#27990=CARTESIAN_POINT('Ctrl Pts',(-1.58327703668208,-1.77005296937036,
1.05592448482897));
#27991=CARTESIAN_POINT('Ctrl Pts',(-1.54626987098914,-1.91043532921589,
0.425235943498823));
#27992=CARTESIAN_POINT('Ctrl Pts',(-1.53813647803417,-1.94128840524023,
0.286623930317463));
#27993=CARTESIAN_POINT('Ctrl Pts',(-1.5300030850792,-1.95556755240123,0.144322800199925));
#27994=CARTESIAN_POINT('Ctrl Pts',(-1.52186969212423,-1.95425590186397,
0.00176118791910092));
#27995=CARTESIAN_POINT('Origin',(-7.7,0.,0.));
#27996=CARTESIAN_POINT('',(-0.720130307875768,-1.95080492165711,-0.000124213833098269));
#27997=CARTESIAN_POINT('',(-0.821869692124232,-1.95083908144908,-0.000261106490282405));
#27998=CARTESIAN_POINT('',(-7.7,-1.954,-2.39295984553393E-16));
#27999=CARTESIAN_POINT('Ctrl Pts',(-0.720130307875768,-1.95080492165711,
-0.000124213833098269));
#28000=CARTESIAN_POINT('Ctrl Pts',(-0.739137031767772,-1.95059134672475,
0.334498713882938));
#28001=CARTESIAN_POINT('Ctrl Pts',(-0.758143755659777,-1.86892145239226,
0.669217915359824));
#28002=CARTESIAN_POINT('Ctrl Pts',(-0.777150479551781,-1.70640146077838,
0.958534628557673));
#28003=CARTESIAN_POINT('Ctrl Pts',(-0.814157645244724,-1.38996585134649,
1.52185062156551));
#28004=CARTESIAN_POINT('Ctrl Pts',(-0.851164810937665,-0.767025170772472,
1.91304446051378));
#28005=CARTESIAN_POINT('Ctrl Pts',(-0.888171976630607,-0.122157367797084,
1.95338006990175));
#28006=CARTESIAN_POINT('Ctrl Pts',(-0.925179142323548,0.522710435178286,
1.99371567928973));
#28007=CARTESIAN_POINT('Ctrl Pts',(-0.96218630801649,1.18950536055502,1.68319305911744));
#28008=CARTESIAN_POINT('Ctrl Pts',(-0.999193473709431,1.57366693816335,
1.16367700557623));
#28009=CARTESIAN_POINT('Ctrl Pts',(-1.03620063940237,1.95782851577169,0.644160952035009));
#28010=CARTESIAN_POINT('Ctrl Pts',(-1.07320780509532,2.0593567456116,-0.084348534875133));
#28011=CARTESIAN_POINT('Ctrl Pts',(-1.11021497078826,1.83186684979789,-0.689097235990698));
#28012=CARTESIAN_POINT('Ctrl Pts',(-1.1472221364812,1.60437695398418,-1.29384593710626));
#28013=CARTESIAN_POINT('Ctrl Pts',(-1.18422930217414,1.04786893251684,-1.77483385242725));
#28014=CARTESIAN_POINT('Ctrl Pts',(-1.22123646786708,0.416548200503856,
-1.91234932504066));
#28015=CARTESIAN_POINT('Ctrl Pts',(-1.25824363356003,-0.214772531509113,
-2.04986479765406));
#28016=CARTESIAN_POINT('Ctrl Pts',(-1.29525079925297,-0.92090597406773,
-1.8439078275599));
#28017=CARTESIAN_POINT('Ctrl Pts',(-1.33225796494591,-1.37930820788441,
-1.38855867400841));
#28018=CARTESIAN_POINT('Ctrl Pts',(-1.36154874592253,-1.7421287367875,-1.0281546259051));
#28019=CARTESIAN_POINT('Ctrl Pts',(-1.39083952689915,-1.94975667778234,
-0.511517463082888));
#28020=CARTESIAN_POINT('Ctrl Pts',(-1.42013030787576,-1.95447741886037,
0.00173992555780794));
#28021=CARTESIAN_POINT('Ctrl Pts',(-1.52186969212423,-1.95425590186397,
0.00176118791910092));
#28022=CARTESIAN_POINT('Ctrl Pts',(-1.49299591938626,-1.94959950572841,
-0.50433652762779));
#28023=CARTESIAN_POINT('Ctrl Pts',(-1.46412214664829,-1.74845698196316,
-1.01371702142446));
#28024=CARTESIAN_POINT('Ctrl Pts',(-1.43524837391032,-1.39481355369076,
-1.37298340112569));
#28025=CARTESIAN_POINT('Ctrl Pts',(-1.39824120821737,-0.941553044055813,
-1.83345077967584));
#28026=CARTESIAN_POINT('Ctrl Pts',(-1.36123404252443,-0.237775650521653,
-2.04732211203193));
#28027=CARTESIAN_POINT('Ctrl Pts',(-1.32422687683149,0.39504888125557,-1.91690517402407));
#28028=CARTESIAN_POINT('Ctrl Pts',(-1.28721971113855,1.02787341303278,-1.78648823601621));
#28029=CARTESIAN_POINT('Ctrl Pts',(-1.25021254544561,1.58974508305305,-1.31178302764444));
#28030=CARTESIAN_POINT('Ctrl Pts',(-1.21320537975267,1.82401231951764,-0.70962541972142));
#28031=CARTESIAN_POINT('Ctrl Pts',(-1.17619821405972,2.05827955598223,-0.107467811798385));
#28032=CARTESIAN_POINT('Ctrl Pts',(-1.13919104836678,1.96494235889112,0.622142195675899));
#28033=CARTESIAN_POINT('Ctrl Pts',(-1.10218388267384,1.58663671031651,1.14593630401315));
#28034=CARTESIAN_POINT('Ctrl Pts',(-1.0651767169809,1.20833106174192,1.66973041235039));
#28035=CARTESIAN_POINT('Ctrl Pts',(-1.02816955128796,0.545056961683846,
1.9877086215506));
#28036=CARTESIAN_POINT('Ctrl Pts',(-0.991162385595016,-0.100219442561468,
1.95462225401688));
#28037=CARTESIAN_POINT('Ctrl Pts',(-0.954155219902073,-0.745495846806819,
1.92153588648315));
#28038=CARTESIAN_POINT('Ctrl Pts',(-0.91714805420913,-1.37277455523941,
1.53738494221546));
#28039=CARTESIAN_POINT('Ctrl Pts',(-0.880140888516187,-1.69552258335969,
0.977647214365655));
#28040=CARTESIAN_POINT('Ctrl Pts',(-0.860717156385535,-1.86492143156978,
0.683860984439727));
#28041=CARTESIAN_POINT('Ctrl Pts',(-0.841293424254884,-1.9504274654474,
0.341703702312491));
#28042=CARTESIAN_POINT('Ctrl Pts',(-0.821869692124232,-1.95083908144908,
-0.000261106490282405));
#28043=CARTESIAN_POINT('Origin',(-7.7,0.,0.));
#28044=CARTESIAN_POINT('',(-0.0201303078757663,-1.95230810266922,-4.45419903166711E-5));
#28045=CARTESIAN_POINT('',(-0.121869692124238,-1.95503470185946,-0.00140694303418273));
#28046=CARTESIAN_POINT('',(-7.7,-1.954,-2.39295984553393E-16));
#28047=CARTESIAN_POINT('Ctrl Pts',(-0.0201303078757663,-1.95230810266922,
-4.45419903166711E-5));
#28048=CARTESIAN_POINT('Ctrl Pts',(-0.0504273709434536,-1.94838732011207,
0.531290941650261));
#28049=CARTESIAN_POINT('Ctrl Pts',(-0.0807244340111409,-1.72620411445923,
1.06315610289758));
#28050=CARTESIAN_POINT('Ctrl Pts',(-0.111021497078828,-1.34149476870851,
1.42492350079784));
#28051=CARTESIAN_POINT('Ctrl Pts',(-0.148028662771771,-0.871581151338641,
1.86681405654212));
#28052=CARTESIAN_POINT('Ctrl Pts',(-0.185035828464712,-0.159177547940315,
2.0549177184817));
#28053=CARTESIAN_POINT('Ctrl Pts',(-0.222042994157654,0.468425641487877,
1.90068671820305));
#28054=CARTESIAN_POINT('Ctrl Pts',(-0.259050159850595,1.09602883091605,
1.74645571792442));
#28055=CARTESIAN_POINT('Ctrl Pts',(-0.296057325543536,1.63883160637408,
1.24989005542759));
#28056=CARTESIAN_POINT('Ctrl Pts',(-0.333064491236477,1.84974165646342,
0.639034692954403));
#28057=CARTESIAN_POINT('Ctrl Pts',(-0.37007165692942,2.06065170655277,0.0281793304812037));
#28058=CARTESIAN_POINT('Ctrl Pts',(-0.407078822622365,1.9396690312734,-0.696965731968384));
#28059=CARTESIAN_POINT('Ctrl Pts',(-0.444085988315308,1.54162814820921,
-1.20579510892095));
#28060=CARTESIAN_POINT('Ctrl Pts',(-0.48109315400825,1.14358726514503,-1.71462448587351));
#28061=CARTESIAN_POINT('Ctrl Pts',(-0.51810031970119,0.468488174296075,
-2.0071381773291));
#28062=CARTESIAN_POINT('Ctrl Pts',(-0.555107485394131,-0.175075909501228,
-1.9493959880236));
#28063=CARTESIAN_POINT('Ctrl Pts',(-0.592114651087072,-0.818639993298532,
-1.89165379871811));
#28064=CARTESIAN_POINT('Ctrl Pts',(-0.629121816780013,-1.43066907004416,
-1.48365572865153));
#28065=CARTESIAN_POINT('Ctrl Pts',(-0.666128982472954,-1.7317183392721,
-0.911937620084552));
#28066=CARTESIAN_POINT('Ctrl Pts',(-0.684129424273892,-1.87814997618576,
-0.633851515755706));
#28067=CARTESIAN_POINT('Ctrl Pts',(-0.70212986607483,-1.95100718918947,
-0.317031039535227));
#28068=CARTESIAN_POINT('Ctrl Pts',(-0.720130307875768,-1.95080492165711,
-0.000124213833098269));
#28069=CARTESIAN_POINT('Ctrl Pts',(-0.821869692124232,-1.95083908144908,
-0.000261106490282405));
#28070=CARTESIAN_POINT('Ctrl Pts',(-0.804286258561941,-1.95121169895482,
-0.309826511108712));
#28071=CARTESIAN_POINT('Ctrl Pts',(-0.78670282499965,-1.88185055673912,
-0.619234186361387));
#28072=CARTESIAN_POINT('Ctrl Pts',(-0.769119391437359,-1.7418642515495,
-0.892457536920604));
#28073=CARTESIAN_POINT('Ctrl Pts',(-0.732112225744419,-1.44724054381106,
-1.46750004892517));
#28074=CARTESIAN_POINT('Ctrl Pts',(-0.69510506005148,-0.839775780526202,
-1.8822605615025));
#28075=CARTESIAN_POINT('Ctrl Pts',(-0.65809789435854,-0.196925867416372,
-1.94726374474532));
#28076=CARTESIAN_POINT('Ctrl Pts',(-0.621090728665598,0.445924045693496,
-2.01226692798816));
#28077=CARTESIAN_POINT('Ctrl Pts',(-0.584083562972655,1.12415910862834,
-1.72751278189645));
#28078=CARTESIAN_POINT('Ctrl Pts',(-0.547076397279713,1.52793680192538,
-1.22311221086593));
#28079=CARTESIAN_POINT('Ctrl Pts',(-0.51006923158677,1.93171449522242,-0.718711639835416));
#28080=CARTESIAN_POINT('Ctrl Pts',(-0.473062065893828,2.06103481888165,
0.00533535613392075));
#28081=CARTESIAN_POINT('Ctrl Pts',(-0.436054900200886,1.8569022710431,0.618378693290504));
#28082=CARTESIAN_POINT('Ctrl Pts',(-0.399047734507945,1.65276972320455,
1.23142203044707));
#28083=CARTESIAN_POINT('Ctrl Pts',(-0.362040568815004,1.11518430386824,
1.73346170879089));
#28084=CARTESIAN_POINT('Ctrl Pts',(-0.325033403122063,0.489560150069195,
1.89502691947245));
#28085=CARTESIAN_POINT('Ctrl Pts',(-0.288026237429121,-0.136064003729868,
2.05659213015401));
#28086=CARTESIAN_POINT('Ctrl Pts',(-0.251019071736179,-0.849726891991672,
1.87768287317329));
#28087=CARTESIAN_POINT('Ctrl Pts',(-0.214011906043236,-1.32516987168342,
1.4403068683668));
#28088=CARTESIAN_POINT('Ctrl Pts',(-0.183297834736904,-1.7197634404401,
1.07730695881503));
#28089=CARTESIAN_POINT('Ctrl Pts',(-0.152583763430571,-1.95026736215908,
0.536271058584337));
#28090=CARTESIAN_POINT('Ctrl Pts',(-0.121869692124238,-1.95503470185946,
-0.00140694303418273));
#28091=CARTESIAN_POINT('Origin',(-16.9400562256037,0.,0.));
#28092=CARTESIAN_POINT('',(-0.490056225603702,-1.55295652796194,-9.88815851658073E-5));
#28093=CARTESIAN_POINT('',(-0.351943774396294,-1.55632368410563,-0.00112001017909952));
#28094=CARTESIAN_POINT('',(-16.9400562256037,-1.5555,-7.70311135908521E-14));
#28095=CARTESIAN_POINT('',(0.,0.4799292661563,1.47961081014119));
#28096=CARTESIAN_POINT('Ctrl Pts',(-0.490056225603702,-1.55295652796194,
-9.88815851658657E-5));
#28097=CARTESIAN_POINT('Ctrl Pts',(-0.472055783802765,-1.55311754492539,
-0.252375528145892));
#28098=CARTESIAN_POINT('Ctrl Pts',(-0.417048176308885,-1.37587923427884,
-1.0230984760672));
#28099=CARTESIAN_POINT('Ctrl Pts',(-0.325033403122065,-0.164474555116665,
-1.83065940731556));
#28100=CARTESIAN_POINT('Ctrl Pts',(-0.21401190604324,1.4477823064221,-1.13208461653888));
#28101=CARTESIAN_POINT('Ctrl Pts',(-0.105667438335883,1.72974363970491,
0.557933133189484));
#28102=CARTESIAN_POINT('Ctrl Pts',(-0.0343301363214699,0.933636559814803,
1.33261642798006));
#28103=CARTESIAN_POINT('Ctrl Pts',(1.07607065619186E-15,0.480182858679997,
1.4822056829043));
#28104=CARTESIAN_POINT('',(2.22044604925031E-15,1.55526325306019,0.0271378643346999));
#28105=CARTESIAN_POINT('Origin',(0.,0.,0.));
#28106=CARTESIAN_POINT('Ctrl Pts',(-0.351943774396294,-1.55632368410563,
-0.00112001017909957));
#28107=CARTESIAN_POINT('Ctrl Pts',(-0.345650680009688,-1.55710127006918,
-0.0888189981367454));
#28108=CARTESIAN_POINT('Ctrl Pts',(-0.302350419930139,-1.51054435461524,
-0.691468448221064));
#28109=CARTESIAN_POINT('Ctrl Pts',(-0.222042994157651,-0.72473494787801,
-1.69026698927826));
#28110=CARTESIAN_POINT('Ctrl Pts',(-0.111021497078823,1.0270020972766,-1.52351327282068));
#28111=CARTESIAN_POINT('Ctrl Pts',(-0.03700716569294,1.56427778786756,-0.489482550463674));
#28112=CARTESIAN_POINT('Ctrl Pts',(2.22044604925031E-15,1.55526325306019,
0.0271378643346999));
#28113=CARTESIAN_POINT('Origin',(-16.9400562256037,0.,0.));
#28114=CARTESIAN_POINT('',(-1.1900562256037,-1.55588005375502,0.00138508403538328));
#28115=CARTESIAN_POINT('',(-1.05194377439629,-1.55298372118426,-0.000207856267061268));
#28116=CARTESIAN_POINT('',(-16.9400562256037,-1.5555,-7.70311135908521E-14));
#28117=CARTESIAN_POINT('Ctrl Pts',(-1.1900562256037,-1.55588005375502,0.00138508403538323));
#28118=CARTESIAN_POINT('Ctrl Pts',(-1.16076544462708,-1.5521220636082,-0.407198267054996));
#28119=CARTESIAN_POINT('Ctrl Pts',(-1.09446749795752,-1.17801114814899,
-1.33809225472144));
#28120=CARTESIAN_POINT('Ctrl Pts',(-0.991162385595018,0.391152455034581,
-1.79576804489885));
#28121=CARTESIAN_POINT('Ctrl Pts',(-0.880140888516193,1.72019272226962,
-0.647083240986163));
#28122=CARTESIAN_POINT('Ctrl Pts',(-0.769119391437366,1.47772522761866,
1.09272715853592));
#28123=CARTESIAN_POINT('Ctrl Pts',(-0.658097894358541,-0.114699807832016,
1.83431047841002));
#28124=CARTESIAN_POINT('Ctrl Pts',(-0.565076839080654,-1.36118632868951,
1.05154277275593));
#28125=CARTESIAN_POINT('Ctrl Pts',(-0.509062949495707,-1.55278650963683,
0.266280833902191));
#28126=CARTESIAN_POINT('Ctrl Pts',(-0.490056225603702,-1.55295652796194,
-9.88815851658657E-5));
#28127=CARTESIAN_POINT('Ctrl Pts',(-1.05194377439629,-1.55298372118426,
-0.000207856267061286));
#28128=CARTESIAN_POINT('Ctrl Pts',(-1.034360340834,-1.5532803468394,-0.24664029581869));
#28129=CARTESIAN_POINT('Ctrl Pts',(-0.979769741578774,-1.38185467141502,
-1.01133963636197));
#28130=CARTESIAN_POINT('Ctrl Pts',(-0.888171976630605,-0.184933360961542,
-1.82856513855231));
#28131=CARTESIAN_POINT('Ctrl Pts',(-0.777150479551777,1.43481276042301,
-1.14852152405029));
#28132=CARTESIAN_POINT('Ctrl Pts',(-0.666128982472953,1.74365272478113,
0.580631652352415));
#28133=CARTESIAN_POINT('Ctrl Pts',(-0.555107485394127,0.459803001478689,
1.7795918156029));
#28134=CARTESIAN_POINT('Ctrl Pts',(-0.450379082701908,-1.14794220903712,
1.37654367374382));
#28135=CARTESIAN_POINT('Ctrl Pts',(-0.38265784570263,-1.55252859868912,
0.426903598581234));
#28136=CARTESIAN_POINT('Ctrl Pts',(-0.351943774396294,-1.55632368410563,
-0.00112001017909957));
#28137=CARTESIAN_POINT('Origin',(-16.9400562256037,0.,0.));
#28138=CARTESIAN_POINT('',(-1.8900562256037,-1.55744918895402,-0.000851737581328525));
#28139=CARTESIAN_POINT('',(-1.75194377439629,-1.55570371307544,0.00140201013713322));
#28140=CARTESIAN_POINT('',(-16.9400562256037,-1.5555,-7.70311135908521E-14));
#28141=CARTESIAN_POINT('Ctrl Pts',(-1.8900562256037,-1.55744918895402,-0.000851737581328577));
#28142=CARTESIAN_POINT('Ctrl Pts',(-1.88648227114434,-1.557777438183,-0.0505751693248516));
#28143=CARTESIAN_POINT('Ctrl Pts',(-1.84590115099204,-1.53307735824119,
-0.614838726303634));
#28144=CARTESIAN_POINT('Ctrl Pts',(-1.7683128651468,-0.845478645101226,
-1.63185140458178));
#28145=CARTESIAN_POINT('Ctrl Pts',(-1.65729136806797,0.910802436555798,
-1.59631211106002));
#28146=CARTESIAN_POINT('Ctrl Pts',(-1.54626987098914,1.83501425402401,-0.102451380513119));
#28147=CARTESIAN_POINT('Ctrl Pts',(-1.43524837391032,1.08283668534245,1.48500401619214));
#28148=CARTESIAN_POINT('Ctrl Pts',(-1.32422687683149,-0.658572718107321,
1.71582529904111));
#28149=CARTESIAN_POINT('Ctrl Pts',(-1.24249616072929,-1.49763533076483,
0.731798689168104));
#28150=CARTESIAN_POINT('Ctrl Pts',(-1.19777261032002,-1.5568700614218,0.109022580222819));
#28151=CARTESIAN_POINT('Ctrl Pts',(-1.1900562256037,-1.55588005375502,0.00138508403538323));
#28152=CARTESIAN_POINT('Ctrl Pts',(-1.75194377439629,-1.55570371307544,
0.00140201013713313));
#28153=CARTESIAN_POINT('Ctrl Pts',(-1.72307000165832,-1.55199694532266,
-0.401481816133661));
#28154=CARTESIAN_POINT('Ctrl Pts',(-1.65718906322741,-1.1866499045939,-1.32669967921838));
#28155=CARTESIAN_POINT('Ctrl Pts',(-1.55430095910356,0.370965051819814,
-1.80004421839588));
#28156=CARTESIAN_POINT('Ctrl Pts',(-1.44327946202473,1.71281466704483,-0.6663636376042));
#28157=CARTESIAN_POINT('Ctrl Pts',(-1.33225796494591,1.48990881738992,1.0760750010236));
#28158=CARTESIAN_POINT('Ctrl Pts',(-1.22123646786708,-0.0941078601541336,
1.83546359530854));
#28159=CARTESIAN_POINT('Ctrl Pts',(-1.12779840435054,-1.35490149413674,
1.06334259309671));
#28160=CARTESIAN_POINT('Ctrl Pts',(-1.07136750652695,-1.55265605041119,
0.272016432419122));
#28161=CARTESIAN_POINT('Ctrl Pts',(-1.05194377439629,-1.55298372118426,
-0.000207856267061286));
#28162=CARTESIAN_POINT('Origin',(-16.9400562256037,0.,0.));
#28163=CARTESIAN_POINT('',(-2.5900562256037,-1.55335839078706,-0.000787431984669446));
#28164=CARTESIAN_POINT('',(-2.45194377439629,-1.55756842773415,-0.000765562632226713));
#28165=CARTESIAN_POINT('',(-16.9400562256037,-1.5555,-7.70311135908521E-14));
#28166=CARTESIAN_POINT('Ctrl Pts',(-2.5900562256037,-1.55335839078706,-0.000787431984669417));
#28167=CARTESIAN_POINT('Ctrl Pts',(-2.57519193196866,-1.55431500661292,
-0.208987047262663));
#28168=CARTESIAN_POINT('Ctrl Pts',(-2.52332047264068,-1.41848003230292,
-0.934337843636373));
#28169=CARTESIAN_POINT('Ctrl Pts',(-2.43444184761975,-0.31818743609586,
-1.81011879586092));
#28170=CARTESIAN_POINT('Ctrl Pts',(-2.32342035054093,1.34690991987603,-1.25044271013452));
#28171=CARTESIAN_POINT('Ctrl Pts',(-2.2123988534621,1.78152905596337,0.45158336374919));
#28172=CARTESIAN_POINT('Ctrl Pts',(-2.10137735638328,0.588620854178164,
1.74106254069739));
#28173=CARTESIAN_POINT('Ctrl Pts',(-1.99392981376381,-1.08631350257498,
1.44967507269646));
#28174=CARTESIAN_POINT('Ctrl Pts',(-1.92348943683728,-1.5543785214527,0.464295206971033));
#28175=CARTESIAN_POINT('Ctrl Pts',(-1.8900562256037,-1.55744918895402,-0.000851737581328577));
#28176=CARTESIAN_POINT('Ctrl Pts',(-2.45194377439629,-1.55756842773415,
-0.0007655626322266));
#28177=CARTESIAN_POINT('Ctrl Pts',(-2.44878682817558,-1.55783429057528,
-0.0446783954609667));
#28178=CARTESIAN_POINT('Ctrl Pts',(-2.40862271626193,-1.53625065827796,
-0.603092332538515));
#28179=CARTESIAN_POINT('Ctrl Pts',(-2.33145143865534,-0.863749286419899,
-1.62225467335409));
#28180=CARTESIAN_POINT('Ctrl Pts',(-2.22042994157651,0.892820136543068,
-1.60643869907147));
#28181=CARTESIAN_POINT('Ctrl Pts',(-2.10940844449769,1.8337480082192,-0.123050285242695));
#28182=CARTESIAN_POINT('Ctrl Pts',(-1.99838694741886,1.09944353382152,1.47275145086502));
#28183=CARTESIAN_POINT('Ctrl Pts',(-1.88736545034003,-0.639264550272716,
1.72311173281902));
#28184=CARTESIAN_POINT('Ctrl Pts',(-1.80521772599918,-1.49366042548188,
0.74359750648739));
#28185=CARTESIAN_POINT('Ctrl Pts',(-1.76007716735126,-1.55674786476977,
0.114889516740449));
#28186=CARTESIAN_POINT('Ctrl Pts',(-1.75194377439629,-1.55570371307544,
0.00140201013713313));
#28187=CARTESIAN_POINT('Origin',(-16.9400562256037,0.,0.));
#28188=CARTESIAN_POINT('',(-3.29005622560369,-1.55459150059108,0.00134208679213341));
#28189=CARTESIAN_POINT('',(-3.15194377439629,-1.55345230451605,-0.000865399907588604));
#28190=CARTESIAN_POINT('',(-16.9400562256037,-1.5555,-7.70311135908521E-14));
#28191=CARTESIAN_POINT('Ctrl Pts',(-3.29005622560369,-1.55459150059108,
0.00134208679213352));
#28192=CARTESIAN_POINT('Ctrl Pts',(-3.26390159279297,-1.55156747530179,
-0.364266587535299));
#28193=CARTESIAN_POINT('Ctrl Pts',(-3.20073979428931,-1.24038640780706,
-1.25182269198089));
#28194=CARTESIAN_POINT('Ctrl Pts',(-3.1005708300927,0.238288506115619,-1.82235888080426));
#28195=CARTESIAN_POINT('Ctrl Pts',(-2.98954933301389,1.65947641764626,-0.789880574454531));
#28196=CARTESIAN_POINT('Ctrl Pts',(-2.87852783593505,1.5646389708752,0.964198212866461));
#28197=CARTESIAN_POINT('Ctrl Pts',(-2.76750633885623,0.0404155252740006,
1.83742751899441));
#28198=CARTESIAN_POINT('Ctrl Pts',(-2.67134913541244,-1.31171330547879,
1.13989061901984));
#28199=CARTESIAN_POINT('Ctrl Pts',(-2.6121990976616,-1.55193335019243,0.309361005391319));
#28200=CARTESIAN_POINT('Ctrl Pts',(-2.5900562256037,-1.55335839078706,-0.000787431984669417));
#28201=CARTESIAN_POINT('Ctrl Pts',(-3.15194377439629,-1.55345230451605,
-0.000865399907588483));
#28202=CARTESIAN_POINT('Ctrl Pts',(-3.1374964889999,-1.55447785607725,-0.203193443099082));
#28203=CARTESIAN_POINT('Ctrl Pts',(-3.08604203791056,-1.4237661941345,-0.922517657784447));
#28204=CARTESIAN_POINT('Ctrl Pts',(-2.99758042112829,-0.338493072017185,
-1.8064317083433));
#28205=CARTESIAN_POINT('Ctrl Pts',(-2.88655892404946,1.33278381758959,-1.26548819539577));
#28206=CARTESIAN_POINT('Ctrl Pts',(-2.77553742697064,1.78648747614462,0.431550201213581));
#28207=CARTESIAN_POINT('Ctrl Pts',(-2.66451592989181,0.608134005493306,
1.73434313370923));
#28208=CARTESIAN_POINT('Ctrl Pts',(-2.5566513790337,-1.07647945219465,1.46072394163763));
#28209=CARTESIAN_POINT('Ctrl Pts',(-2.48579399386852,-1.55471772490545,
0.470087890350195));
#28210=CARTESIAN_POINT('Ctrl Pts',(-2.45194377439629,-1.55756842773415,
-0.0007655626322266));
#28211=CARTESIAN_POINT('Origin',(-16.9400562256037,0.,0.));
#28212=CARTESIAN_POINT('',(-3.9900562256037,-1.55802831486089,-0.000113059531867663));
#28213=CARTESIAN_POINT('',(-3.85194377439629,-1.55443423291916,0.00130798020558064));
#28214=CARTESIAN_POINT('',(-16.9400562256037,-1.5555,-7.70311135908521E-14));
#28215=CARTESIAN_POINT('Ctrl Pts',(-3.9900562256037,-1.55802831486089,-0.000113059531867614));
#28216=CARTESIAN_POINT('Ctrl Pts',(-3.98961841931024,-1.55803469606833,
-0.00619811891591143));
#28217=CARTESIAN_POINT('Ctrl Pts',(-3.95217344732383,-1.55524873298545,
-0.526638897489874));
#28218=CARTESIAN_POINT('Ctrl Pts',(-3.87772130964449,-0.980111674806025,
-1.55472004153636));
#28219=CARTESIAN_POINT('Ctrl Pts',(-3.76669981256566,0.772908208897534,
-1.66744901069363));
#28220=CARTESIAN_POINT('Ctrl Pts',(-3.65567831548684,1.81983282548855,-0.256869207804794));
#28221=CARTESIAN_POINT('Ctrl Pts',(-3.54465681840801,1.20423745559398,1.38837511256683));
#28222=CARTESIAN_POINT('Ctrl Pts',(-3.43363532132918,-0.511496789897079,
1.76526041607566));
#28223=CARTESIAN_POINT('Ctrl Pts',(-3.34876845706108,-1.46583715960521,
0.820607790786356));
#28224=CARTESIAN_POINT('Ctrl Pts',(-3.30090875848592,-1.5558462814984,0.153046765228203));
#28225=CARTESIAN_POINT('Ctrl Pts',(-3.29005622560369,-1.55459150059108,
0.00134208679213352));
#28226=CARTESIAN_POINT('Ctrl Pts',(-3.85194377439629,-1.55443423291916,
0.00130798020558057));
#28227=CARTESIAN_POINT('Ctrl Pts',(-3.82620614982422,-1.55155547974314,
-0.358563543523688));
#28228=CARTESIAN_POINT('Ctrl Pts',(-3.7634613595592,-1.24823606413057,-1.24025965145944));
#28229=CARTESIAN_POINT('Ctrl Pts',(-3.66370940360124,0.217810325062528,
-1.82491965286328));
#28230=CARTESIAN_POINT('Ctrl Pts',(-3.55268790652242,1.65050222030251,-0.808464902075287));
#28231=CARTESIAN_POINT('Ctrl Pts',(-3.4416664094436,1.57536719290506,0.946568161661344));
#28232=CARTESIAN_POINT('Ctrl Pts',(-3.33064491236476,0.0610453305290268,
1.83685779108923));
#28233=CARTESIAN_POINT('Ctrl Pts',(-3.23407070068233,-1.30472822637037,
1.15158886161436));
#28234=CARTESIAN_POINT('Ctrl Pts',(-3.17450365469284,-1.5518508742249,0.315076059667656));
#28235=CARTESIAN_POINT('Ctrl Pts',(-3.15194377439629,-1.55345230451605,
-0.000865399907588483));
#28236=CARTESIAN_POINT('Origin',(-16.9400562256037,0.,0.));
#28237=CARTESIAN_POINT('',(-4.6900562256037,-1.55426764476375,-0.00126339721357951));
#28238=CARTESIAN_POINT('',(-4.55194377439629,-1.55803858294675,-5.37804637934514E-6));
#28239=CARTESIAN_POINT('',(-16.9400562256037,-1.5555,-7.70311135908521E-14));
#28240=CARTESIAN_POINT('Ctrl Pts',(-4.6900562256037,-1.55426764476375,-0.00126339721357914));
#28241=CARTESIAN_POINT('Ctrl Pts',(-4.67832808013455,-1.55552512007785,
-0.165294437232494));
#28242=CARTESIAN_POINT('Ctrl Pts',(-4.62959276897247,-1.45615629828598,
-0.845427058906527));
#28243=CARTESIAN_POINT('Ctrl Pts',(-4.54385029211744,-0.469736383593091,
-1.77682892608546));
#28244=CARTESIAN_POINT('Ctrl Pts',(-4.43282879503861,1.2366354145067,-1.35959779134602));
#28245=CARTESIAN_POINT('Ctrl Pts',(-4.32180729795979,1.8132709732004,0.299702653298089));
#28246=CARTESIAN_POINT('Ctrl Pts',(-4.21078580088097,0.733381167783709,
1.68520781074188));
#28247=CARTESIAN_POINT('Ctrl Pts',(-4.1002021100956,-1.00959320041139,1.53178792699158));
#28248=CARTESIAN_POINT('Ctrl Pts',(-4.02662558500318,-1.55749530135286,
0.50816360735401));
#28249=CARTESIAN_POINT('Ctrl Pts',(-3.9900562256037,-1.55802831486089,-0.000113059531867614));
#28250=CARTESIAN_POINT('Ctrl Pts',(-4.55194377439629,-1.55803858294675,
-5.37804637950411E-6));
#28251=CARTESIAN_POINT('Ctrl Pts',(-4.55192297634147,-1.55803859780055,
-0.000294444541598174));
#28252=CARTESIAN_POINT('Ctrl Pts',(-4.51489501259372,-1.55790772834933,
-0.514936006620134));
#28253=CARTESIAN_POINT('Ctrl Pts',(-4.44085988315302,-0.997507700137877,
-1.5436163594892));
#28254=CARTESIAN_POINT('Ctrl Pts',(-4.3298383860742,0.754135777011385,-1.67602276444812));
#28255=CARTESIAN_POINT('Ctrl Pts',(-4.21881688899538,1.81683366297973,-0.277287789454163));
#28256=CARTESIAN_POINT('Ctrl Pts',(-4.10779539191654,1.21975146666773,1.37476522965911));
#28257=CARTESIAN_POINT('Ctrl Pts',(-3.99677389483772,-0.491642529871626,
1.77089262800929));
#28258=CARTESIAN_POINT('Ctrl Pts',(-3.91149002233097,-1.46127128776662,
0.832427049795263));
#28259=CARTESIAN_POINT('Ctrl Pts',(-3.86321331551716,-1.55569473103557,
0.158882231999483));
#28260=CARTESIAN_POINT('Ctrl Pts',(-3.85194377439629,-1.55443423291916,
0.00130798020558057));
#28261=CARTESIAN_POINT('Origin',(-16.9400562256037,0.,0.));
#28262=CARTESIAN_POINT('',(-5.3900562256037,-1.55356607152694,0.000946640642580529));
#28263=CARTESIAN_POINT('',(-5.25194377439629,-1.55441883725758,-0.00130423800998869));
#28264=CARTESIAN_POINT('',(-16.9400562256037,-1.5555,-7.70311135908521E-14));
#28265=CARTESIAN_POINT('Ctrl Pts',(-5.3900562256037,-1.55356607152694,0.000946640642580637));
#28266=CARTESIAN_POINT('Ctrl Pts',(-5.36703774095887,-1.55177070227827,
-0.321358232211269));
#28267=CARTESIAN_POINT('Ctrl Pts',(-5.30701209062111,-1.29693323687991,
-1.16443930671404));
#28268=CARTESIAN_POINT('Ctrl Pts',(-5.20997927459039,0.0837239529942017,
-1.83596394363836));
#28269=CARTESIAN_POINT('Ctrl Pts',(-5.09895777751157,1.58693624990787,-0.927041876817589));
#28270=CARTESIAN_POINT('Ctrl Pts',(-4.98793628043274,1.64039272540732,0.828785261135749));
#28271=CARTESIAN_POINT('Ctrl Pts',(-4.87691478335392,0.195257872362318,
1.82747029139345));
#28272=CARTESIAN_POINT('Ctrl Pts',(-4.77762143174423,-1.25675047370399,
1.22752168128547));
#28273=CARTESIAN_POINT('Ctrl Pts',(-4.71533524582749,-1.55155726365705,
0.352291560718858));
#28274=CARTESIAN_POINT('Ctrl Pts',(-4.6900562256037,-1.55426764476375,-0.00126339721357914));
#28275=CARTESIAN_POINT('Ctrl Pts',(-5.25194377439629,-1.55441883725758,
-0.00130423800998841));
#28276=CARTESIAN_POINT('Ctrl Pts',(-5.2406326371658,-1.55567946829412,-0.159464061065563));
#28277=CARTESIAN_POINT('Ctrl Pts',(-5.19231433424236,-1.46081140823039,
-0.833606098981985));
#28278=CARTESIAN_POINT('Ctrl Pts',(-5.10698886562598,-0.489658649608892,
-1.77144220452719));
#28279=CARTESIAN_POINT('Ctrl Pts',(-4.99596736854715,1.22129057217261,-1.37339812706995));
#28280=CARTESIAN_POINT('Ctrl Pts',(-4.88494587146833,1.81652193399072,0.279322645783608));
#28281=CARTESIAN_POINT('Ctrl Pts',(-4.77392437438949,0.752257995551791,
1.67686641842616));
#28282=CARTESIAN_POINT('Ctrl Pts',(-4.66292367536549,-0.998907961074514,
1.54252325729719));
#28283=CARTESIAN_POINT('Ctrl Pts',(-4.58893014203442,-1.55801216758575,
0.514058064897643));
#28284=CARTESIAN_POINT('Ctrl Pts',(-4.55194377439629,-1.55803858294675,
-5.37804637950411E-6));
#28285=CARTESIAN_POINT('Origin',(-16.9400562256037,0.,0.));
#28286=CARTESIAN_POINT('',(-6.0900562256037,-1.55768689774605,0.000665455443045115));
#28287=CARTESIAN_POINT('',(-5.95194377439629,-1.55346217675642,0.000872969649942032));
#28288=CARTESIAN_POINT('',(-16.9400562256037,-1.5555,-7.70311135908521E-14));
#28289=CARTESIAN_POINT('Ctrl Pts',(-6.0900562256037,-1.55768689774605,0.000665455443045072));
#28290=CARTESIAN_POINT('Ctrl Pts',(-6.05574740178319,-1.5551166351628,-0.476471113420595));
#28291=CARTESIAN_POINT('Ctrl Pts',(-5.98443141226975,-1.06553522999869,
-1.47283120294195));
#28292=CARTESIAN_POINT('Ctrl Pts',(-5.87610825706334,0.629504981698008,
-1.72670112661761));
#28293=CARTESIAN_POINT('Ctrl Pts',(-5.76508675998453,1.79168050778642,-0.409456054617966));
#28294=CARTESIAN_POINT('Ctrl Pts',(-5.65406526290569,1.31705477835589,1.28185023050864));
#28295=CARTESIAN_POINT('Ctrl Pts',(-5.54304376582688,-0.360774817741443,
1.80211399015954));
#28296=CARTESIAN_POINT('Ctrl Pts',(-5.45504075339287,-1.42948053097645,
0.909516853134372));
#28297=CARTESIAN_POINT('Ctrl Pts',(-5.40404490665181,-1.55465714455676,
0.196816183584846));
#28298=CARTESIAN_POINT('Ctrl Pts',(-5.3900562256037,-1.55356607152694,0.000946640642580637));
#28299=CARTESIAN_POINT('Ctrl Pts',(-5.95194377439629,-1.55346217675642,
0.000872969649942171));
#28300=CARTESIAN_POINT('Ctrl Pts',(-5.92934229799011,-1.55184313839371,
-0.315645984838267));
#28301=CARTESIAN_POINT('Ctrl Pts',(-5.86973365589099,-1.30402610796483,
-1.15275506404449));
#28302=CARTESIAN_POINT('Ctrl Pts',(-5.77311784809893,0.0631027514921653,
-1.83678826212252));
#28303=CARTESIAN_POINT('Ctrl Pts',(-5.6620963510201,1.57642645299097,-0.944803003502463));
#28304=CARTESIAN_POINT('Ctrl Pts',(-5.55107485394128,1.64959562566877,0.810313117807789));
#28305=CARTESIAN_POINT('Ctrl Pts',(-5.44005335686245,0.215766101057041,
1.82516247680901));
#28306=CARTESIAN_POINT('Ctrl Pts',(-5.34034299701413,-1.24901343126791,
1.23910521287792));
#28307=CARTESIAN_POINT('Ctrl Pts',(-5.27763980285874,-1.5515550039988,0.357994675267643));
#28308=CARTESIAN_POINT('Ctrl Pts',(-5.25194377439629,-1.55441883725758,
-0.00130423800998841));
#28309=CARTESIAN_POINT('Origin',(-16.9400562256037,0.,0.));
#28310=CARTESIAN_POINT('',(-6.7900562256037,-1.55551006981711,-0.00141244968499829));
#28311=CARTESIAN_POINT('',(-6.65194377439629,-1.55757973858287,0.000756704723131347));
#28312=CARTESIAN_POINT('',(-16.9400562256037,-1.5555,-7.70311135908521E-14));
#28313=CARTESIAN_POINT('Ctrl Pts',(-6.7900562256037,-1.55551006981711,-0.00141244968499835));
#28314=CARTESIAN_POINT('Ctrl Pts',(-6.78146422830045,-1.55660813262382,
-0.121337247012077));
#28315=CARTESIAN_POINT('Ctrl Pts',(-6.73586506530426,-1.48920084493374,
-0.756577051035784));
#28316=CARTESIAN_POINT('Ctrl Pts',(-6.65325873661513,-0.617937253968403,
-1.73087459187634));
#28317=CARTESIAN_POINT('Ctrl Pts',(-6.5422372395363,1.11754670885474,-1.45906225232958));
#28318=CARTESIAN_POINT('Ctrl Pts',(-6.43121574245748,1.83208868553414,0.145685795405434));
#28319=CARTESIAN_POINT('Ctrl Pts',(-6.32019424537864,0.872914255927876,
1.6173416474088));
#28320=CARTESIAN_POINT('Ctrl Pts',(-6.20917274829983,-0.883716608491293,
1.61146463148335));
#28321=CARTESIAN_POINT('Ctrl Pts',(-6.13246007504151,-1.53965976377384,
0.590180722825843));
#28322=CARTESIAN_POINT('Ctrl Pts',(-6.09275456747613,-1.55788904536813,
0.0381915912665651));
#28323=CARTESIAN_POINT('Ctrl Pts',(-6.0900562256037,-1.55768689774605,0.000665455443045072));
#28324=CARTESIAN_POINT('Ctrl Pts',(-6.65194377439629,-1.55757973858287,
0.000756704723131364));
#28325=CARTESIAN_POINT('Ctrl Pts',(-6.61805195881443,-1.55475278059858,
-0.470666295640637));
#28326=CARTESIAN_POINT('Ctrl Pts',(-6.54715297753963,-1.07549238527194,
-1.4618239969165));
#28327=CARTESIAN_POINT('Ctrl Pts',(-6.43924683057189,0.610076257496618,
-1.73366087720635));
#28328=CARTESIAN_POINT('Ctrl Pts',(-6.32822533349305,1.78696973330201,-0.429548890557871));
#28329=CARTESIAN_POINT('Ctrl Pts',(-6.21720383641424,1.3313655119277,1.26698024876731));
#28330=CARTESIAN_POINT('Ctrl Pts',(-6.10618233933541,-0.340516238842866,
1.80605143010969));
#28331=CARTESIAN_POINT('Ctrl Pts',(-6.01776231866276,-1.42428876297189,
0.92133852484065));
#28332=CARTESIAN_POINT('Ctrl Pts',(-5.96634946368305,-1.55449411658094,
0.202615264258711));
#28333=CARTESIAN_POINT('Ctrl Pts',(-5.95194377439629,-1.55346217675642,
0.000872969649942171));
#28334=CARTESIAN_POINT('Origin',(-16.9400562256037,0.,0.));
#28335=CARTESIAN_POINT('',(-7.4900562256037,-1.5530180908049,0.000313254609165155));
#28336=CARTESIAN_POINT('',(-7.3519437743963,-1.55568612057705,-0.00140331110564815));
#28337=CARTESIAN_POINT('',(-16.9400562256037,-1.5555,-7.70311135908521E-14));
#28338=CARTESIAN_POINT('Ctrl Pts',(-7.4900562256037,-1.5530180908049,0.000313254609165155));
#28339=CARTESIAN_POINT('Ctrl Pts',(-7.47017388912477,-1.55251547593583,
-0.278325135901937));
#28340=CARTESIAN_POINT('Ctrl Pts',(-7.4132843869529,-1.34789754076425,-1.07628426120452));
#28341=CARTESIAN_POINT('Ctrl Pts',(-7.31938771908807,-0.0714373480345857,
-1.8364830540876));
#28342=CARTESIAN_POINT('Ctrl Pts',(-7.20836622200926,1.50308509085693,-1.05759562796407));
#28343=CARTESIAN_POINT('Ctrl Pts',(-7.09734472493043,1.70445447418163,0.687465088631667));
#28344=CARTESIAN_POINT('Ctrl Pts',(-6.9863232278516,0.348708506197304,1.80448765037358));
#28345=CARTESIAN_POINT('Ctrl Pts',(-6.88389372807603,-1.19602678497936,
1.31414025780625));
#28346=CARTESIAN_POINT('Ctrl Pts',(-6.81847139399339,-1.55187859293768,
0.39519886080267));
#28347=CARTESIAN_POINT('Ctrl Pts',(-6.7900562256037,-1.55551006981711,-0.00141244968499835));
#28348=CARTESIAN_POINT('Ctrl Pts',(-7.3519437743963,-1.55568612057705,-0.00140331110564832));
#28349=CARTESIAN_POINT('Ctrl Pts',(-7.3437687853317,-1.55673540772934,-0.115474538019075));
#28350=CARTESIAN_POINT('Ctrl Pts',(-7.29858663057415,-1.49325970695437,
-0.744774653469687));
#28351=CARTESIAN_POINT('Ctrl Pts',(-7.21639731012365,-0.637334153250706,
-1.723826631137));
#28352=CARTESIAN_POINT('Ctrl Pts',(-7.10537581304485,1.10109249863036,-1.47151907448626));
#28353=CARTESIAN_POINT('Ctrl Pts',(-6.994354315966,1.83360901398418,0.125104200380868));
#28354=CARTESIAN_POINT('Ctrl Pts',(-6.8833328188872,0.891020217215038,1.60743772807255));
#28355=CARTESIAN_POINT('Ctrl Pts',(-6.77231132180836,-0.865565831794229,
1.62128617706663));
#28356=CARTESIAN_POINT('Ctrl Pts',(-6.69518164031139,-1.53656334674878,
0.601920948524818));
#28357=CARTESIAN_POINT('Ctrl Pts',(-6.65505912450737,-1.55783959376381,
0.0440901075324884));
#28358=CARTESIAN_POINT('Ctrl Pts',(-6.65194377439629,-1.55757973858287,
0.000756704723131364));
#28359=CARTESIAN_POINT('Origin',(-16.9400562256037,0.,0.));
#28360=CARTESIAN_POINT('',(-8.1900562256037,-1.55665418971026,0.00122204596489902));
#28361=CARTESIAN_POINT('',(-8.05194377439629,-1.55298816336082,0.000219416486716834));
#28362=CARTESIAN_POINT('',(-16.9400562256037,-1.5555,-7.70311135908521E-14));
#28363=CARTESIAN_POINT('Ctrl Pts',(-8.1900562256037,-1.55665418971026,0.00122204596489912));
#28364=CARTESIAN_POINT('Ctrl Pts',(-8.15888354994909,-1.5529084750837,-0.433054190629925));
#28365=CARTESIAN_POINT('Ctrl Pts',(-8.09070370860153,-1.1376911274873,-1.38916802661491));
#28366=CARTESIAN_POINT('Ctrl Pts',(-7.98551670156104,0.481614916815858,
-1.77364606800387));
#28367=CARTESIAN_POINT('Ctrl Pts',(-7.87449520448221,1.75075787078272,-0.559124476782657));
#28368=CARTESIAN_POINT('Ctrl Pts',(-7.76347370740338,1.42048470756065,1.16618887759722));
#28369=CARTESIAN_POINT('Ctrl Pts',(-7.65245221032457,-0.207481399618984,
1.82612287961606));
#28370=CARTESIAN_POINT('Ctrl Pts',(-7.56131304972465,-1.3883013990334,0.998368235695849));
#28371=CARTESIAN_POINT('Ctrl Pts',(-7.50718105481771,-1.55345099736004,
0.240306922105225));
#28372=CARTESIAN_POINT('Ctrl Pts',(-7.4900562256037,-1.5530180908049,0.000313254609165155));
#28373=CARTESIAN_POINT('Ctrl Pts',(-8.05194377439629,-1.55298816336082,
0.00021941648671699));
#28374=CARTESIAN_POINT('Ctrl Pts',(-8.03247844615601,-1.55264386792659,
-0.272587956900562));
#28375=CARTESIAN_POINT('Ctrl Pts',(-7.97600595222279,-1.35426737168086,
-1.06452050752492));
#28376=CARTESIAN_POINT('Ctrl Pts',(-7.88252629259662,-0.0920545910400277,
-1.83556504362701));
#28377=CARTESIAN_POINT('Ctrl Pts',(-7.77150479551779,1.49111460364442,-1.07440696010184));
#28378=CARTESIAN_POINT('Ctrl Pts',(-7.66048329843897,1.71206645837288,0.668282514533717));
#28379=CARTESIAN_POINT('Ctrl Pts',(-7.54946180136013,0.368948984659062,
1.80045819830287));
#28380=CARTESIAN_POINT('Ctrl Pts',(-7.44661529334591,-1.18750584841491,
1.32556192353867));
#28381=CARTESIAN_POINT('Ctrl Pts',(-7.38077595102464,-1.55198541440245,
0.40091181575136));
#28382=CARTESIAN_POINT('Ctrl Pts',(-7.3519437743963,-1.55568612057705,-0.00140331110564832));
#28383=CARTESIAN_POINT('Origin',(-16.9400562256037,0.,0.));
#28384=CARTESIAN_POINT('',(-8.8900562256037,-1.55680109303704,-0.00117256108906006));
#28385=CARTESIAN_POINT('',(-8.7519437743963,-1.55648790187904,0.0012702340526393));
#28386=CARTESIAN_POINT('',(-16.9400562256037,-1.5555,-7.70311135908521E-14));
#28387=CARTESIAN_POINT('Ctrl Pts',(-8.8900562256037,-1.55680109303704,-0.00117256108905984));
#28388=CARTESIAN_POINT('Ctrl Pts',(-8.88460037646635,-1.5574388429621,-0.0771610424262627));
#28389=CARTESIAN_POINT('Ctrl Pts',(-8.84213736163605,-1.51787106717481,
-0.667914644327412));
#28390=CARTESIAN_POINT('Ctrl Pts',(-8.7626671811128,-0.761733736392313,
-1.67258333648488));
#28391=CARTESIAN_POINT('Ctrl Pts',(-8.651645684034,0.990492616380764,-1.54812715225214));
#28392=CARTESIAN_POINT('Ctrl Pts',(-8.54062418695516,1.83784806665277,-0.00936944746539623));
#28393=CARTESIAN_POINT('Ctrl Pts',(-8.42960268987634,1.00622559096247,1.53794777633616));
#28394=CARTESIAN_POINT('Ctrl Pts',(-8.31858119279751,-0.744640747383609,
1.68026291394564));
#28395=CARTESIAN_POINT('Ctrl Pts',(-8.2387323713733,-1.51463350220016,0.678606070894573));
#28396=CARTESIAN_POINT('Ctrl Pts',(-8.19589071564203,-1.55735526314127,
0.0825041407189418));
#28397=CARTESIAN_POINT('Ctrl Pts',(-8.1900562256037,-1.55665418971026,0.00122204596489912));
#28398=CARTESIAN_POINT('Ctrl Pts',(-8.7519437743963,-1.55648790187904,0.00127023405263929));
#28399=CARTESIAN_POINT('Ctrl Pts',(-8.72118810698033,-1.55270169329837,
-0.427315239145853));
#28400=CARTESIAN_POINT('Ctrl Pts',(-8.65342527387141,-1.14681610862558,
-1.37790157034533));
#28401=CARTESIAN_POINT('Ctrl Pts',(-8.54865527506958,0.461668379793908,
-1.77894220935235));
#28402=CARTESIAN_POINT('Ctrl Pts',(-8.43763377799074,1.74436906067446,-0.578748354018101));
#28403=CARTESIAN_POINT('Ctrl Pts',(-8.32661228091193,1.43349016294594,1.15016478378281));
#28404=CARTESIAN_POINT('Ctrl Pts',(-8.21559078383309,-0.186962896184165,
1.82833748322551));
#28405=CARTESIAN_POINT('Ctrl Pts',(-8.12403461499455,-1.38244825556081,
1.01016791192593));
#28406=CARTESIAN_POINT('Ctrl Pts',(-8.06948561184895,-1.55329843681054,
0.246068987620239));
#28407=CARTESIAN_POINT('Ctrl Pts',(-8.05194377439629,-1.55298816336082,
0.00021941648671699));
#28408=CARTESIAN_POINT('Origin',(-16.9400562256037,0.,0.));
#28409=CARTESIAN_POINT('',(-9.5900562256037,-1.55305431186606,-0.000397270594051011));
#28410=CARTESIAN_POINT('',(-9.45194377439629,-1.55695751420806,-0.00111193227041603));
#28411=CARTESIAN_POINT('',(-16.9400562256037,-1.5555,-7.70311135908521E-14));
#28412=CARTESIAN_POINT('Ctrl Pts',(-9.5900562256037,-1.55305431186606,-0.000397270594050692));
#28413=CARTESIAN_POINT('Ctrl Pts',(-9.57331003729067,-1.5535918950784,-0.235070859271372));
#28414=CARTESIAN_POINT('Ctrl Pts',(-9.51955668328469,-1.39353800000331,
-0.98765021615145));
#28415=CARTESIAN_POINT('Ctrl Pts',(-9.42879616358577,-0.226089474720918,
-1.82391251217418));
#28416=CARTESIAN_POINT('Ctrl Pts',(-9.31777466650694,1.40852059510137,-1.18061129751514));
#28417=CARTESIAN_POINT('Ctrl Pts',(-9.20675316942812,1.75636761288009,0.541244964014445));
#28418=CARTESIAN_POINT('Ctrl Pts',(-9.09573167234929,0.499673697483888,
1.76864340631115));
#28419=CARTESIAN_POINT('Ctrl Pts',(-8.99016602440781,-1.12931106646732,
1.3993710384868));
#28420=CARTESIAN_POINT('Ctrl Pts',(-8.92160754215929,-1.55311296873919,
0.438270790237053));
#28421=CARTESIAN_POINT('Ctrl Pts',(-8.8900562256037,-1.55680109303704,-0.00117256108905984));
#28422=CARTESIAN_POINT('Ctrl Pts',(-9.4519437743963,-1.55695751420806,-0.00111193227041606));
#28423=CARTESIAN_POINT('Ctrl Pts',(-9.44690493349759,-1.55752501833762,
-0.0712739806210275));
#28424=CARTESIAN_POINT('Ctrl Pts',(-9.40485892690594,-1.52136701702691,
-0.656144510346978));
#28425=CARTESIAN_POINT('Ctrl Pts',(-9.32580575462134,-0.780467016280449,
-1.66392437136285));
#28426=CARTESIAN_POINT('Ctrl Pts',(-9.21478425754254,0.973046316719188,
-1.5591516740318));
#28427=CARTESIAN_POINT('Ctrl Pts',(-9.10376276046368,1.83762692652266,-0.0300059333434424));
#28428=CARTESIAN_POINT('Ctrl Pts',(-8.99274126338489,1.02343163435251,1.5265519208083));
#28429=CARTESIAN_POINT('Ctrl Pts',(-8.88171976630603,-0.725726212115684,
1.68851844590611));
#28430=CARTESIAN_POINT('Ctrl Pts',(-8.80145393664319,-1.51099768765163,
0.690385345643029));
#28431=CARTESIAN_POINT('Ctrl Pts',(-8.75819527267327,-1.55725749910801,
0.088385929218701));
#28432=CARTESIAN_POINT('Ctrl Pts',(-8.7519437743963,-1.55648790187904,0.00127023405263929));
#28433=CARTESIAN_POINT('Origin',(-16.9400562256037,0.,0.));
#28434=CARTESIAN_POINT('',(-10.2900562256037,-1.55535099785736,0.00141466667608078));
#28435=CARTESIAN_POINT('',(-10.1519437743963,-1.55310404192406,-0.000488110324520369));
#28436=CARTESIAN_POINT('',(-16.9400562256037,-1.5555,-7.70311135908521E-14));
#28437=CARTESIAN_POINT('Ctrl Pts',(-10.2900562256037,-1.55535099785736,
0.00141466667608059));
#28438=CARTESIAN_POINT('Ctrl Pts',(-10.262019698115,-1.5517955612436,-0.390013984173206));
#28439=CARTESIAN_POINT('Ctrl Pts',(-10.1969760049333,-1.20367189210361,
-1.30374819544608));
#28440=CARTESIAN_POINT('Ctrl Pts',(-10.0949251460587,0.330292110303061,
-1.80794923173099));
#28441=CARTESIAN_POINT('Ctrl Pts',(-9.98390364897991,1.69735659323361,-0.704807702888898));
#28442=CARTESIAN_POINT('Ctrl Pts',(-9.87288215190106,1.51379003966279,1.04221543764369));
#28443=CARTESIAN_POINT('Ctrl Pts',(-9.76186065482225,-0.0527091443318308,
1.83711595952703));
#28444=CARTESIAN_POINT('Ctrl Pts',(-9.66758534605645,-1.34203220347939,
1.08695838544496));
#28445=CARTESIAN_POINT('Ctrl Pts',(-9.61031720298361,-1.55240389750898,
0.283530999109612));
#28446=CARTESIAN_POINT('Ctrl Pts',(-9.5900562256037,-1.55305431186606,-0.000397270594050692));
#28447=CARTESIAN_POINT('Ctrl Pts',(-10.1519437743963,-1.55310404192406,
-0.000488110324520508));
#28448=CARTESIAN_POINT('Ctrl Pts',(-10.1356145943219,-1.5537492772768,-0.22929960521096));
#28449=CARTESIAN_POINT('Ctrl Pts',(-10.0822782485546,-1.3992198808917,-0.975842246865478));
#28450=CARTESIAN_POINT('Ctrl Pts',(-9.99193473709432,-0.246555808489883,
-1.82125871594808));
#28451=CARTESIAN_POINT('Ctrl Pts',(-9.88091324001547,1.39517473801909,-1.19635301124305));
#28452=CARTESIAN_POINT('Ctrl Pts',(-9.76989174293666,1.76233442608894,0.521488684190485));
#28453=CARTESIAN_POINT('Ctrl Pts',(-9.65887024585783,0.519502160386579,
1.76292103693575));
#28454=CARTESIAN_POINT('Ctrl Pts',(-9.5528875896777,-1.1199772158385,1.41057736623951));
#28455=CARTESIAN_POINT('Ctrl Pts',(-9.48391209919053,-1.55335705197859,
0.444022811014936));
#28456=CARTESIAN_POINT('Ctrl Pts',(-9.4519437743963,-1.55695751420806,-0.00111193227041606));
#28457=CARTESIAN_POINT('Origin',(-16.9400562256037,0.,0.));
#28458=CARTESIAN_POINT('',(-10.9900562256037,-1.5577736303666,-0.000579010970803218));
#28459=CARTESIAN_POINT('',(-10.8519437743963,-1.55517737544971,0.00141046793165706));
#28460=CARTESIAN_POINT('',(-16.9400562256037,-1.5555,-7.70311135908521E-14));
#28461=CARTESIAN_POINT('Ctrl Pts',(-10.9900562256037,-1.5577736303666,-0.000579010970803324));
#28462=CARTESIAN_POINT('Ctrl Pts',(-10.9877365246322,-1.55792790669674,
-0.0328345769997972));
#28463=CARTESIAN_POINT('Ctrl Pts',(-10.9484096579678,-1.54241106195977,
-0.579525553204954));
#28464=CARTESIAN_POINT('Ctrl Pts',(-10.8720756256105,-0.900100912087758,
-1.60237063462356));
#28465=CARTESIAN_POINT('Ctrl Pts',(-10.7610541285317,0.85637872338898,-1.62615767524916));
#28466=CARTESIAN_POINT('Ctrl Pts',(-10.6500326314529,1.83050806619295,-0.164357908990289));
#28467=CARTESIAN_POINT('Ctrl Pts',(-10.539011134374,1.13236498768008,1.44759208250163));
#28468=CARTESIAN_POINT('Ctrl Pts',(-10.4279896372952,-0.600257410937894,
1.73708501325043));
#28469=CARTESIAN_POINT('Ctrl Pts',(-10.3450046677051,-1.48544841640631,
0.767296463912538));
#28470=CARTESIAN_POINT('Ctrl Pts',(-10.2990268638079,-1.5564886043435,0.126657167229999));
#28471=CARTESIAN_POINT('Ctrl Pts',(-10.2900562256037,-1.55535099785736,
0.00141466667608059));
#28472=CARTESIAN_POINT('Ctrl Pts',(-10.8519437743963,-1.55517737544971,
0.00141046793165704));
#28473=CARTESIAN_POINT('Ctrl Pts',(-10.8243242551462,-1.5517190272114,-0.384305966949585));
#28474=CARTESIAN_POINT('Ctrl Pts',(-10.7596975702032,-1.21199099487677,
-1.29228056265986));
#28475=CARTESIAN_POINT('Ctrl Pts',(-10.6580637195673,0.309969930699919,
-1.81154401524745));
#28476=CARTESIAN_POINT('Ctrl Pts',(-10.5470422224884,1.68933528416089,-0.723822750959111));
#28477=CARTESIAN_POINT('Ctrl Pts',(-10.4360207254096,1.52539751963279,1.02515144452665));
#28478=CARTESIAN_POINT('Ctrl Pts',(-10.3249992283308,-0.0320769633279623,
1.83759194206456));
#28479=CARTESIAN_POINT('Ctrl Pts',(-10.2303069113264,-1.33548212909013,
1.09870548750621));
#28480=CARTESIAN_POINT('Ctrl Pts',(-10.1726217600148,-1.55228696676881,
0.289260718402204));
#28481=CARTESIAN_POINT('Ctrl Pts',(-10.1519437743963,-1.55310404192406,
-0.000488110324520508));
#28482=CARTESIAN_POINT('Origin',(-16.9400562256037,0.,0.));
#28483=CARTESIAN_POINT('',(-11.6900562256037,-1.55366781884501,-0.00100983995776636));
#28484=CARTESIAN_POINT('',(-11.5519437743963,-1.55785653804749,-0.000480323856083265));
#28485=CARTESIAN_POINT('',(-16.9400562256037,-1.5555,-7.70311135908521E-14));
#28486=CARTESIAN_POINT('Ctrl Pts',(-11.6900562256037,-1.55366781884501,
-0.00100983995776658));
#28487=CARTESIAN_POINT('Ctrl Pts',(-11.6764461854566,-1.55480484065087,
-0.191546334115928));
#28488=CARTESIAN_POINT('Ctrl Pts',(-11.6258289796165,-1.43412071110437,
-0.898781982870385));
#28489=CARTESIAN_POINT('Ctrl Pts',(-11.5382046080835,-0.379130133977537,
-1.79834191525306));
#28490=CARTESIAN_POINT('Ctrl Pts',(-11.4271831110046,1.30391677723258,-1.2952120832884));
#28491=CARTESIAN_POINT('Ctrl Pts',(-11.3161616139258,1.79576212723163,0.391167080728389));
#28492=CARTESIAN_POINT('Ctrl Pts',(-11.205140116847,0.647077432006542,1.72019304138606));
#28493=CARTESIAN_POINT('Ctrl Pts',(-11.0964383207396,-1.05639680161046,
1.48279173541205));
#28494=CARTESIAN_POINT('Ctrl Pts',(-11.0247436903252,-1.55546667148486,
0.481752040517312));
#28495=CARTESIAN_POINT('Ctrl Pts',(-10.9900562256037,-1.5577736303666,-0.000579010970803324));
#28496=CARTESIAN_POINT('Ctrl Pts',(-11.5519437743963,-1.55785653804749,
-0.000480323856082957));
#28497=CARTESIAN_POINT('Ctrl Pts',(-11.5500410816635,-1.55796398188818,
-0.026933615327131));
#28498=CARTESIAN_POINT('Ctrl Pts',(-11.5111312232377,-1.54537528569271,
-0.567796152963855));
#28499=CARTESIAN_POINT('Ctrl Pts',(-11.435214199119,-0.918037049911427,
-1.59216238245569));
#28500=CARTESIAN_POINT('Ctrl Pts',(-11.3241927020402,0.838064683925275,
-1.63567131865609));
#28501=CARTESIAN_POINT('Ctrl Pts',(-11.2131712049614,1.82854703367336,-0.184902197827091));
#28502=CARTESIAN_POINT('Ctrl Pts',(-11.1021497078826,1.14854847598013,1.43478551548331));
#28503=CARTESIAN_POINT('Ctrl Pts',(-10.9911282108037,-0.580713931678918,
1.74371568974732));
#28504=CARTESIAN_POINT('Ctrl Pts',(-10.907726232975,-1.4812414118026,0.779105032812509));
#28505=CARTESIAN_POINT('Ctrl Pts',(-10.8613314208392,-1.55635283944833,
0.132512297948512));
#28506=CARTESIAN_POINT('Ctrl Pts',(-10.8519437743963,-1.55517737544971,
0.00141046793165704));
#28507=CARTESIAN_POINT('Origin',(-16.9400562256037,0.,0.));
#28508=CARTESIAN_POINT('',(-12.3900562256037,-1.55413552921628,0.00122121428746227));
#28509=CARTESIAN_POINT('',(-12.2519437743963,-1.55378767035869,-0.0010750654722666));
#28510=CARTESIAN_POINT('',(-16.9400562256037,-1.5555,-7.70311135908521E-14));
#28511=CARTESIAN_POINT('Ctrl Pts',(-12.3900562256037,-1.55413552921628,
0.0012212142874622));
#28512=CARTESIAN_POINT('Ctrl Pts',(-12.3651558462809,-1.55156996285741,
-0.347112742422888));
#28513=CARTESIAN_POINT('Ctrl Pts',(-12.3032483012651,-1.2636873551123,-1.21698840048794));
#28514=CARTESIAN_POINT('Ctrl Pts',(-12.2043335905564,0.176615125299183,
-1.82936611977922));
#28515=CARTESIAN_POINT('Ctrl Pts',(-12.0933120934776,1.63185729621746,-0.845467366266227));
#28516=CARTESIAN_POINT('Ctrl Pts',(-11.9822905963988,1.59630573484127,0.910813539398446));
#28517=CARTESIAN_POINT('Ctrl Pts',(-11.8712690993199,0.10243879880857,1.83501487600212));
#28518=CARTESIAN_POINT('Ctrl Pts',(-11.7738576423882,-1.29040741479283,
1.17503675398003));
#28519=CARTESIAN_POINT('Ctrl Pts',(-11.7134533511495,-1.55171315584237,
0.326542924521853));
#28520=CARTESIAN_POINT('Ctrl Pts',(-11.6900562256037,-1.55366781884501,
-0.00100983995776658));
#28521=CARTESIAN_POINT('Ctrl Pts',(-12.2519437743963,-1.55378767035869,
-0.00107506547226662));
#28522=CARTESIAN_POINT('Ctrl Pts',(-12.2387507424878,-1.55496678448482,
-0.185737759807948));
#28523=CARTESIAN_POINT('Ctrl Pts',(-12.1885505448864,-1.43915025335468,
-0.886958792124525));
#28524=CARTESIAN_POINT('Ctrl Pts',(-12.101343181592,-0.399299683385937,
-1.79397124836776));
#28525=CARTESIAN_POINT('Ctrl Pts',(-11.9903216845132,1.28929067374477,-1.30977197851782));
#28526=CARTESIAN_POINT('Ctrl Pts',(-11.8793001874343,1.80004124060888,0.370977909346943));
#28527=CARTESIAN_POINT('Ctrl Pts',(-11.7682786903555,0.666352550691795,
1.71281854126591));
#28528=CARTESIAN_POINT('Ctrl Pts',(-11.6591598860095,-1.04622477450308,
1.49372311766702));
#28529=CARTESIAN_POINT('Ctrl Pts',(-11.5870482473564,-1.55587421093005,
0.487580012496977));
#28530=CARTESIAN_POINT('Ctrl Pts',(-11.5519437743963,-1.55785653804749,
-0.000480323856082957));
#28531=CARTESIAN_POINT('Origin',(-16.9400562256037,0.,0.));
#28532=CARTESIAN_POINT('',(-13.0900562256037,-1.55800332081628,0.000210157868350831));
#28533=CARTESIAN_POINT('',(-12.9519437743963,-1.55399622131086,0.00116937500724938));
#28534=CARTESIAN_POINT('',(-16.9400562256037,-1.5555,-7.70311135908521E-14));
#28535=CARTESIAN_POINT('Ctrl Pts',(-13.0900562256037,-1.55800332081628,
0.00021015786835074));
#28536=CARTESIAN_POINT('Ctrl Pts',(-13.0538655071052,-1.55704751416205,
-0.502825518255894));
#28537=CARTESIAN_POINT('Ctrl Pts',(-12.9806676229138,-1.0191962748975,-1.52200078717984));
#28538=CARTESIAN_POINT('Ctrl Pts',(-12.8704625730293,0.716160935289581,
-1.69259765416285));
#28539=CARTESIAN_POINT('Ctrl Pts',(-12.7594410759505,1.81012100052783,-0.318174898587703));
#28540=CARTESIAN_POINT('Ctrl Pts',(-12.6484195788717,1.25043337930754,1.3469185818581));
#28541=CARTESIAN_POINT('Ctrl Pts',(-12.5373980817929,-0.451595700759593,
1.78152592625865));
#28542=CARTESIAN_POINT('Ctrl Pts',(-12.4512769640369,-1.45185853317557,
0.856161387294219));
#28543=CARTESIAN_POINT('Ctrl Pts',(-12.4021630119738,-1.55538293044751,
0.170584288828434));
#28544=CARTESIAN_POINT('Ctrl Pts',(-12.3900562256037,-1.55413552921628,
0.0012212142874622));
#28545=CARTESIAN_POINT('Ctrl Pts',(-12.9519437743963,-1.55399622131086,
0.00116937500724928));
#28546=CARTESIAN_POINT('Ctrl Pts',(-12.9274604033121,-1.55159520168044,
-0.341408350569593));
#28547=CARTESIAN_POINT('Ctrl Pts',(-12.865969866535,-1.2712304187298,-1.20537147389457));
#28548=CARTESIAN_POINT('Ctrl Pts',(-12.767472164065,0.156062150750201,-1.83123392346586));
#28549=CARTESIAN_POINT('Ctrl Pts',(-12.6564506669861,1.62226066059323,-0.863738054150705));
#28550=CARTESIAN_POINT('Ctrl Pts',(-12.5454291699073,1.60643250632205,0.892831271683784));
#28551=CARTESIAN_POINT('Ctrl Pts',(-12.4344076728285,0.123037600173064,
1.8337488448793));
#28552=CARTESIAN_POINT('Ctrl Pts',(-12.3365792076581,-1.28312558209438,
1.18669436910945));
#28553=CARTESIAN_POINT('Ctrl Pts',(-12.2757579081807,-1.55165930579917,
0.332251052315397));
#28554=CARTESIAN_POINT('Ctrl Pts',(-12.2519437743963,-1.55378767035869,
-0.00107506547226662));
#28555=CARTESIAN_POINT('Origin',(-16.9400562256037,0.,0.));
#28556=CARTESIAN_POINT('',(-13.7900562256037,-1.55473841727083,-0.00136756133992672));
#28557=CARTESIAN_POINT('',(-13.6519437743963,-1.55795954537968,0.000315683116621389));
#28558=CARTESIAN_POINT('',(-16.9400562256037,-1.5555,-7.70311135908521E-14));
#28559=CARTESIAN_POINT('Ctrl Pts',(-13.7900562256037,-1.55473841727083,
-0.00136756133992656));
#28560=CARTESIAN_POINT('Ctrl Pts',(-13.7795823336225,-1.55598127536203,
-0.147744259734356));
#28561=CARTESIAN_POINT('Ctrl Pts',(-13.7321012759483,-1.46991308354017,
-0.809877587435659));
#28562=CARTESIAN_POINT('Ctrl Pts',(-13.6476130525811,-0.529468511212632,
-1.75995347711011));
#28563=CARTESIAN_POINT('Ctrl Pts',(-13.5365915555023,1.19001920390447,-1.40058118296215));
#28564=CARTESIAN_POINT('Ctrl Pts',(-13.4255700584235,1.82235723230149,0.238301140323824));
#28565=CARTESIAN_POINT('Ctrl Pts',(-13.3145485613446,0.789869078999073,
1.65948188258691));
#28566=CARTESIAN_POINT('Ctrl Pts',(-13.2035270642659,-0.964209049677692,
1.56463229551752));
#28567=CARTESIAN_POINT('Ctrl Pts',(-13.1286962856855,-1.5527764949361,0.537270179800524));
#28568=CARTESIAN_POINT('Ctrl Pts',(-13.0908726727981,-1.55802488340729,
0.0115584284612541));
#28569=CARTESIAN_POINT('Ctrl Pts',(-13.0900562256037,-1.55800332081628,
0.00021015786835074));
#28570=CARTESIAN_POINT('Ctrl Pts',(-13.6519437743963,-1.55795954537968,
0.000315683116621417));
#28571=CARTESIAN_POINT('Ctrl Pts',(-13.6161700641364,-1.55657771788537,
-0.496961205609469));
#28572=CARTESIAN_POINT('Ctrl Pts',(-13.5433891881836,-1.02966362241915,
-1.51117950611935));
#28573=CARTESIAN_POINT('Ctrl Pts',(-13.4336011465379,0.697109689533605,
-1.70053261271694));
#28574=CARTESIAN_POINT('Ctrl Pts',(-13.3225796494591,1.8064340535295,-0.338480558245879));
#28575=CARTESIAN_POINT('Ctrl Pts',(-13.2115581523802,1.26547896337724,1.33279258226153));
#28576=CARTESIAN_POINT('Ctrl Pts',(-13.1005366553014,-0.431562574783867,
1.78648448709609));
#28577=CARTESIAN_POINT('Ctrl Pts',(-13.0139985293068,-1.44704656389406,
0.867984154568371));
#28578=CARTESIAN_POINT('Ctrl Pts',(-12.9644675690051,-1.55522439681821,
0.176405581570162));
#28579=CARTESIAN_POINT('Ctrl Pts',(-12.9519437743963,-1.55399622131086,
0.00116937500724928));
#28580=CARTESIAN_POINT('Origin',(-16.9400562256037,0.,0.));
#28581=CARTESIAN_POINT('',(-14.4900562256037,-1.55328082746597,0.000715383538183075));
#28582=CARTESIAN_POINT('',(-14.3519437743963,-1.55490416069612,-0.00138938706337133));
#28583=CARTESIAN_POINT('',(-16.9400562256037,-1.5555,-7.70311135908521E-14));
#28584=CARTESIAN_POINT('Ctrl Pts',(-14.4900562256037,-1.55328082746597,
0.000715383538183074));
#28585=CARTESIAN_POINT('Ctrl Pts',(-14.4682919944468,-1.55201539840468,
-0.304168296634556));
#28586=CARTESIAN_POINT('Ctrl Pts',(-14.4095205975969,-1.31797175976879,
-1.129261225486));
#28587=CARTESIAN_POINT('Ctrl Pts',(-14.3137420350541,0.0216796534424384,
-1.83774207162163));
#28588=CARTESIAN_POINT('Ctrl Pts',(-14.2027205379753,1.55472664688603,-0.980101962297276));
#28589=CARTESIAN_POINT('Ctrl Pts',(-14.0916990408964,1.66744375345186,0.772920313447068));
#28590=CARTESIAN_POINT('Ctrl Pts',(-13.9806775438176,0.256856552130983,
1.81983431302347));
#28591=CARTESIAN_POINT('Ctrl Pts',(-13.88012993872,-1.23316965064986,1.26230497981326));
#28592=CARTESIAN_POINT('Ctrl Pts',(-13.8165894993154,-1.55158991297295,
0.369445218710443));
#28593=CARTESIAN_POINT('Ctrl Pts',(-13.7900562256037,-1.55473841727083,
-0.00136756133992656));
#28594=CARTESIAN_POINT('Ctrl Pts',(-14.3519437743963,-1.55490416069612,
-0.00138938706337152));
#28595=CARTESIAN_POINT('Ctrl Pts',(-14.3418868906537,-1.55612679718045,
-0.141900236675545));
#28596=CARTESIAN_POINT('Ctrl Pts',(-14.2948228412182,-1.47432573136466,
-0.798062339120933));
#28597=CARTESIAN_POINT('Ctrl Pts',(-14.2107516260897,-0.549197426397097,
-1.75389685400554));
#28598=CARTESIAN_POINT('Ctrl Pts',(-14.0997301290109,1.17421705517224,-1.41385560804608));
#28599=CARTESIAN_POINT('Ctrl Pts',(-13.988708631932,1.82491817106717,0.217823042681003));
#28600=CARTESIAN_POINT('Ctrl Pts',(-13.8776871348532,0.808453455731279,
1.65050777944339));
#28601=CARTESIAN_POINT('Ctrl Pts',(-13.7666656377744,-0.946579065961039,
1.57536065782744));
#28602=CARTESIAN_POINT('Ctrl Pts',(-13.6914178509554,-1.54998955482229,
0.54898434204543));
#28603=CARTESIAN_POINT('Ctrl Pts',(-13.6531772298294,-1.55800718993816,
0.0174614830823369));
#28604=CARTESIAN_POINT('Ctrl Pts',(-13.6519437743963,-1.55795954537968,
0.000315683116621417));
#28605=CARTESIAN_POINT('Origin',(-16.9400562256037,0.,0.));
#28606=CARTESIAN_POINT('',(-15.1900562256037,-1.55731346481242,0.00103325697183645));
#28607=CARTESIAN_POINT('',(-15.0519437743963,-1.55320111767851,0.000640865722738582));
#28608=CARTESIAN_POINT('',(-16.9400562256037,-1.5555,-7.70311135908521E-14));
#28609=CARTESIAN_POINT('Ctrl Pts',(-15.1900562256037,-1.55731346481242,
0.00103325697183652));
#28610=CARTESIAN_POINT('Ctrl Pts',(-15.1570016552711,-1.55406616181334,
-0.458910165558249));
#28611=CARTESIAN_POINT('Ctrl Pts',(-15.0869399192455,-1.09517591543371,
-1.43978275398639));
#28612=CARTESIAN_POINT('Ctrl Pts',(-14.979871017527,0.570855243925188,-1.74687800671557));
#28613=CARTESIAN_POINT('Ctrl Pts',(-14.8688495204482,1.77682346771718,-0.469774267555894));
#28614=CARTESIAN_POINT('Ctrl Pts',(-14.7578280233694,1.3595938034014,1.2366712040288));
#28615=CARTESIAN_POINT('Ctrl Pts',(-14.6468065262906,-0.299717618166574,
1.81325504017035));
#28616=CARTESIAN_POINT('Ctrl Pts',(-14.5575492603687,-1.41360466166464,
0.94507199546461));
#28617=CARTESIAN_POINT('Ctrl Pts',(-14.5052991601397,-1.55416709136393,
0.214245645391361));
#28618=CARTESIAN_POINT('Ctrl Pts',(-14.4900562256037,-1.55328082746597,
0.000715383538183074));
#28619=CARTESIAN_POINT('Ctrl Pts',(-15.0519437743963,-1.55320111767851,
0.000640865722738825));
#28620=CARTESIAN_POINT('Ctrl Pts',(-15.030596551478,-1.55211155703931,-0.298442301630793));
#28621=CARTESIAN_POINT('Ctrl Pts',(-14.9722421628668,-1.32477770343153,
-1.11755737738762));
#28622=CARTESIAN_POINT('Ctrl Pts',(-14.8768806085626,0.00104665412810624,
-1.83785829362665));
#28623=CARTESIAN_POINT('Ctrl Pts',(-14.7658591114838,1.54362083748287,-0.99750399698833));
#28624=CARTESIAN_POINT('Ctrl Pts',(-14.654837614405,1.67601881849698,0.754151058535186));
#28625=CARTESIAN_POINT('Ctrl Pts',(-14.5438161173262,0.277274533789786,
1.81683365360614));
#28626=CARTESIAN_POINT('Ctrl Pts',(-14.4428515039899,-1.22512254880408,
1.2738304268474));
#28627=CARTESIAN_POINT('Ctrl Pts',(-14.3788940563466,-1.55162775830162,
0.375149420687903));
#28628=CARTESIAN_POINT('Ctrl Pts',(-14.3519437743963,-1.55490416069612,
-0.00138938706337152));
#28629=CARTESIAN_POINT('Ctrl Pts',(-15.8760740822721,-0.685825729128752,
1.39614588036674));
#28630=CARTESIAN_POINT('Ctrl Pts',(-15.8390669165791,-1.14959124433326,
1.16833134674053));
#28631=CARTESIAN_POINT('Ctrl Pts',(-15.7650525851932,-1.82433082916238,
0.2182728247837));
#28632=CARTESIAN_POINT('Ctrl Pts',(-15.6540310881144,-1.17303546001366,
-1.41641485775535));
#28633=CARTESIAN_POINT('Ctrl Pts',(-15.5430095910356,0.551406182529313,
-1.75263860476265));
#28634=CARTESIAN_POINT('Ctrl Pts',(-15.4319880939568,1.77133009557791,-0.489978596140976));
#28635=CARTESIAN_POINT('Ctrl Pts',(-15.3209665968779,1.37345033995276,1.2214745163176));
#28636=CARTESIAN_POINT('Ctrl Pts',(-15.2099450997991,-0.279367108572254,
1.81642835228867));
#28637=CARTESIAN_POINT('Ctrl Pts',(-15.0989236027203,-1.67685487580139,
0.752294539512666));
#28638=CARTESIAN_POINT('Ctrl Pts',(-14.9879021056415,-1.54249996813387,
-0.999272066172348));
#28639=CARTESIAN_POINT('Ctrl Pts',(-14.8768806085626,0.00104665412810624,
-1.83785829362665));
#28640=CARTESIAN_POINT('Ctrl Pts',(-14.7658591114838,1.54362083748287,-0.99750399698833));
#28641=CARTESIAN_POINT('Ctrl Pts',(-14.654837614405,1.67601881849698,0.754151058535186));
#28642=CARTESIAN_POINT('Ctrl Pts',(-14.5438161173262,0.277274533789786,
1.81683365360614));
#28643=CARTESIAN_POINT('Ctrl Pts',(-14.4327946202473,-1.37477332540386,
1.21974295854618));
#28644=CARTESIAN_POINT('Ctrl Pts',(-14.3217731231685,-1.77088940801687,
-0.491655328889854));
#28645=CARTESIAN_POINT('Ctrl Pts',(-14.2107516260897,-0.549197426397097,
-1.75389685400554));
#28646=CARTESIAN_POINT('Ctrl Pts',(-14.0997301290109,1.17421705517224,-1.41385560804608));
#28647=CARTESIAN_POINT('Ctrl Pts',(-13.988708631932,1.82491817106717,0.217823042681003));
#28648=CARTESIAN_POINT('Ctrl Pts',(-13.8776871348532,0.808453455731279,
1.65050777944339));
#28649=CARTESIAN_POINT('Ctrl Pts',(-13.7666656377744,-0.946579065961039,
1.57536065782744));
#28650=CARTESIAN_POINT('Ctrl Pts',(-13.6556441406956,-1.83685821779324,
0.0610325963455999));
#28651=CARTESIAN_POINT('Ctrl Pts',(-13.5446226436167,-1.04906371273324,
-1.5090521467585));
#28652=CARTESIAN_POINT('Ctrl Pts',(-13.4336011465379,0.697109689533605,
-1.70053261271694));
#28653=CARTESIAN_POINT('Ctrl Pts',(-13.3225796494591,1.8064340535295,-0.338480558245879));
#28654=CARTESIAN_POINT('Ctrl Pts',(-13.2115581523802,1.26547896337724,1.33279258226153));
#28655=CARTESIAN_POINT('Ctrl Pts',(-13.1005366553014,-0.431562574783867,
1.78648448709609));
#28656=CARTESIAN_POINT('Ctrl Pts',(-12.9895151582226,-1.73434734663761,
0.60812199296339));
#28657=CARTESIAN_POINT('Ctrl Pts',(-12.8784936611437,-1.45270794093109,
-1.12579425965292));
#28658=CARTESIAN_POINT('Ctrl Pts',(-12.767472164065,0.156062150750201,-1.83123392346586));
#28659=CARTESIAN_POINT('Ctrl Pts',(-12.6564506669861,1.62226066059323,-0.863738054150705));
#28660=CARTESIAN_POINT('Ctrl Pts',(-12.5454291699073,1.60643250632205,0.892831271683784));
#28661=CARTESIAN_POINT('Ctrl Pts',(-12.4344076728285,0.123037600173064,
1.8337488448793));
#28662=CARTESIAN_POINT('Ctrl Pts',(-12.3233861757497,-1.47275909724666,
1.09943336250467));
#28663=CARTESIAN_POINT('Ctrl Pts',(-12.2123646786708,-1.72310724567287,
-0.639276541897258));
#28664=CARTESIAN_POINT('Ctrl Pts',(-12.101343181592,-0.399299683385937,
-1.79397124836776));
#28665=CARTESIAN_POINT('Ctrl Pts',(-11.9903216845132,1.28929067374477,-1.30977197851782));
#28666=CARTESIAN_POINT('Ctrl Pts',(-11.8793001874343,1.80004124060888,0.370977909346943));
#28667=CARTESIAN_POINT('Ctrl Pts',(-11.7682786903555,0.666352550691795,
1.71281854126591));
#28668=CARTESIAN_POINT('Ctrl Pts',(-11.6572571932767,-1.07608679920682,
1.4899027745761));
#28669=CARTESIAN_POINT('Ctrl Pts',(-11.5462356961979,-1.83546013017251,
-0.0941232578271086));
#28670=CARTESIAN_POINT('Ctrl Pts',(-11.435214199119,-0.918037049911427,
-1.59216238245569));
#28671=CARTESIAN_POINT('Ctrl Pts',(-11.3241927020402,0.838064683925275,
-1.63567131865609));
#28672=CARTESIAN_POINT('Ctrl Pts',(-11.2131712049614,1.82854703367336,-0.184902197827091));
#28673=CARTESIAN_POINT('Ctrl Pts',(-11.1021497078826,1.14854847598013,1.43478551548331));
#28674=CARTESIAN_POINT('Ctrl Pts',(-10.9911282108037,-0.580713931678918,
1.74371568974732));
#28675=CARTESIAN_POINT('Ctrl Pts',(-10.8801067137249,-1.77946139075276,
0.459663176616526));
#28676=CARTESIAN_POINT('Ctrl Pts',(-10.7690852166461,-1.35257044729127,
-1.24431758897447));
#28677=CARTESIAN_POINT('Ctrl Pts',(-10.6580637195673,0.309969930699919,
-1.81154401524745));
#28678=CARTESIAN_POINT('Ctrl Pts',(-10.5470422224884,1.68933528416089,-0.723822750959111));
#28679=CARTESIAN_POINT('Ctrl Pts',(-10.4360207254096,1.52539751963279,1.02515144452665));
#28680=CARTESIAN_POINT('Ctrl Pts',(-10.3249992283308,-0.0320769633279623,
1.83759194206456));
#28681=CARTESIAN_POINT('Ctrl Pts',(-10.213977731252,-1.56024733005802,0.971288497905627));
#28682=CARTESIAN_POINT('Ctrl Pts',(-10.1029562341731,-1.66304370981859,
-0.782341802762569));
#28683=CARTESIAN_POINT('Ctrl Pts',(-9.99193473709432,-0.246555808489883,
-1.82125871594808));
#28684=CARTESIAN_POINT('Ctrl Pts',(-9.88091324001547,1.39517473801909,-1.19635301124305));
#28685=CARTESIAN_POINT('Ctrl Pts',(-9.76989174293666,1.76233442608894,0.521488684190485));
#28686=CARTESIAN_POINT('Ctrl Pts',(-9.65887024585783,0.519502160386579,
1.76292103693575));
#28687=CARTESIAN_POINT('Ctrl Pts',(-9.547848748779,-1.19792464640174,1.39382553379547));
#28688=CARTESIAN_POINT('Ctrl Pts',(-9.43682725170018,-1.82097968505047,
-0.248608253584697));
#28689=CARTESIAN_POINT('Ctrl Pts',(-9.32580575462134,-0.780467016280449,
-1.66392437136285));
#28690=CARTESIAN_POINT('Ctrl Pts',(-9.21478425754254,0.973046316719188,
-1.5591516740318));
#28691=CARTESIAN_POINT('Ctrl Pts',(-9.10376276046368,1.83762692652266,-0.0300059333434424));
#28692=CARTESIAN_POINT('Ctrl Pts',(-8.99274126338489,1.02343163435251,1.5265519208083));
#28693=CARTESIAN_POINT('Ctrl Pts',(-8.88171976630603,-0.725726212115684,
1.68851844590611));
#28694=CARTESIAN_POINT('Ctrl Pts',(-8.77069826922724,-1.81189220820005,
0.307928080858025));
#28695=CARTESIAN_POINT('Ctrl Pts',(-8.65967677214839,-1.24279241981098,
-1.35397196366001));
#28696=CARTESIAN_POINT('Ctrl Pts',(-8.54865527506958,0.461668379793908,
-1.77894220935235));
#28697=CARTESIAN_POINT('Ctrl Pts',(-8.43763377799074,1.74436906067446,-0.578748354018101));
#28698=CARTESIAN_POINT('Ctrl Pts',(-8.32661228091193,1.43349016294594,1.15016478378281));
#28699=CARTESIAN_POINT('Ctrl Pts',(-8.21559078383309,-0.186962896184165,
1.82833748322551));
#28700=CARTESIAN_POINT('Ctrl Pts',(-8.10456928675427,-1.63661479859031,
0.836220711386745));
#28701=CARTESIAN_POINT('Ctrl Pts',(-7.99354778967544,-1.59112672180277,
-0.919830871563968));
#28702=CARTESIAN_POINT('Ctrl Pts',(-7.88252629259662,-0.0920545910400277,
-1.83556504362701));
#28703=CARTESIAN_POINT('Ctrl Pts',(-7.77150479551779,1.49111460364442,-1.07440696010184));
#28704=CARTESIAN_POINT('Ctrl Pts',(-7.66048329843897,1.71206645837288,0.668282514533717));
#28705=CARTESIAN_POINT('Ctrl Pts',(-7.54946180136013,0.368948984659062,
1.80045819830287));
#28706=CARTESIAN_POINT('Ctrl Pts',(-7.43844030428131,-1.31122420779922,
1.28781371090631));
#28707=CARTESIAN_POINT('Ctrl Pts',(-7.3274188072025,-1.7935200888365,-0.401321277852141));
#28708=CARTESIAN_POINT('Ctrl Pts',(-7.21639731012365,-0.637334153250706,
-1.723826631137));
#28709=CARTESIAN_POINT('Ctrl Pts',(-7.10537581304485,1.10109249863036,-1.47151907448626));
#28710=CARTESIAN_POINT('Ctrl Pts',(-6.994354315966,1.83360901398418,0.125104200380868));
#28711=CARTESIAN_POINT('Ctrl Pts',(-6.8833328188872,0.891020217215038,1.60743772807255));
#28712=CARTESIAN_POINT('Ctrl Pts',(-6.77231132180836,-0.865565831794229,
1.62128617706663));
#28713=CARTESIAN_POINT('Ctrl Pts',(-6.66128982472953,-1.83140864613746,
0.153998207683987));
#28714=CARTESIAN_POINT('Ctrl Pts',(-6.55026832765071,-1.12415630856125,
-1.45397581514925));
#28715=CARTESIAN_POINT('Ctrl Pts',(-6.43924683057189,0.610076257496618,
-1.73366087720635));
#28716=CARTESIAN_POINT('Ctrl Pts',(-6.32822533349305,1.78696973330201,-0.429548890557871));
#28717=CARTESIAN_POINT('Ctrl Pts',(-6.21720383641424,1.3313655119277,1.26698024876731));
#28718=CARTESIAN_POINT('Ctrl Pts',(-6.10618233933541,-0.340516238842866,
1.80605143010969));
#28719=CARTESIAN_POINT('Ctrl Pts',(-5.99516084225658,-1.70131718874498,
0.695192707382526));
#28720=CARTESIAN_POINT('Ctrl Pts',(-5.88413934517776,-1.50786887463394,
-1.05076378602764));
#28721=CARTESIAN_POINT('Ctrl Pts',(-5.77311784809893,0.0631027514921653,
-1.83678826212252));
#28722=CARTESIAN_POINT('Ctrl Pts',(-5.6620963510201,1.57642645299097,-0.944803003502463));
#28723=CARTESIAN_POINT('Ctrl Pts',(-5.55107485394128,1.64959562566877,0.810313117807789));
#28724=CARTESIAN_POINT('Ctrl Pts',(-5.44005335686245,0.215766101057041,
1.82516247680901));
#28725=CARTESIAN_POINT('Ctrl Pts',(-5.32903185978363,-1.41517793340943,
1.17262291206848));
#28726=CARTESIAN_POINT('Ctrl Pts',(-5.2180103627048,-1.75327706158784,-0.551173858620724));
#28727=CARTESIAN_POINT('Ctrl Pts',(-5.10698886562598,-0.489658649608892,
-1.77144220452719));
#28728=CARTESIAN_POINT('Ctrl Pts',(-4.99596736854715,1.22129057217261,-1.37339812706995));
#28729=CARTESIAN_POINT('Ctrl Pts',(-4.88494587146833,1.81652193399072,0.279322645783608));
#28730=CARTESIAN_POINT('Ctrl Pts',(-4.77392437438949,0.752257995551791,
1.67686641842616));
#28731=CARTESIAN_POINT('Ctrl Pts',(-4.66290287731068,-0.999236074733923,
1.54249808559599));
#28732=CARTESIAN_POINT('Ctrl Pts',(-4.55188138023185,-1.8378715998848,-0.00102929772714257));
#28733=CARTESIAN_POINT('Ctrl Pts',(-4.44085988315302,-0.997507700137877,
-1.5436163594892));
#28734=CARTESIAN_POINT('Ctrl Pts',(-4.3298383860742,0.754135777011385,-1.67602276444812));
#28735=CARTESIAN_POINT('Ctrl Pts',(-4.21881688899538,1.81683366297973,-0.277287789454163));
#28736=CARTESIAN_POINT('Ctrl Pts',(-4.10779539191654,1.21975146666773,1.37476522965911));
#28737=CARTESIAN_POINT('Ctrl Pts',(-3.99677389483772,-0.491642529871626,
1.77089262800929));
#28738=CARTESIAN_POINT('Ctrl Pts',(-3.88575239775889,-1.75389333002919,
0.549209672160667));
#28739=CARTESIAN_POINT('Ctrl Pts',(-3.77473090068007,-1.4138635940316,-1.17420731329451));
#28740=CARTESIAN_POINT('Ctrl Pts',(-3.66370940360124,0.217810325062528,
-1.82491965286328));
#28741=CARTESIAN_POINT('Ctrl Pts',(-3.55268790652242,1.65050222030251,-0.808464902075287));
#28742=CARTESIAN_POINT('Ctrl Pts',(-3.4416664094436,1.57536719290506,0.946568161661344));
#28743=CARTESIAN_POINT('Ctrl Pts',(-3.33064491236476,0.0610453305290268,
1.83685779108923));
#28744=CARTESIAN_POINT('Ctrl Pts',(-3.21962341528594,-1.50904488626973,
1.04907416721584));
#28745=CARTESIAN_POINT('Ctrl Pts',(-3.10860191820711,-1.70053743814524,
-0.697097911928709));
#28746=CARTESIAN_POINT('Ctrl Pts',(-2.99758042112829,-0.338493072017185,
-1.8064317083433));
#28747=CARTESIAN_POINT('Ctrl Pts',(-2.88655892404946,1.33278381758959,-1.26548819539577));
#28748=CARTESIAN_POINT('Ctrl Pts',(-2.77553742697064,1.78648747614462,0.431550201213581));
#28749=CARTESIAN_POINT('Ctrl Pts',(-2.66451592989181,0.608134005493306,
1.73434313370923));
#28750=CARTESIAN_POINT('Ctrl Pts',(-2.55349443281299,-1.12578419639739,
1.4527157399861));
#28751=CARTESIAN_POINT('Ctrl Pts',(-2.44247293573416,-1.83123500658462,
-0.156049469126138));
#28752=CARTESIAN_POINT('Ctrl Pts',(-2.33145143865534,-0.863749286419899,
-1.62225467335409));
#28753=CARTESIAN_POINT('Ctrl Pts',(-2.22042994157651,0.892820136543068,
-1.60643869907147));
#28754=CARTESIAN_POINT('Ctrl Pts',(-2.10940844449769,1.8337480082192,-0.123050285242695));
#28755=CARTESIAN_POINT('Ctrl Pts',(-1.99838694741886,1.09944353382152,1.47275145086502));
#28756=CARTESIAN_POINT('Ctrl Pts',(-1.88736545034003,-0.639264550272716,
1.72311173281902));
#28757=CARTESIAN_POINT('Ctrl Pts',(-1.77634395326121,-1.7939685901571,0.399311996552182));
#28758=CARTESIAN_POINT('Ctrl Pts',(-1.66532245618238,-1.30978070402824,
-1.28928138705521));
#28759=CARTESIAN_POINT('Ctrl Pts',(-1.55430095910356,0.370965051819814,
-1.80004421839588));
#28760=CARTESIAN_POINT('Ctrl Pts',(-1.44327946202473,1.71281466704483,-0.6663636376042));
#28761=CARTESIAN_POINT('Ctrl Pts',(-1.33225796494591,1.48990881738992,1.0760750010236));
#28762=CARTESIAN_POINT('Ctrl Pts',(-1.22123646786708,-0.0941078601541336,
1.83546359530854));
#28763=CARTESIAN_POINT('Ctrl Pts',(-1.11021497078826,-1.59216113185349,
0.918042724568974));
#28764=CARTESIAN_POINT('Ctrl Pts',(-0.999193473709428,-1.63566740285966,
-0.83804316724106));
#28765=CARTESIAN_POINT('Ctrl Pts',(-0.888171976630605,-0.184933360961542,
-1.82856513855231));
#28766=CARTESIAN_POINT('Ctrl Pts',(-0.777150479551777,1.43481276042301,
-1.14852152405029));
#28767=CARTESIAN_POINT('Ctrl Pts',(-0.666128982472953,1.74365272478113,
0.580631652352415));
#28768=CARTESIAN_POINT('Ctrl Pts',(-0.555107485394127,0.459803001478689,
1.7795918156029));
#28769=CARTESIAN_POINT('Ctrl Pts',(-0.444085988315302,-1.24455107634816,
1.35232464687182));
#28770=CARTESIAN_POINT('Ctrl Pts',(-0.333064491236475,-1.81108201871734,
-0.309471773373046));
#28771=CARTESIAN_POINT('Ctrl Pts',(-0.222042994157651,-0.72473494787801,
-1.69026698927826));
#28772=CARTESIAN_POINT('Ctrl Pts',(-0.111021497078823,1.0270020972766,-1.52351327282068));
#28773=CARTESIAN_POINT('Ctrl Pts',(-0.03700716569294,1.56427778786756,-0.489482550463674));
#28774=CARTESIAN_POINT('Ctrl Pts',(2.22044604925031E-15,1.55526325306019,
0.0271378643346999));
#28775=CARTESIAN_POINT('Ctrl Pts',(-15.7993827215147,-0.744392439309354,
1.51537102412034));
#28776=CARTESIAN_POINT('Ctrl Pts',(-15.7623755558218,-1.24776163131854,
1.26810206176809));
#28777=CARTESIAN_POINT('Ctrl Pts',(-15.6883612244359,-1.9801212149807,0.236912430628839));
#28778=CARTESIAN_POINT('Ctrl Pts',(-15.577339727357,-1.2732078870608,-1.53737088921693));
#28779=CARTESIAN_POINT('Ctrl Pts',(-15.4663182302782,0.598494013609971,
-1.90230676805375));
#28780=CARTESIAN_POINT('Ctrl Pts',(-15.3552967331994,1.92259443568029,-0.531820762767402));
#28781=CARTESIAN_POINT('Ctrl Pts',(-15.2442752361206,1.49073737744792,1.32578344051186));
#28782=CARTESIAN_POINT('Ctrl Pts',(-15.1332537390418,-0.303223916193815,
1.97154389892684));
#28783=CARTESIAN_POINT('Ctrl Pts',(-15.0222322419629,-1.82005141882225,
0.816537414043005));
#28784=CARTESIAN_POINT('Ctrl Pts',(-14.9112107448841,-1.67422315195502,
-1.08460581059957));
#28785=CARTESIAN_POINT('Ctrl Pts',(-14.8001892478053,0.00113603410668217,
-1.99480386954226));
#28786=CARTESIAN_POINT('Ctrl Pts',(-14.6891677507265,1.67543973895868,-1.08268675554397));
#28787=CARTESIAN_POINT('Ctrl Pts',(-14.5781462536476,1.81914396564604,0.818552472191297));
#28788=CARTESIAN_POINT('Ctrl Pts',(-14.4671247565688,0.300952644089851,
1.97198381131792));
#28789=CARTESIAN_POINT('Ctrl Pts',(-14.35610325949,-1.49217334044155,1.32390401479405));
#28790=CARTESIAN_POINT('Ctrl Pts',(-14.2450817624111,-1.92211611520528,
-0.533640681630147));
#28791=CARTESIAN_POINT('Ctrl Pts',(-14.1340602653324,-0.596096638744525,
-1.90367246663196));
#28792=CARTESIAN_POINT('Ctrl Pts',(-14.0230387682535,1.27449038560964,-1.53459309005752));
#28793=CARTESIAN_POINT('Ctrl Pts',(-13.9120172711747,1.98075871348017,0.236424238975518));
#28794=CARTESIAN_POINT('Ctrl Pts',(-13.8009957740958,0.877492071848058,
1.79145438827402));
#28795=CARTESIAN_POINT('Ctrl Pts',(-13.689974277017,-1.02741304384284,1.70989001004951));
#28796=CARTESIAN_POINT('Ctrl Pts',(-13.5789527799382,-1.99371839132599,
0.0662445302669022));
#28797=CARTESIAN_POINT('Ctrl Pts',(-13.4679312828594,-1.13864945997941,
-1.63791902353622));
#28798=CARTESIAN_POINT('Ctrl Pts',(-13.3569097857806,0.756640003747492,
-1.84575113755733));
#28799=CARTESIAN_POINT('Ctrl Pts',(-13.2458882887017,1.96069612796034,-0.367385412518035));
#28800=CARTESIAN_POINT('Ctrl Pts',(-13.1348667916229,1.37354568724006,1.44660761366219));
#28801=CARTESIAN_POINT('Ctrl Pts',(-13.023845294544,-0.468416252283351,
1.93904295020716));
#28802=CARTESIAN_POINT('Ctrl Pts',(-12.9128237974653,-1.88245351135101,
0.660053122117134));
#28803=CARTESIAN_POINT('Ctrl Pts',(-12.8018023003864,-1.57676325314819,
-1.22193248154763));
#28804=CARTESIAN_POINT('Ctrl Pts',(-12.6907808033076,0.16938921966136,-1.98761380528331));
#28805=CARTESIAN_POINT('Ctrl Pts',(-12.5797593062288,1.76079508108961,-0.937497748692457));
#28806=CARTESIAN_POINT('Ctrl Pts',(-12.4687378091499,1.74361526722837,0.969075407924211));
#28807=CARTESIAN_POINT('Ctrl Pts',(-12.3577163120711,0.133544507634545,
1.99034349069188));
#28808=CARTESIAN_POINT('Ctrl Pts',(-12.2466948149923,-1.59852669614364,
1.19332047167817));
#28809=CARTESIAN_POINT('Ctrl Pts',(-12.1356733179135,-1.87025355176966,
-0.693868142014267));
#28810=CARTESIAN_POINT('Ctrl Pts',(-12.0246518208346,-0.433398242012175,
-1.94716905024808));
#28811=CARTESIAN_POINT('Ctrl Pts',(-11.9136303237558,1.39939082021156,-1.42162114458219));
#28812=CARTESIAN_POINT('Ctrl Pts',(-11.802608826677,1.9537573949821,0.402657904391348));
#28813=CARTESIAN_POINT('Ctrl Pts',(-11.6915873295982,0.723256331137679,
1.85908623411803));
#28814=CARTESIAN_POINT('Ctrl Pts',(-11.5805658325193,-1.16798020743223,
1.61713437334789));
#28815=CARTESIAN_POINT('Ctrl Pts',(-11.4695443354405,-1.99220091274483,
-0.102160998798728));
#28816=CARTESIAN_POINT('Ctrl Pts',(-11.3585228383617,-0.996433656445175,
-1.72812653319149));
#28817=CARTESIAN_POINT('Ctrl Pts',(-11.2475013412829,0.909631977730951,
-1.77535095446118));
#28818=CARTESIAN_POINT('Ctrl Pts',(-11.136479844204,1.98469746609999,-0.200692088716223));
#28819=CARTESIAN_POINT('Ctrl Pts',(-11.0254583471252,1.24662981481611,1.5573103259237));
#28820=CARTESIAN_POINT('Ctrl Pts',(-10.9144368500464,-0.630304524580239,
1.89262187261763));
#28821=CARTESIAN_POINT('Ctrl Pts',(-10.8034153529676,-1.93142011018166,
0.498916530496676));
#28822=CARTESIAN_POINT('Ctrl Pts',(-10.6923938558887,-1.46807442741462,
-1.35057721807686));
#28823=CARTESIAN_POINT('Ctrl Pts',(-10.5813723588099,0.336440094073728,
-1.96624245949391));
#28824=CARTESIAN_POINT('Ctrl Pts',(-10.4703508617311,1.83359760297329,-0.785634251282103));
#28825=CARTESIAN_POINT('Ctrl Pts',(-10.3593293646522,1.65566022435232,1.11269518194096));
#28826=CARTESIAN_POINT('Ctrl Pts',(-10.2483078675734,-0.0348162047050451,
1.99451477264695));
#28827=CARTESIAN_POINT('Ctrl Pts',(-10.1372863704946,-1.69348606594746,
1.05423256013973));
#28828=CARTESIAN_POINT('Ctrl Pts',(-10.0262648734158,-1.80506083579367,
-0.849150590590889));
#28829=CARTESIAN_POINT('Ctrl Pts',(-9.91524337633695,-0.267610665381181,
-1.97678675587207));
#28830=CARTESIAN_POINT('Ctrl Pts',(-9.80422187925813,1.51431695019108,-1.29851666172637));
#28831=CARTESIAN_POINT('Ctrl Pts',(-9.69320038217929,1.91283057283628,0.56602168336543));
#28832=CARTESIAN_POINT('Ctrl Pts',(-9.58217888510047,0.563865518559531,
1.9134672778484));
#28833=CARTESIAN_POINT('Ctrl Pts',(-9.47115738802165,-1.30022250809489,
1.51285252944907));
#28834=CARTESIAN_POINT('Ctrl Pts',(-9.36013589094282,-1.97648389687789,
-0.269838380886415));
#28835=CARTESIAN_POINT('Ctrl Pts',(-9.24911439386399,-0.847115705016716,
-1.80601670222925));
#28836=CARTESIAN_POINT('Ctrl Pts',(-9.13809289678518,1.05614048948519,-1.69229684538114));
#28837=CARTESIAN_POINT('Ctrl Pts',(-9.02707139970634,1.99455274463459,-0.0325683172365964));
#28838=CARTESIAN_POINT('Ctrl Pts',(-8.91604990262752,1.11082850701714,1.65691320666324));
#28839=CARTESIAN_POINT('Ctrl Pts',(-8.80502840554869,-0.787700260230558,
1.83271101007488));
#28840=CARTESIAN_POINT('Ctrl Pts',(-8.69400690846987,-1.96662038669951,
0.334223878612652));
#28841=CARTESIAN_POINT('Ctrl Pts',(-8.58298541139104,-1.34892180570934,
-1.46959562754482));
#28842=CARTESIAN_POINT('Ctrl Pts',(-8.47196391431221,0.501092969818087,
-1.93085659281467));
#28843=CARTESIAN_POINT('Ctrl Pts',(-8.3609424172334,1.8933310387477,-0.62817109463232));
#28844=CARTESIAN_POINT('Ctrl Pts',(-8.24992092015456,1.55590435558153,1.24838414868958));
#28845=CARTESIAN_POINT('Ctrl Pts',(-8.13889942307575,-0.20292876227853,
1.98447002090158));
#28846=CARTESIAN_POINT('Ctrl Pts',(-8.0278779259969,-1.77637500372011,0.907630537485031));
#28847=CARTESIAN_POINT('Ctrl Pts',(-7.9168564289181,-1.72700243135777,-0.998380663124713));
#28848=CARTESIAN_POINT('Ctrl Pts',(-7.80583493183926,-0.0999156763351079,
-1.99231478537893));
#28849=CARTESIAN_POINT('Ctrl Pts',(-7.69481343476044,1.61844968765863,-1.16615691694329));
#28850=CARTESIAN_POINT('Ctrl Pts',(-7.58379193768161,1.85826992642422,0.725351105992336));
#28851=CARTESIAN_POINT('Ctrl Pts',(-7.47277044060279,0.400455717839537,
1.95420995915655));
#28852=CARTESIAN_POINT('Ctrl Pts',(-7.36174894352396,-1.42319738830023,
1.39778773079191));
#28853=CARTESIAN_POINT('Ctrl Pts',(-7.25072744644514,-1.94667936353946,
-0.435592472371381));
#28854=CARTESIAN_POINT('Ctrl Pts',(-7.13970594936631,-0.691759881327519,
-1.87103436980797));
#28855=CARTESIAN_POINT('Ctrl Pts',(-7.02868445228748,1.19512129123814,-1.59718078051493));
#28856=CARTESIAN_POINT('Ctrl Pts',(-6.91766295520866,1.99019171881064,0.135787587041479));
#28857=CARTESIAN_POINT('Ctrl Pts',(-6.80664145812983,0.967109696816501,
1.74470633080198));
#28858=CARTESIAN_POINT('Ctrl Pts',(-6.69561996105101,-0.939481611065625,
1.75973738065841));
#28859=CARTESIAN_POINT('Ctrl Pts',(-6.58459846397218,-1.98780344855593,
0.16714902430503));
#28860=CARTESIAN_POINT('Ctrl Pts',(-6.47357696689336,-1.22015465613688,
-1.57813939863514));
#28861=CARTESIAN_POINT('Ctrl Pts',(-6.36255546981452,0.662174272842673,
-1.88170842024004));
#28862=CARTESIAN_POINT('Ctrl Pts',(-6.25153397273571,1.93956963445295,-0.466230607666484));
#28863=CARTESIAN_POINT('Ctrl Pts',(-6.14051247565688,1.44505867736286,1.37517517625766));
#28864=CARTESIAN_POINT('Ctrl Pts',(-6.02949097857805,-0.369594931905942,
1.96028083006656));
#28865=CARTESIAN_POINT('Ctrl Pts',(-5.91846948149923,-1.84660271316689,
0.754559319166941));
#28866=CARTESIAN_POINT('Ctrl Pts',(-5.8074479844204,-1.63663470481537,-1.14049471257472));
#28867=CARTESIAN_POINT('Ctrl Pts',(-5.69642648734157,0.0684914681898172,
-1.99364246172733));
#28868=CARTESIAN_POINT('Ctrl Pts',(-5.58540499026275,1.71104681975768,-1.02548531291975));
#28869=CARTESIAN_POINT('Ctrl Pts',(-5.47438349318392,1.79046434030052,0.879510541454284));
#28870=CARTESIAN_POINT('Ctrl Pts',(-5.3633619961051,0.234191642955949,1.98102388193242));
#28871=CARTESIAN_POINT('Ctrl Pts',(-5.25234049902627,-1.53602833659461,
1.27276010920966));
#28872=CARTESIAN_POINT('Ctrl Pts',(-5.14131900194745,-1.90299974647861,
-0.598241850190491));
#28873=CARTESIAN_POINT('Ctrl Pts',(-5.03029750486863,-0.531473494111017,
-1.92271611827498));
#28874=CARTESIAN_POINT('Ctrl Pts',(-4.91927600778979,1.32558378828978,-1.49068070579863));
#28875=CARTESIAN_POINT('Ctrl Pts',(-4.80825451071098,1.97164547212322,0.303175656465004));
#28876=CARTESIAN_POINT('Ctrl Pts',(-4.69723301363214,0.816497749377447,
1.82006394713993));
#28877=CARTESIAN_POINT('Ctrl Pts',(-4.58621151655333,-1.08456674563962,
1.6742211086561));
#28878=CARTESIAN_POINT('Ctrl Pts',(-4.47519001947449,-1.99481831210039,
-0.0011171955401132));
#28879=CARTESIAN_POINT('Ctrl Pts',(-4.36416852239567,-1.08269077492733,
-1.67543487856269));
#28880=CARTESIAN_POINT('Ctrl Pts',(-4.25314702531684,0.818535885687912,
-1.81914824856525));
#28881=CARTESIAN_POINT('Ctrl Pts',(-4.14212552823802,1.97198382149198,-0.300967031733712));
#28882=CARTESIAN_POINT('Ctrl Pts',(-4.03110403115918,1.32391324947435,1.49216455335334));
#28883=CARTESIAN_POINT('Ctrl Pts',(-3.92008253408037,-0.533626789628149,
1.92211961017187));
#28884=CARTESIAN_POINT('Ctrl Pts',(-3.80906103700153,-1.90366864172245,
0.596109930246183));
#28885=CARTESIAN_POINT('Ctrl Pts',(-3.69803953992272,-1.53460175801352,
-1.27447981181542));
#28886=CARTESIAN_POINT('Ctrl Pts',(-3.58701804284388,0.236410435324478,
-1.9807603218156));
#28887=CARTESIAN_POINT('Ctrl Pts',(-3.47599654576507,1.79144835440527,-0.877504495662993));
#28888=CARTESIAN_POINT('Ctrl Pts',(-3.36497504868623,1.70989710319601,1.02740120836059));
#28889=CARTESIAN_POINT('Ctrl Pts',(-3.25395355160742,0.0662583518974708,
1.99371792818321));
#28890=CARTESIAN_POINT('Ctrl Pts',(-3.14293205452858,-1.63791114303142,
1.13866080723203));
#28891=CARTESIAN_POINT('Ctrl Pts',(-3.03191055744976,-1.84575637505747,
-0.756627220383344));
#28892=CARTESIAN_POINT('Ctrl Pts',(-2.92088906037093,-0.36739899491419,
-1.96069358250483));
#28893=CARTESIAN_POINT('Ctrl Pts',(-2.80986756329211,1.44659810052314,-1.37355570763518));
#28894=CARTESIAN_POINT('Ctrl Pts',(-2.69884606621328,1.9390461945082,0.468402822060808));
#28895=CARTESIAN_POINT('Ctrl Pts',(-2.58782456913446,0.660066160467937,
1.88244893865578));
#28896=CARTESIAN_POINT('Ctrl Pts',(-2.47680307205563,-1.22192155893126,
1.57677171821057));
#28897=CARTESIAN_POINT('Ctrl Pts',(-2.36578157497681,-1.98761498089598,
-0.169375455078507));
#28898=CARTESIAN_POINT('Ctrl Pts',(-2.25476007789798,-0.937509940151467,
-1.76078858256476));
#28899=CARTESIAN_POINT('Ctrl Pts',(-2.14373858081916,0.969063321888055,
-1.74362198881325));
#28900=CARTESIAN_POINT('Ctrl Pts',(-2.03271708374032,1.99034258258444,-0.133558275957203));
#28901=CARTESIAN_POINT('Ctrl Pts',(-1.92169558666151,1.19333151158385,1.59851839679231));
#28902=CARTESIAN_POINT('Ctrl Pts',(-1.81067408958268,-0.693855126354071,
1.87025842209972));
#28903=CARTESIAN_POINT('Ctrl Pts',(-1.69965259250386,-1.94716616503712,
0.433411606672418));
#28904=CARTESIAN_POINT('Ctrl Pts',(-1.58863109542502,-1.42163061521549,
-1.39938074047672));
#28905=CARTESIAN_POINT('Ctrl Pts',(-1.4776095983462,0.402643948884029,-1.95376062705992));
#28906=CARTESIAN_POINT('Ctrl Pts',(-1.36658810126737,1.85908202905433,-0.723268364827023));
#28907=CARTESIAN_POINT('Ctrl Pts',(-1.25556660418855,1.61714093219328,1.16796740173245));
#28908=CARTESIAN_POINT('Ctrl Pts',(-1.14454510710972,-0.102144286227503,
1.9922046737893));
#28909=CARTESIAN_POINT('Ctrl Pts',(-1.0335236100309,-1.72812517579298,0.99643981569525));
#28910=CARTESIAN_POINT('Ctrl Pts',(-0.922502112952074,-1.77534670427177,
-0.909608623609972));
#28911=CARTESIAN_POINT('Ctrl Pts',(-0.811480615873249,-0.200725913054806,
-1.98471711706149));
#28912=CARTESIAN_POINT('Ctrl Pts',(-0.700459118794423,1.55733989746973,
-1.24660056130178));
#28913=CARTESIAN_POINT('Ctrl Pts',(-0.589437621715598,1.89255353070104,
0.630215218936021));
#28914=CARTESIAN_POINT('Ctrl Pts',(-0.478416124636772,0.499068295829763,
1.93156167278018));
#28915=CARTESIAN_POINT('Ctrl Pts',(-0.367394627557947,-1.3508306443166,
1.4678076366454));
#28916=CARTESIAN_POINT('Ctrl Pts',(-0.25637313047912,-1.96574101035108,
-0.335899396150099));
#28917=CARTESIAN_POINT('Ctrl Pts',(-0.145351633400296,-0.78662434608425,
-1.83460887189422));
#28918=CARTESIAN_POINT('Ctrl Pts',(-0.0343301363214683,1.11470387286102,
-1.65361507057469));
#28919=CARTESIAN_POINT('Ctrl Pts',(0.0396841950644149,1.69786070835726,
-0.531282356819573));
#28920=CARTESIAN_POINT('Ctrl Pts',(0.0766913607573572,1.68807636917386,
0.0294553268735078));
#28921=CARTESIAN_POINT('Ctrl Pts',(-15.7226913607574,-0.802959149489957,
1.63459616787393));
#28922=CARTESIAN_POINT('Ctrl Pts',(-15.6856841950644,-1.34593201830381,
1.36787277679565));
#28923=CARTESIAN_POINT('Ctrl Pts',(-15.6116698636785,-2.13591160079902,
0.255552036473978));
#28924=CARTESIAN_POINT('Ctrl Pts',(-15.5006483665997,-1.37338031410794,
-1.65832692067852));
#28925=CARTESIAN_POINT('Ctrl Pts',(-15.3896268695209,0.645581844690631,
-2.05197493134485));
#28926=CARTESIAN_POINT('Ctrl Pts',(-15.278605372442,2.07385877578268,-0.573662929393826));
#28927=CARTESIAN_POINT('Ctrl Pts',(-15.1675838753632,1.60802441494309,1.43009236470613));
#28928=CARTESIAN_POINT('Ctrl Pts',(-15.0565623782844,-0.327080723815373,
2.12665944556502));
#28929=CARTESIAN_POINT('Ctrl Pts',(-14.9455408812056,-1.96324796184311,
0.880780288573345));
#28930=CARTESIAN_POINT('Ctrl Pts',(-14.8345193841267,-1.80594633577617,
-1.1699395550268));
#28931=CARTESIAN_POINT('Ctrl Pts',(-14.7234978870479,0.00122541408525625,
-2.15174944545788));
#28932=CARTESIAN_POINT('Ctrl Pts',(-14.6124763899691,1.8072586404345,-1.1678695140996));
#28933=CARTESIAN_POINT('Ctrl Pts',(-14.5014548928903,1.9622691127951,0.882953885847407));
#28934=CARTESIAN_POINT('Ctrl Pts',(-14.3904333958115,0.32463075438992,2.1271339690297));
#28935=CARTESIAN_POINT('Ctrl Pts',(-14.2794118987326,-1.60957335547925,
1.42806507104192));
#28936=CARTESIAN_POINT('Ctrl Pts',(-14.1683904016538,-2.07334282239369,
-0.575626034370439));
#28937=CARTESIAN_POINT('Ctrl Pts',(-14.057368904575,-0.642995851091954,
-2.05344807925839));
#28938=CARTESIAN_POINT('Ctrl Pts',(-13.9463474074961,1.37476371604704,-1.65533057206896));
#28939=CARTESIAN_POINT('Ctrl Pts',(-13.8353259104173,2.13659925589318,0.255025435270031));
#28940=CARTESIAN_POINT('Ctrl Pts',(-13.7243044133385,0.946530687964835,
1.93240099710466));
#28941=CARTESIAN_POINT('Ctrl Pts',(-13.6132829162597,-1.10824702172465,
1.84441936227157));
#28942=CARTESIAN_POINT('Ctrl Pts',(-13.5022614191808,-2.15057856485875,
0.0714564641882035));
#28943=CARTESIAN_POINT('Ctrl Pts',(-13.391239922102,-1.22823520722557,-1.76678590031394));
#28944=CARTESIAN_POINT('Ctrl Pts',(-13.2802184250232,0.816170317961378,
-1.99096966239773));
#28945=CARTESIAN_POINT('Ctrl Pts',(-13.1691969279444,2.11495820239117,-0.396290266790191));
#28946=CARTESIAN_POINT('Ctrl Pts',(-13.0581754308655,1.48161241110288,1.56042264506286));
#28947=CARTESIAN_POINT('Ctrl Pts',(-12.9471539337867,-0.505269929782832,
2.09160141331823));
#28948=CARTESIAN_POINT('Ctrl Pts',(-12.8361324367079,-2.03055967606441,
0.711984251270878));
#28949=CARTESIAN_POINT('Ctrl Pts',(-12.7251109396291,-1.70081856536528,
-1.31807070344234));
#28950=CARTESIAN_POINT('Ctrl Pts',(-12.6140894425502,0.182716288572517,
-2.14399368710076));
#28951=CARTESIAN_POINT('Ctrl Pts',(-12.5030679454714,1.899329501586,-1.01125744323421));
#28952=CARTESIAN_POINT('Ctrl Pts',(-12.3920464483926,1.88079802813469,1.04531954416464));
#28953=CARTESIAN_POINT('Ctrl Pts',(-12.2810249513138,0.144051415096028,
2.14693813650445));
#28954=CARTESIAN_POINT('Ctrl Pts',(-12.1700034542349,-1.72429429504063,
1.28720758085167));
#28955=CARTESIAN_POINT('Ctrl Pts',(-12.0589819571561,-2.01739985786644,
-0.748459742131278));
#28956=CARTESIAN_POINT('Ctrl Pts',(-11.9479604600773,-0.467496800638412,
-2.10036685212841));
#28957=CARTESIAN_POINT('Ctrl Pts',(-11.8369389629985,1.50949096667834,-1.53347031064656));
#28958=CARTESIAN_POINT('Ctrl Pts',(-11.7259174659196,2.10747354935533,0.434337899435756));
#28959=CARTESIAN_POINT('Ctrl Pts',(-11.6148959688408,0.780160111583563,
2.00535392697016));
#28960=CARTESIAN_POINT('Ctrl Pts',(-11.503874471762,-1.25987361565765,1.74436597211969));
#28961=CARTESIAN_POINT('Ctrl Pts',(-11.3928529746832,-2.14894169531716,
-0.110198739770348));
#28962=CARTESIAN_POINT('Ctrl Pts',(-11.2818314776043,-1.07483026297892,
-1.86409068392728));
#28963=CARTESIAN_POINT('Ctrl Pts',(-11.1708099805255,0.981199271536627,
-1.91503059026627));
#28964=CARTESIAN_POINT('Ctrl Pts',(-11.0597884834467,2.14084789852661,-0.216481979605357));
#28965=CARTESIAN_POINT('Ctrl Pts',(-10.9487669863679,1.34471115365209,1.67983513636409));
#28966=CARTESIAN_POINT('Ctrl Pts',(-10.837745489289,-0.679895117481559,
2.04152805548794));
#28967=CARTESIAN_POINT('Ctrl Pts',(-10.7267239922102,-2.08337882961056,
0.538169884376828));
#28968=CARTESIAN_POINT('Ctrl Pts',(-10.6157024951314,-1.58357840753797,
-1.45683684717925));
#28969=CARTESIAN_POINT('Ctrl Pts',(-10.5046809980526,0.362910257447538,
-2.12094090374037));
#28970=CARTESIAN_POINT('Ctrl Pts',(-10.3936595009737,1.9778599217857,-0.847445751605094));
#28971=CARTESIAN_POINT('Ctrl Pts',(-10.2826380038949,1.78592292907185,1.20023891935526));
#28972=CARTESIAN_POINT('Ctrl Pts',(-10.1716165068161,-0.0375554460821274,
2.15143760322934));
#28973=CARTESIAN_POINT('Ctrl Pts',(-10.0605950097372,-1.82672480183691,
1.13717662237383));
#28974=CARTESIAN_POINT('Ctrl Pts',(-9.94957351265842,-1.94707796176875,
-0.915959378419207));
#28975=CARTESIAN_POINT('Ctrl Pts',(-9.83855201557959,-0.288665522272483,
-2.13231479579607));
#28976=CARTESIAN_POINT('Ctrl Pts',(-9.72753051850077,1.63345916236307,-1.40068031220968));
#28977=CARTESIAN_POINT('Ctrl Pts',(-9.61650902142194,2.06332671958362,0.610554682540373));
#28978=CARTESIAN_POINT('Ctrl Pts',(-9.50548752434312,0.608228876732484,
2.06401351876105));
#28979=CARTESIAN_POINT('Ctrl Pts',(-9.39446602726429,-1.40252036978803,
1.63187952510266));
#28980=CARTESIAN_POINT('Ctrl Pts',(-9.28344453018547,-2.1319881087053,-0.291068508188133));
#28981=CARTESIAN_POINT('Ctrl Pts',(-9.17242303310663,-0.913764393752982,
-1.94810903309566));
#28982=CARTESIAN_POINT('Ctrl Pts',(-9.06140153602782,1.1392346622512,-1.82544201673049));
#28983=CARTESIAN_POINT('Ctrl Pts',(-8.95038003894899,2.15147856274651,-0.0351307011297477));
#28984=CARTESIAN_POINT('Ctrl Pts',(-8.83935854187017,1.19822537968178,1.78727449251818));
#28985=CARTESIAN_POINT('Ctrl Pts',(-8.72833704479134,-0.849674308345434,
1.97690357424366));
#28986=CARTESIAN_POINT('Ctrl Pts',(-8.61731554771251,-2.12134856519896,
0.360519676367277));
#28987=CARTESIAN_POINT('Ctrl Pts',(-8.5062940506337,-1.4550511916077,-1.58521929142964));
#28988=CARTESIAN_POINT('Ctrl Pts',(-8.39527255355485,0.540517559842268,
-2.08277097627699));
#28989=CARTESIAN_POINT('Ctrl Pts',(-8.28425105647605,2.04229301682093,-0.677593835246537));
#28990=CARTESIAN_POINT('Ctrl Pts',(-8.1732295593972,1.67831854821712,1.34660351359635));
#28991=CARTESIAN_POINT('Ctrl Pts',(-8.06220806231839,-0.218894628372896,
2.14060255857764));
#28992=CARTESIAN_POINT('Ctrl Pts',(-7.95118656523956,-1.91613520884992,
0.979040363583317));
#28993=CARTESIAN_POINT('Ctrl Pts',(-7.84016506816073,-1.86287814091277,
-1.07693045468546));
#28994=CARTESIAN_POINT('Ctrl Pts',(-7.7291435710819,-0.107776761630186,
-2.14906452713085));
#28995=CARTESIAN_POINT('Ctrl Pts',(-7.61812207400309,1.74578477167283,-1.25790687378474));
#28996=CARTESIAN_POINT('Ctrl Pts',(-7.50710057692426,2.00447339447557,0.78241969745096));
#28997=CARTESIAN_POINT('Ctrl Pts',(-7.39607907984543,0.431962451020007,
2.10796172001022));
#28998=CARTESIAN_POINT('Ctrl Pts',(-7.2850575827666,-1.53517056880124,1.50776175067752));
#28999=CARTESIAN_POINT('Ctrl Pts',(-7.17403608568778,-2.09983863824241,
-0.469863666890626));
#29000=CARTESIAN_POINT('Ctrl Pts',(-7.06301458860895,-0.74618560940433,
-2.01824210847894));
#29001=CARTESIAN_POINT('Ctrl Pts',(-6.95199309153013,1.28915008384591,-1.7228424865436));
#29002=CARTESIAN_POINT('Ctrl Pts',(-6.8409715944513,2.1467744236371,0.146470973702092));
#29003=CARTESIAN_POINT('Ctrl Pts',(-6.72995009737248,1.04319917641796,1.88197493353141));
#29004=CARTESIAN_POINT('Ctrl Pts',(-6.61892860029365,-1.01339739033702,
1.8981885842502));
#29005=CARTESIAN_POINT('Ctrl Pts',(-6.50790710321483,-2.1441982509744,0.180299840926073));
#29006=CARTESIAN_POINT('Ctrl Pts',(-6.396885606136,-1.31615300371251,-1.70230298212104));
#29007=CARTESIAN_POINT('Ctrl Pts',(-6.28586410905717,0.714272288188727,
-2.02975596327374));
#29008=CARTESIAN_POINT('Ctrl Pts',(-6.17484261197835,2.09216953560388,-0.502912324775098));
#29009=CARTESIAN_POINT('Ctrl Pts',(-6.06382111489953,1.55875184279803,1.48337010374802));
#29010=CARTESIAN_POINT('Ctrl Pts',(-5.95279961782069,-0.398673624969019,
2.11451023002342));
#29011=CARTESIAN_POINT('Ctrl Pts',(-5.84177812074189,-1.9918882375888,0.813925930951356));
#29012=CARTESIAN_POINT('Ctrl Pts',(-5.73075662366303,-1.7654005349968,-1.23022563912181));
#29013=CARTESIAN_POINT('Ctrl Pts',(-5.61973512658423,0.0738801848874695,
-2.15049666133214));
#29014=CARTESIAN_POINT('Ctrl Pts',(-5.50871362950539,1.8456671865244,-1.10616762233703));
#29015=CARTESIAN_POINT('Ctrl Pts',(-5.39769213242658,1.93133305493226,0.948707965100779));
#29016=CARTESIAN_POINT('Ctrl Pts',(-5.28667063534773,0.252617184854861,
2.13688528705583));
#29017=CARTESIAN_POINT('Ctrl Pts',(-5.17564913826893,-1.65687873977979,
1.37289730635085));
#29018=CARTESIAN_POINT('Ctrl Pts',(-5.06462764119009,-2.05272243136938,
-0.645309841760259));
#29019=CARTESIAN_POINT('Ctrl Pts',(-4.95360614411127,-0.573288338613145,
-2.07399003202278));
#29020=CARTESIAN_POINT('Ctrl Pts',(-4.84258464703244,1.42987700440694,-1.60796328452731));
#29021=CARTESIAN_POINT('Ctrl Pts',(-4.73156314995361,2.12676901025572,0.327028667146397));
#29022=CARTESIAN_POINT('Ctrl Pts',(-4.62054165287479,0.880737503203102,
1.9632614758537));
#29023=CARTESIAN_POINT('Ctrl Pts',(-4.50952015579596,-1.16989741654532,
1.80594413171622));
#29024=CARTESIAN_POINT('Ctrl Pts',(-4.39849865871714,-2.151765024316,-0.00120509335308468));
#29025=CARTESIAN_POINT('Ctrl Pts',(-4.28747716163831,-1.16787384971678,
-1.80725339763617));
#29026=CARTESIAN_POINT('Ctrl Pts',(-4.17645566455949,0.882935994364434,
-1.96227373268238));
#29027=CARTESIAN_POINT('Ctrl Pts',(-4.06543416748067,2.12713398000424,-0.324646274013261));
#29028=CARTESIAN_POINT('Ctrl Pts',(-3.95441267040183,1.42807503228097,1.60956387704757));
#29029=CARTESIAN_POINT('Ctrl Pts',(-3.84339117332301,-0.575611049384669,
2.07334659233446));
#29030=CARTESIAN_POINT('Ctrl Pts',(-3.73236967624418,-2.05344395341572,
0.643010188331699));
#29031=CARTESIAN_POINT('Ctrl Pts',(-3.62134817916536,-1.65533992199544,
-1.37475231033633));
#29032=CARTESIAN_POINT('Ctrl Pts',(-3.51032668208653,0.255010545586425,
-2.13660099076793));
#29033=CARTESIAN_POINT('Ctrl Pts',(-3.39930518500771,1.93239448850803,-0.946544089250699));
#29034=CARTESIAN_POINT('Ctrl Pts',(-3.28828368792888,1.84442701348695,1.10823425505983));
#29035=CARTESIAN_POINT('Ctrl Pts',(-3.17726219085005,0.0714713732659194,
2.15057806527719));
#29036=CARTESIAN_POINT('Ctrl Pts',(-3.06624069377123,-1.76677739979312,
1.22824744724822));
#29037=CARTESIAN_POINT('Ctrl Pts',(-2.9552191966924,-1.99097531196969,-0.81615652883798));
#29038=CARTESIAN_POINT('Ctrl Pts',(-2.84419769961358,-0.396304917811199,
-2.11495545666636));
#29039=CARTESIAN_POINT('Ctrl Pts',(-2.73317620253476,1.56041238345669,-1.4816232198746));
#29040=CARTESIAN_POINT('Ctrl Pts',(-2.62215470545592,2.09160491287177,0.505255442908033));
#29041=CARTESIAN_POINT('Ctrl Pts',(-2.5111332083771,0.711998315442568,2.03055474360234));
#29042=CARTESIAN_POINT('Ctrl Pts',(-2.40011171129828,-1.31805892146514,
1.70082769643504));
#29043=CARTESIAN_POINT('Ctrl Pts',(-2.28909021421945,-2.14399495520735,
-0.182701441030875));
#29044=CARTESIAN_POINT('Ctrl Pts',(-2.17806871714062,-1.01127059388303,
-1.89932249177543));
#29045=CARTESIAN_POINT('Ctrl Pts',(-2.0670472200618,1.04530650723304,-1.88080527855502));
#29046=CARTESIAN_POINT('Ctrl Pts',(-1.95602572298297,2.14693715694967,-0.144066266671712));
#29047=CARTESIAN_POINT('Ctrl Pts',(-1.84500422590415,1.28721948934618,1.72428534271959));
#29048=CARTESIAN_POINT('Ctrl Pts',(-1.73398272882532,-0.748445702435426,
2.01740511138042));
#29049=CARTESIAN_POINT('Ctrl Pts',(-1.6229612317465,-2.10036373991713,0.467511216792655));
#29050=CARTESIAN_POINT('Ctrl Pts',(-1.51193973466767,-1.53348052640274,
-1.50948009389823));
#29051=CARTESIAN_POINT('Ctrl Pts',(-1.40091823758885,0.434322845948246,
-2.10747703572397));
#29052=CARTESIAN_POINT('Ctrl Pts',(-1.28989674051002,2.00534939106384,-0.780173092049846));
#29053=CARTESIAN_POINT('Ctrl Pts',(-1.1788752434312,1.74437304699665,1.25985980244131));
#29054=CARTESIAN_POINT('Ctrl Pts',(-1.06785374635237,-0.110180712300874,
2.14894575227006));
#29055=CARTESIAN_POINT('Ctrl Pts',(-0.956832249273545,-1.86408921973246,
1.07483690682153));
#29056=CARTESIAN_POINT('Ctrl Pts',(-0.845810752194719,-1.91502600568388,
-0.981174079978886));
#29057=CARTESIAN_POINT('Ctrl Pts',(-0.734789255115894,-0.216518465148069,
-2.14086909557066));
#29058=CARTESIAN_POINT('Ctrl Pts',(-0.623767758037068,1.67986703451646,
-1.34467959855327));
#29059=CARTESIAN_POINT('Ctrl Pts',(-0.512746260958242,2.04145433662096,
0.67979878551963));
#29060=CARTESIAN_POINT('Ctrl Pts',(-0.401724763879417,0.538333590180839,
2.08353152995745));
#29061=CARTESIAN_POINT('Ctrl Pts',(-0.290703266800591,-1.45711021228504,
1.58329062641899));
#29062=CARTESIAN_POINT('Ctrl Pts',(-0.179681769721765,-2.12040000198483,
-0.362327018927154));
#29063=CARTESIAN_POINT('Ctrl Pts',(-0.0686602726429408,-0.84851374429049,
-1.97895075451018));
#29064=CARTESIAN_POINT('Ctrl Pts',(0.0423612244358866,1.20240564844544,
-1.78371686832869));
#29065=CARTESIAN_POINT('Ctrl Pts',(0.11637555582177,1.83144362884697,-0.573082163175473));
#29066=CARTESIAN_POINT('Ctrl Pts',(0.153382721514712,1.82088948528754,0.0317727894123157));
#29067=CARTESIAN_POINT('Ctrl Pts',(-15.646,-0.861525859670559,1.75382131162753));
#29068=CARTESIAN_POINT('Ctrl Pts',(-15.6089928343071,-1.44410240528908,
1.46764349182322));
#29069=CARTESIAN_POINT('Ctrl Pts',(-15.5349785029212,-2.29170198661735,
0.274191642319117));
#29070=CARTESIAN_POINT('Ctrl Pts',(-15.4239570058423,-1.47355274115507,
-1.7792829521401));
#29071=CARTESIAN_POINT('Ctrl Pts',(-15.3129355087636,0.692669675771291,
-2.20164309463595));
#29072=CARTESIAN_POINT('Ctrl Pts',(-15.2019140116847,2.22512311588507,-0.615505096020252));
#29073=CARTESIAN_POINT('Ctrl Pts',(-15.0908925146059,1.72531145243826,1.53440128890039));
#29074=CARTESIAN_POINT('Ctrl Pts',(-14.979871017527,-0.350937531436932,
2.28177499220319));
#29075=CARTESIAN_POINT('Ctrl Pts',(-14.8688495204482,-2.10644450486397,
0.945023163103684));
#29076=CARTESIAN_POINT('Ctrl Pts',(-14.7578280233694,-1.93766951959731,
-1.25527329945402));
#29077=CARTESIAN_POINT('Ctrl Pts',(-14.6468065262906,0.00131479406382864,
-2.3086950213735));
#29078=CARTESIAN_POINT('Ctrl Pts',(-14.5357850292118,1.93907754191032,-1.25305227265524));
#29079=CARTESIAN_POINT('Ctrl Pts',(-14.4247635321329,2.10539425994415,0.947355299503518));
#29080=CARTESIAN_POINT('Ctrl Pts',(-14.3137420350541,0.348308864689988,
2.28228412674149));
#29081=CARTESIAN_POINT('Ctrl Pts',(-14.2027205379753,-1.72697337051695,
1.53222612728979));
#29082=CARTESIAN_POINT('Ctrl Pts',(-14.0916990408964,-2.22456952958211,
-0.617611387110731));
#29083=CARTESIAN_POINT('Ctrl Pts',(-13.9806775438176,-0.689895063439384,
-2.20322369188481));
#29084=CARTESIAN_POINT('Ctrl Pts',(-13.8696560467388,1.47503704648443,-1.7760680540804));
#29085=CARTESIAN_POINT('Ctrl Pts',(-13.75863454966,2.29243979830618,0.273626631564544));
#29086=CARTESIAN_POINT('Ctrl Pts',(-13.6476130525811,1.01556930408161,2.0733476059353));
#29087=CARTESIAN_POINT('Ctrl Pts',(-13.5365915555023,-1.18908099960645,
1.97894871449363));
#29088=CARTESIAN_POINT('Ctrl Pts',(-13.4255700584235,-2.30743873839151,
0.0766683981095072));
#29089=CARTESIAN_POINT('Ctrl Pts',(-13.3145485613447,-1.31782095447173,
-1.89565277709167));
#29090=CARTESIAN_POINT('Ctrl Pts',(-13.2035270642658,0.875700632175267,
-2.13618818723813));
#29091=CARTESIAN_POINT('Ctrl Pts',(-13.092505567187,2.26922027682201,-0.425195121062348));
#29092=CARTESIAN_POINT('Ctrl Pts',(-12.9814840701082,1.5896791349657,1.67423767646352));
#29093=CARTESIAN_POINT('Ctrl Pts',(-12.8704625730294,-0.542123607282315,
2.24415987642929));
#29094=CARTESIAN_POINT('Ctrl Pts',(-12.7594410759505,-2.17866584077781,
0.763915380424621));
#29095=CARTESIAN_POINT('Ctrl Pts',(-12.6484195788717,-1.82487387758237,
-1.41420892533704));
#29096=CARTESIAN_POINT('Ctrl Pts',(-12.5373980817929,0.196043357483676,
-2.30037356891822));
#29097=CARTESIAN_POINT('Ctrl Pts',(-12.426376584714,2.03786392208238,-1.08501713777596));
#29098=CARTESIAN_POINT('Ctrl Pts',(-12.3153550876352,2.01798078904102,1.12156368040506));
#29099=CARTESIAN_POINT('Ctrl Pts',(-12.2043335905564,0.154558322557508,
2.30353278231703));
#29100=CARTESIAN_POINT('Ctrl Pts',(-12.0933120934776,-1.85006189393761,
1.38109469002517));
#29101=CARTESIAN_POINT('Ctrl Pts',(-11.9822905963987,-2.16454616396323,
-0.803051342248286));
#29102=CARTESIAN_POINT('Ctrl Pts',(-11.8712690993199,-0.501595359264648,
-2.25356465400873));
#29103=CARTESIAN_POINT('Ctrl Pts',(-11.7602476022411,1.61959111314513,-1.64531947671092));
#29104=CARTESIAN_POINT('Ctrl Pts',(-11.6492261051623,2.26118970372855,0.466017894480162));
#29105=CARTESIAN_POINT('Ctrl Pts',(-11.5382046080835,0.837063892029446,
2.15162161982229));
#29106=CARTESIAN_POINT('Ctrl Pts',(-11.4271831110046,-1.35176702388306,
1.87159757089149));
#29107=CARTESIAN_POINT('Ctrl Pts',(-11.3161616139258,-2.30568247788948,
-0.118236480741969));
#29108=CARTESIAN_POINT('Ctrl Pts',(-11.205140116847,-1.15322686951267,-2.00005483466307));
#29109=CARTESIAN_POINT('Ctrl Pts',(-11.0941186197681,1.05276656534231,-2.05471022607136));
#29110=CARTESIAN_POINT('Ctrl Pts',(-10.9830971226893,2.29699833095323,-0.232271870494488));
#29111=CARTESIAN_POINT('Ctrl Pts',(-10.8720756256105,1.44279249248807,1.80235994680447));
#29112=CARTESIAN_POINT('Ctrl Pts',(-10.7610541285317,-0.729485710382879,
2.19043423835826));
#29113=CARTESIAN_POINT('Ctrl Pts',(-10.6500326314528,-2.23533754903947,
0.577423238256977));
#29114=CARTESIAN_POINT('Ctrl Pts',(-10.539011134374,-1.69908238766131,-1.56309647628163));
#29115=CARTESIAN_POINT('Ctrl Pts',(-10.4279896372952,0.389380420821346,
-2.27563934798683));
#29116=CARTESIAN_POINT('Ctrl Pts',(-10.3169681402164,2.12212224059811,-0.909257251928086));
#29117=CARTESIAN_POINT('Ctrl Pts',(-10.2059466431375,1.91618563379138,1.28778265676956));
#29118=CARTESIAN_POINT('Ctrl Pts',(-10.0949251460587,-0.0402946874592114,
2.30836043381174));
#29119=CARTESIAN_POINT('Ctrl Pts',(-9.98390364897989,-1.95996353772636,
1.22012068460793));
#29120=CARTESIAN_POINT('Ctrl Pts',(-9.87288215190107,-2.08909508774384,
-0.982768166247527));
#29121=CARTESIAN_POINT('Ctrl Pts',(-9.76186065482224,-0.309720379163782,
-2.28784283572006));
#29122=CARTESIAN_POINT('Ctrl Pts',(-9.65083915774341,1.75260137453506,-1.50284396269299));
#29123=CARTESIAN_POINT('Ctrl Pts',(-9.53981766066459,2.21382286633095,0.655087681715316));
#29124=CARTESIAN_POINT('Ctrl Pts',(-9.42879616358576,0.652592234905436,
2.2145597596737));
#29125=CARTESIAN_POINT('Ctrl Pts',(-9.31777466650695,-1.50481823148118,
1.75090652075626));
#29126=CARTESIAN_POINT('Ctrl Pts',(-9.2067531694281,-2.28749232053271,-0.31229863548985));
#29127=CARTESIAN_POINT('Ctrl Pts',(-9.0957316723493,-0.980413082489249,
-2.09020136396206));
#29128=CARTESIAN_POINT('Ctrl Pts',(-8.98471017527046,1.22232883501721,-1.95858718807982));
#29129=CARTESIAN_POINT('Ctrl Pts',(-8.87368867819164,2.30840438085843,-0.0376930850229031));
#29130=CARTESIAN_POINT('Ctrl Pts',(-8.76266718111281,1.28562225234641,1.91763577837313));
#29131=CARTESIAN_POINT('Ctrl Pts',(-8.65164568403398,-0.911648356460311,
2.12109613841244));
#29132=CARTESIAN_POINT('Ctrl Pts',(-8.54062418695517,-2.27607674369842,
0.386815474121903));
#29133=CARTESIAN_POINT('Ctrl Pts',(-8.42960268987633,-1.56118057750606,
-1.70084295531445));
#29134=CARTESIAN_POINT('Ctrl Pts',(-8.31858119279751,0.57994214986645,-2.23468535973931));
#29135=CARTESIAN_POINT('Ctrl Pts',(-8.20755969571868,2.19125499489417,-0.727016575860756));
#29136=CARTESIAN_POINT('Ctrl Pts',(-8.09653819863985,1.80073274085271,1.44482287850311));
#29137=CARTESIAN_POINT('Ctrl Pts',(-7.98551670156104,-0.234860494467263,
2.29673509625371));
#29138=CARTESIAN_POINT('Ctrl Pts',(-7.87449520448219,-2.05589541397972,
1.0504501896816));
#29139=CARTESIAN_POINT('Ctrl Pts',(-7.76347370740339,-1.99875385046778,
-1.1554802462462));
#29140=CARTESIAN_POINT('Ctrl Pts',(-7.65245221032454,-0.115637846925265,
-2.30581426888278));
#29141=CARTESIAN_POINT('Ctrl Pts',(-7.54143071324574,1.87311985568703,-1.34965683062618));
#29142=CARTESIAN_POINT('Ctrl Pts',(-7.43040921616689,2.15067686252692,0.839488288909578));
#29143=CARTESIAN_POINT('Ctrl Pts',(-7.31938771908808,0.46346918420048,2.2617134808639));
#29144=CARTESIAN_POINT('Ctrl Pts',(-7.20836622200924,-1.64714374930225,
1.61773577056313));
#29145=CARTESIAN_POINT('Ctrl Pts',(-7.09734472493043,-2.25299791294537,
-0.504134861409866));
#29146=CARTESIAN_POINT('Ctrl Pts',(-6.98632322785159,-0.800611337481142,
-2.16544984714991));
#29147=CARTESIAN_POINT('Ctrl Pts',(-6.87530173077277,1.38317887645369,-1.84850419257227));
#29148=CARTESIAN_POINT('Ctrl Pts',(-6.76428023369394,2.30335712846357,0.157154360362701));
#29149=CARTESIAN_POINT('Ctrl Pts',(-6.65325873661513,1.11928865601943,2.01924353626084));
#29150=CARTESIAN_POINT('Ctrl Pts',(-6.54223723953629,-1.08731316960842,
2.03663978784199));
#29151=CARTESIAN_POINT('Ctrl Pts',(-6.43121574245748,-2.30059305339287,
0.193450657547119));
#29152=CARTESIAN_POINT('Ctrl Pts',(-6.32019424537864,-1.41215135128814,
-1.82646656560694));
#29153=CARTESIAN_POINT('Ctrl Pts',(-6.20917274829982,0.766370303534781,
-2.17780350630744));
#29154=CARTESIAN_POINT('Ctrl Pts',(-6.09815125122099,2.24476943675482,-0.539594041883711));
#29155=CARTESIAN_POINT('Ctrl Pts',(-5.98712975414218,1.6724450082332,1.59156503123837));
#29156=CARTESIAN_POINT('Ctrl Pts',(-5.87610825706333,-0.427752318032092,
2.26873962998029));
#29157=CARTESIAN_POINT('Ctrl Pts',(-5.76508675998452,-2.13717376201072,
0.873292542735772));
#29158=CARTESIAN_POINT('Ctrl Pts',(-5.65406526290569,-1.89416636517823,
-1.3199565656689));
#29159=CARTESIAN_POINT('Ctrl Pts',(-5.54304376582687,0.0792689015851208,
-2.30735086093694));
#29160=CARTESIAN_POINT('Ctrl Pts',(-5.43202226874804,1.98028755329112,-1.18684993175432));
#29161=CARTESIAN_POINT('Ctrl Pts',(-5.32100077166922,2.072201769564,1.01790538874728));
#29162=CARTESIAN_POINT('Ctrl Pts',(-5.20997927459039,0.271042726753771,
2.29274669217924));
#29163=CARTESIAN_POINT('Ctrl Pts',(-5.09895777751157,-1.77772914296497,
1.47303450349202));
#29164=CARTESIAN_POINT('Ctrl Pts',(-4.98793628043274,-2.20244511626014,
-0.692377833330026));
#29165=CARTESIAN_POINT('Ctrl Pts',(-4.87691478335391,-0.615103183115273,
-2.22526394577057));
#29166=CARTESIAN_POINT('Ctrl Pts',(-4.76589328627509,1.53417022052411,-1.725245863256));
#29167=CARTESIAN_POINT('Ctrl Pts',(-4.65487178919626,2.28189254838822,0.350881677827793));
#29168=CARTESIAN_POINT('Ctrl Pts',(-4.54385029211743,0.944977257028757,
2.10645900456747));
#29169=CARTESIAN_POINT('Ctrl Pts',(-4.43282879503862,-1.25522808745102,
1.93766715477633));
#29170=CARTESIAN_POINT('Ctrl Pts',(-4.32180729795978,-2.3087117365316,-0.00129299116605801));
#29171=CARTESIAN_POINT('Ctrl Pts',(-4.21078580088096,-1.25305692450623,
-1.93907191670966));
#29172=CARTESIAN_POINT('Ctrl Pts',(-4.09976430380213,0.947336103040959,
-2.10539921679951));
#29173=CARTESIAN_POINT('Ctrl Pts',(-3.98874280672331,2.28228413851649,-0.348325516292812));
#29174=CARTESIAN_POINT('Ctrl Pts',(-3.87772130964448,1.5322368150876,1.7269632007418));
#29175=CARTESIAN_POINT('Ctrl Pts',(-3.76669981256566,-0.617595309141191,
2.22457357449704));
#29176=CARTESIAN_POINT('Ctrl Pts',(-3.65567831548683,-2.20321926510898,
0.689910446417216));
#29177=CARTESIAN_POINT('Ctrl Pts',(-3.54465681840801,-1.77607808597735,
-1.47502480885725));
#29178=CARTESIAN_POINT('Ctrl Pts',(-3.43363532132918,0.273610655848373,
-2.29244165972025));
#29179=CARTESIAN_POINT('Ctrl Pts',(-3.32261382425035,2.07334062261079,-1.01558368283841));
#29180=CARTESIAN_POINT('Ctrl Pts',(-3.21159232717153,1.97895692377789,1.18906730175907));
#29181=CARTESIAN_POINT('Ctrl Pts',(-3.1005708300927,0.0766843946343644,
2.30743820237117));
#29182=CARTESIAN_POINT('Ctrl Pts',(-2.98954933301387,-1.89564365655482,
1.31783408726441));
#29183=CARTESIAN_POINT('Ctrl Pts',(-2.87852783593505,-2.13619424888191,
-0.875685837292615));
#29184=CARTESIAN_POINT('Ctrl Pts',(-2.76750633885622,-0.425210840708204,
-2.2692173308279));
#29185=CARTESIAN_POINT('Ctrl Pts',(-2.6564848417774,1.67422666639024,-1.58969073211401));
#29186=CARTESIAN_POINT('Ctrl Pts',(-2.54546334469857,2.24416363123536,0.542108063755256));
#29187=CARTESIAN_POINT('Ctrl Pts',(-2.43444184761975,0.763930470417198,
2.1786605485489));
#29188=CARTESIAN_POINT('Ctrl Pts',(-2.32342035054092,-1.41419628399901,
1.8248836746595));
#29189=CARTESIAN_POINT('Ctrl Pts',(-2.2123988534621,-2.30037492951871,-0.196027426983243));
#29190=CARTESIAN_POINT('Ctrl Pts',(-2.10137735638327,-1.0850312476146,-2.0378564009861));
#29191=CARTESIAN_POINT('Ctrl Pts',(-1.99035585930445,1.12154969257803,-2.0179885682968));
#29192=CARTESIAN_POINT('Ctrl Pts',(-1.87933436222562,2.3035317313149,-0.154574257386218));
#29193=CARTESIAN_POINT('Ctrl Pts',(-1.76831286514679,1.38110746710851,1.85005228864688));
#29194=CARTESIAN_POINT('Ctrl Pts',(-1.65729136806797,-0.803036278516782,
2.16455180066113));
#29195=CARTESIAN_POINT('Ctrl Pts',(-1.54626987098914,-2.25356131479715,
0.501610826912889));
#29196=CARTESIAN_POINT('Ctrl Pts',(-1.43524837391032,-1.64533043758998,
-1.61957944731974));
#29197=CARTESIAN_POINT('Ctrl Pts',(-1.32422687683149,0.46600174301246,-2.26119344438801));
#29198=CARTESIAN_POINT('Ctrl Pts',(-1.21320537975266,2.15161675307334,-0.837077819272669));
#29199=CARTESIAN_POINT('Ctrl Pts',(-1.10218388267384,1.87160516180001,1.35175220315016));
#29200=CARTESIAN_POINT('Ctrl Pts',(-0.991162385595015,-0.118217138374247,
2.30568683075082));
#29201=CARTESIAN_POINT('Ctrl Pts',(-0.88014088851619,-2.00005326367194,
1.1532339979478));
#29202=CARTESIAN_POINT('Ctrl Pts',(-0.769119391437363,-2.05470530709598,
-1.0527395363478));
#29203=CARTESIAN_POINT('Ctrl Pts',(-0.65809789435854,-0.23231101724133,
-2.29702107407985));
#29204=CARTESIAN_POINT('Ctrl Pts',(-0.547076397279713,1.80239417156319,
-1.44275863580475));
#29205=CARTESIAN_POINT('Ctrl Pts',(-0.436054900200888,2.19035514254088,
0.729382352103237));
#29206=CARTESIAN_POINT('Ctrl Pts',(-0.325033403122062,0.577598884531914,
2.23550138713472));
#29207=CARTESIAN_POINT('Ctrl Pts',(-0.214011906043236,-1.56338978025347,
1.69877361619258));
#29208=CARTESIAN_POINT('Ctrl Pts',(-0.10299040896441,-2.27505899361857,
-0.388754641704208));
#29209=CARTESIAN_POINT('Ctrl Pts',(0.00803108811441417,-0.910403142496731,
-2.12329263712614));
#29210=CARTESIAN_POINT('Ctrl Pts',(0.119052585193242,1.29010742402986,-1.9138186660827));
#29211=CARTESIAN_POINT('Ctrl Pts',(0.193066916579125,1.96502654933667,-0.614881969531372));
#29212=CARTESIAN_POINT('Ctrl Pts',(0.230074082272067,1.95370260140122,0.0340902519511237));
#29213=CARTESIAN_POINT('',(0.,-0.896933272146831,-1.73598004173895));
#29214=CARTESIAN_POINT('Ctrl Pts',(2.66453525910038E-15,-0.897777576978214,
-1.73914455526119));
#29215=CARTESIAN_POINT('Ctrl Pts',(2.42885616950946E-15,-0.854308595888035,
-1.75665132687895));
#29216=CARTESIAN_POINT('Ctrl Pts',(-1.52008741663672E-16,-0.810233059137786,
-1.77245732638827));
#29217=CARTESIAN_POINT('Ctrl Pts',(8.60422844084496E-16,-0.765604712779606,
-1.78648174433319));
#29218=CARTESIAN_POINT('Ctrl Pts',(2.41466958929901E-15,-0.697057735880828,
-1.80802257054201));
#29219=CARTESIAN_POINT('Ctrl Pts',(3.66730899670521E-15,-0.627206169701796,
-1.82536276747026));
#29220=CARTESIAN_POINT('Ctrl Pts',(4.13558076672871E-15,-0.556420062791459,
-1.83857524845937));
#29221=CARTESIAN_POINT('Ctrl Pts',(4.36243855997318E-15,-0.522127199044321,
-1.84497613459506));
#29222=CARTESIAN_POINT('Ctrl Pts',(8.67308952147876E-15,-0.48761501095824,
-1.85040746202521));
#29223=CARTESIAN_POINT('Ctrl Pts',(9.43689570931383E-15,-0.452926237145203,
-1.85487325410974));
#29224=CARTESIAN_POINT('Ctrl Pts',(9.76107763911627E-15,-0.438203295885635,
-1.85676866831182));
#29225=CARTESIAN_POINT('Ctrl Pts',(6.11879014245653E-15,-0.423448554037784,
-1.85849011749958));
#29226=CARTESIAN_POINT('Ctrl Pts',(5.93969318174459E-15,-0.408665330346609,
-1.8600377655215));
#29227=CARTESIAN_POINT('Ctrl Pts',(5.75276829265403E-15,-0.393235964946499,
-1.86165305778386));
#29228=CARTESIAN_POINT('Ctrl Pts',(4.14358898742961E-15,-0.377783449474029,
-1.86307814468624));
#29229=CARTESIAN_POINT('Ctrl Pts',(4.19109191795997E-15,-0.36231842649289,
-1.86431332307229));
#29230=CARTESIAN_POINT('Ctrl Pts',(4.40966368558951E-15,-0.291160344840241,
-1.86999665924045));
#29231=CARTESIAN_POINT('Ctrl Pts',(3.34716857295974E-15,-0.219690647889499,
-1.87166839472062));
#29232=CARTESIAN_POINT('Ctrl Pts',(5.21804821573824E-15,-0.148275107848417,
-1.86939686799115));
#29233=CARTESIAN_POINT('Ctrl Pts',(6.55714620959737E-15,-0.0971588285257386,
-1.86777100344225));
#29234=CARTESIAN_POINT('Ctrl Pts',(1.54180173149947E-15,-0.0460702963087095,
-1.86412382836371));
#29235=CARTESIAN_POINT('Ctrl Pts',(1.33226762955019E-15,0.00485094964988812,
-1.85846491542322));
#29236=CARTESIAN_POINT('Ctrl Pts',(1.21176555987097E-15,0.0341355170380698,
-1.8552105013917));
#29237=CARTESIAN_POINT('Ctrl Pts',(4.62515714886742E-15,0.0633646503133136,
-1.8512905051685));
#29238=CARTESIAN_POINT('Ctrl Pts',(5.74540415243519E-15,0.0925106744803074,
-1.84670495503791));
#29239=CARTESIAN_POINT('Ctrl Pts',(6.22649828274991E-15,0.105027540050217,
-1.84473567393735));
#29240=CARTESIAN_POINT('Ctrl Pts',(5.83817128828971E-15,0.117520189266528,
-1.84264500601019));
#29241=CARTESIAN_POINT('Ctrl Pts',(5.6621374255883E-15,0.129983639985351,
-1.84043395959634));
#29242=CARTESIAN_POINT('Ctrl Pts',(4.69391821206743E-15,0.198534953167655,
-1.82827279022231));
#29243=CARTESIAN_POINT('Ctrl Pts',(4.42924793610523E-15,0.266233864746607,
-1.81246923639649));
#29244=CARTESIAN_POINT('Ctrl Pts',(4.413136522885E-15,0.332741006672829,
-1.7930834653544));
#29245=CARTESIAN_POINT('Ctrl Pts',(4.39742118597367E-15,0.397613164570649,
-1.7741742660776));
#29246=CARTESIAN_POINT('Ctrl Pts',(2.78842801225445E-15,0.461352264091458,
-1.75185630563892));
#29247=CARTESIAN_POINT('Ctrl Pts',(2.52575738102223E-15,0.52361861632967,
-1.72614358359088));
#29248=CARTESIAN_POINT('Ctrl Pts',(2.35257199225765E-15,0.564672396757043,
-1.70919053580173));
#29249=CARTESIAN_POINT('Ctrl Pts',(9.35783025048596E-16,0.605085429674089,
-1.69076091627867));
#29250=CARTESIAN_POINT('Ctrl Pts',(7.21644966006352E-16,0.644751661649001,
-1.67084992281155));
#29251=CARTESIAN_POINT('Ctrl Pts',(5.4073076524326E-16,0.678263615045427,
-1.65402815144772));
#29252=CARTESIAN_POINT('Ctrl Pts',(6.64449045267152E-15,0.711242437386654,
-1.63614889178973));
#29253=CARTESIAN_POINT('Ctrl Pts',(6.68909372336657E-15,0.743619323760163,
-1.6172057038497));
#29254=CARTESIAN_POINT('Ctrl Pts',(6.70260297825943E-15,0.753425501734138,
-1.61146826911952));
#29255=CARTESIAN_POINT('Ctrl Pts',(-4.4167704875882E-15,0.763176219215081,
-1.60563322846188));
#29256=CARTESIAN_POINT('Ctrl Pts',(-4.10782519111308E-15,0.772857613917434,
-1.5997079485001));
#29257=CARTESIAN_POINT('Ctrl Pts',(-2.33423005065088E-15,0.828436626748831,
-1.56569206327379));
#29258=CARTESIAN_POINT('Ctrl Pts',(5.3236200784477E-15,0.88183656846137,
-1.52864593801835));
#29259=CARTESIAN_POINT('Ctrl Pts',(4.05231403988182E-15,0.932748709480243,
-1.48859056817433));
#29260=CARTESIAN_POINT('Ctrl Pts',(3.67993039744611E-15,0.947661600587246,
-1.47685777994778));
#29261=CARTESIAN_POINT('Ctrl Pts',(-2.77500390110177E-15,0.962360807573884,
-1.46486655879511));
#29262=CARTESIAN_POINT('Ctrl Pts',(-2.52575738102223E-15,0.976837943247501,
-1.45261684628832));
#29263=CARTESIAN_POINT('Ctrl Pts',(-1.61095971371858E-15,1.02921122594054,
-1.40830161221923));
#29264=CARTESIAN_POINT('Ctrl Pts',(-1.20919530929667E-15,1.07868231006794,
-1.36060541153686));
#29265=CARTESIAN_POINT('Ctrl Pts',(-1.08246744900953E-15,1.12509528635148,
-1.30988296450997));
#29266=CARTESIAN_POINT('Ctrl Pts',(-9.67595445409575E-16,1.16716615827062,
-1.26390578866033));
#29267=CARTESIAN_POINT('Ctrl Pts',(4.18879340799465E-17,1.20672391844854,
-1.21544096567182));
#29268=CARTESIAN_POINT('Ctrl Pts',(1.01307850997046E-15,1.24361190857,-1.16474132238846));
#29269=CARTESIAN_POINT('Ctrl Pts',(1.19552438322947E-15,1.25054161087308,
-1.15521699119912));
#29270=CARTESIAN_POINT('Ctrl Pts',(2.90706964741059E-15,1.25737148574206,
-1.14562128847553));
#29271=CARTESIAN_POINT('Ctrl Pts',(2.84494650060196E-15,1.26409862962719,
-1.13595948716456));
#29272=CARTESIAN_POINT('Ctrl Pts',(2.50292880016366E-15,1.30113478121168,
-1.08276663979238));
#29273=CARTESIAN_POINT('Ctrl Pts',(1.91762847285502E-15,1.33508460122726,
-1.02753972970139));
#29274=CARTESIAN_POINT('Ctrl Pts',(2.04003480774873E-15,1.36583796777706,
-0.970591450617083));
#29275=CARTESIAN_POINT('Ctrl Pts',(2.16190419186033E-15,1.39645643081688,
-0.913892982320922));
#29276=CARTESIAN_POINT('Ctrl Pts',(-1.01931864381867E-15,1.42390663940794,
-0.855487109860612));
#29277=CARTESIAN_POINT('Ctrl Pts',(-3.59434704222394E-15,1.44803019585752,
-0.795670327485843));
#29278=CARTESIAN_POINT('Ctrl Pts',(-6.11597449534489E-15,1.47165347793389,
-0.737094025691661));
#29279=CARTESIAN_POINT('Ctrl Pts',(1.01337469259877E-15,1.4920867044338,
-0.677163760277832));
#29280=CARTESIAN_POINT('Ctrl Pts',(2.08166817117217E-16,1.5091315905072,
-0.616161567602637));
#29281=CARTESIAN_POINT('Ctrl Pts',(6.26169911362964E-17,1.51221263364822,
-0.605134777131891));
#29282=CARTESIAN_POINT('Ctrl Pts',(3.45179592633212E-16,1.5151828306955,
-0.594072993522759));
#29283=CARTESIAN_POINT('Ctrl Pts',(3.88578058618805E-16,1.51804083102399,
-0.582977932470115));
#29284=CARTESIAN_POINT('Ctrl Pts',(4.28030529389721E-16,1.52063896835125,
-0.572891687209135));
#29285=CARTESIAN_POINT('Ctrl Pts',(-1.01862452835985E-15,1.52314194434016,
-0.562787410979804));
#29286=CARTESIAN_POINT('Ctrl Pts',(-8.32667268468867E-16,1.52554925331476,
-0.552666456127963));
#29287=CARTESIAN_POINT('Ctrl Pts',(2.76065174993704E-16,1.53990234478933,
-0.492322315707556));
#29288=CARTESIAN_POINT('Ctrl Pts',(-3.91459791985415E-16,1.55085890343775,
-0.431384487161399));
#29289=CARTESIAN_POINT('Ctrl Pts',(3.01841884819964E-16,1.55828603425274,
-0.370123355547507));
#29290=CARTESIAN_POINT('Ctrl Pts',(9.825982558262E-16,1.56557877100754,
-0.309970745166737));
#29291=CARTESIAN_POINT('Ctrl Pts',(3.5825896615399E-15,1.56946866269597,
-0.24950554168674));
#29292=CARTESIAN_POINT('Ctrl Pts',(3.23005511226881E-15,1.56978073257091,
-0.188991307723295));
#29293=CARTESIAN_POINT('Ctrl Pts',(2.88873803673286E-15,1.57008287253789,
-0.130402606538099));
#29294=CARTESIAN_POINT('Ctrl Pts',(5.02537364202987E-15,1.56703113522227,
-0.0717672828486066));
#29295=CARTESIAN_POINT('Ctrl Pts',(6.32133234645949E-15,1.56042122340447,
-0.013342828381275));
#29296=CARTESIAN_POINT('Ctrl Pts',(6.62092093472987E-15,1.55889320083453,
0.000163234562326977));
#29297=CARTESIAN_POINT('Ctrl Pts',(2.18341315110387E-15,1.55717483559577,
0.0136579261245166));
#29298=CARTESIAN_POINT('Ctrl Pts',(2.22044604925031E-15,1.55526325306019,
0.0271378643347));
#29299=CARTESIAN_POINT('Ctrl Pts',(-0.121869692124238,-1.95503470185946,
-0.00140694303418273));
#29300=CARTESIAN_POINT('Ctrl Pts',(-0.115576597737629,-1.9560114957989,
-0.111573334849889));
#29301=CARTESIAN_POINT('Ctrl Pts',(-0.10928350335102,-1.9475116218801,-0.221598758420366));
#29302=CARTESIAN_POINT('Ctrl Pts',(-0.10299040896441,-1.92900481620408,
-0.329922931291736));
#29303=CARTESIAN_POINT('Ctrl Pts',(-0.0686602726429393,-1.82804634923992,
-0.920853782336577));
#29304=CARTESIAN_POINT('Ctrl Pts',(-0.0343301363214685,-1.42928869857895,
-1.46115662054476));
#29305=CARTESIAN_POINT('Ctrl Pts',(2.32452945780892E-15,-0.897777576978214,
-1.73914455526119));
#29306=CARTESIAN_POINT('',(-15.646,-0.903606778650182,-1.26612599672285));
#29307=CARTESIAN_POINT('Ctrl Pts',(-15.646,-0.90554130419335,-1.26787397308659));
#29308=CARTESIAN_POINT('Ctrl Pts',(-15.646,-0.9388319205117,-1.25008095488368));
#29309=CARTESIAN_POINT('Ctrl Pts',(-15.646,-0.971367568991014,-1.23102934423823));
#29310=CARTESIAN_POINT('Ctrl Pts',(-15.646,-1.0030683062222,-1.21073538899741));
#29311=CARTESIAN_POINT('Ctrl Pts',(-15.646,-1.05303568714615,-1.17874762213329));
#29312=CARTESIAN_POINT('Ctrl Pts',(-15.646,-1.10093004937321,-1.14367606433464));
#29313=CARTESIAN_POINT('Ctrl Pts',(-15.646,-1.14667319981616,-1.10584089641864));
#29314=CARTESIAN_POINT('Ctrl Pts',(-15.646,-1.17363908823249,-1.08353681577801));
#29315=CARTESIAN_POINT('Ctrl Pts',(-15.646,-1.1998571211457,-1.06027134077856));
#29316=CARTESIAN_POINT('Ctrl Pts',(-15.646,-1.22530816463228,-1.03610248194796));
#29317=CARTESIAN_POINT('Ctrl Pts',(-15.646,-1.23682022027328,-1.02517038606812));
#29318=CARTESIAN_POINT('Ctrl Pts',(-15.646,-1.24817682883917,-1.01405163699654));
#29319=CARTESIAN_POINT('Ctrl Pts',(-15.646,-1.25936010833055,-1.00276802411491));
#29320=CARTESIAN_POINT('Ctrl Pts',(-15.646,-1.30322784282822,-0.958506720045097));
#29321=CARTESIAN_POINT('Ctrl Pts',(-15.646,-1.34448541532842,-0.911661957910068));
#29322=CARTESIAN_POINT('Ctrl Pts',(-15.646,-1.38304512047716,-0.862582893866261));
#29323=CARTESIAN_POINT('Ctrl Pts',(-15.646,-1.41274047352769,-0.824786439548259));
#29324=CARTESIAN_POINT('Ctrl Pts',(-15.646,-1.44083552294601,-0.785663647481262));
#29325=CARTESIAN_POINT('Ctrl Pts',(-15.646,-1.4672800556148,-0.745355620103979));
#29326=CARTESIAN_POINT('Ctrl Pts',(-15.646,-1.47638184737574,-0.731482231752685));
#29327=CARTESIAN_POINT('Ctrl Pts',(-15.646,-1.48528802466688,-0.717468314833474));
#29328=CARTESIAN_POINT('Ctrl Pts',(-15.646,-1.4939962396742,-0.70331926166881));
#29329=CARTESIAN_POINT('Ctrl Pts',(-15.646,-1.50231026779888,-0.689810680880463));
#29330=CARTESIAN_POINT('Ctrl Pts',(-15.646,-1.51044565988147,-0.676175502864343));
#29331=CARTESIAN_POINT('Ctrl Pts',(-15.646,-1.5183869558134,-0.662442089798388));
#29332=CARTESIAN_POINT('Ctrl Pts',(-15.646,-1.55077996339743,-0.606422699838139));
#29333=CARTESIAN_POINT('Ctrl Pts',(-15.646,-1.57999117124514,-0.548701659160568));
#29334=CARTESIAN_POINT('Ctrl Pts',(-15.646,-1.60592950648782,-0.489633408577941));
#29335=CARTESIAN_POINT('Ctrl Pts',(-15.646,-1.6324092676445,-0.429332192145295));
#29336=CARTESIAN_POINT('Ctrl Pts',(-15.646,-1.65547885224142,-0.367626155535072));
#29337=CARTESIAN_POINT('Ctrl Pts',(-15.646,-1.67500744714839,-0.304850769250659));
#29338=CARTESIAN_POINT('Ctrl Pts',(-15.646,-1.68791747427872,-0.263351012411529));
#29339=CARTESIAN_POINT('Ctrl Pts',(-15.646,-1.69927926283844,-0.221383073699382));
#29340=CARTESIAN_POINT('Ctrl Pts',(-15.646,-1.70904465268481,-0.179036877539802));
#29341=CARTESIAN_POINT('Ctrl Pts',(-15.646,-1.71384145896988,-0.158236223077195));
#29342=CARTESIAN_POINT('Ctrl Pts',(-15.646,-1.71825294582739,-0.137344232813234));
#29343=CARTESIAN_POINT('Ctrl Pts',(-15.646,-1.72227256103369,-0.116371238196171));
#29344=CARTESIAN_POINT('Ctrl Pts',(-15.646,-1.72482838629632,-0.103035805144933));
#29345=CARTESIAN_POINT('Ctrl Pts',(-15.646,-1.72722577012393,-0.0896676190078338));
#29346=CARTESIAN_POINT('Ctrl Pts',(-15.646,-1.72946290153931,-0.0762693043065953));
#29347=CARTESIAN_POINT('Ctrl Pts',(-15.646,-1.73118679540451,-0.065944800185506));
#29348=CARTESIAN_POINT('Ctrl Pts',(-15.646,-1.73281491882756,-0.0556057409752924));
#29349=CARTESIAN_POINT('Ctrl Pts',(-15.646,-1.73434548980575,-0.045261864309701));
#29350=CARTESIAN_POINT('Ctrl Pts',(-15.646,-1.74426354163551,0.0217661313542963));
#29351=CARTESIAN_POINT('Ctrl Pts',(-15.646,-1.75010629770909,0.0890975130769489));
#29352=CARTESIAN_POINT('Ctrl Pts',(-15.646,-1.75175066215845,0.156377409541393));
#29353=CARTESIAN_POINT('Ctrl Pts',(-15.646,-1.75216844738295,0.173471276208168));
#29354=CARTESIAN_POINT('Ctrl Pts',(-15.646,-1.75231500242569,0.190561969387215));
#29355=CARTESIAN_POINT('Ctrl Pts',(-15.646,-1.75218784680546,0.207643941770755));
#29356=CARTESIAN_POINT('Ctrl Pts',(-15.646,-1.7517050717956,0.272499505144288));
#29357=CARTESIAN_POINT('Ctrl Pts',(-15.646,-1.74728083397727,0.337228600758688));
#29358=CARTESIAN_POINT('Ctrl Pts',(-15.646,-1.73913184783819,0.401595905267991));
#29359=CARTESIAN_POINT('Ctrl Pts',(-15.646,-1.73471144430273,0.436511839049797));
#29360=CARTESIAN_POINT('Ctrl Pts',(-15.646,-1.72919412473302,0.47132150623283));
#29361=CARTESIAN_POINT('Ctrl Pts',(-15.646,-1.72260827310355,0.505987965615567));
#29362=CARTESIAN_POINT('Ctrl Pts',(-15.646,-1.71757351777636,0.532489798768173));
#29363=CARTESIAN_POINT('Ctrl Pts',(-15.646,-1.71191419079661,0.558907947509954));
#29364=CARTESIAN_POINT('Ctrl Pts',(-15.646,-1.70564134060446,0.585225824611134));
#29365=CARTESIAN_POINT('Ctrl Pts',(-15.646,-1.70220225814383,0.599654568605839));
#29366=CARTESIAN_POINT('Ctrl Pts',(-15.646,-1.69857761981803,0.614056894407544));
#29367=CARTESIAN_POINT('Ctrl Pts',(-15.646,-1.69477643427966,0.628403772607706));
#29368=CARTESIAN_POINT('Ctrl Pts',(-15.646,-1.67740647456813,0.693963502278271));
#29369=CARTESIAN_POINT('Ctrl Pts',(-15.646,-1.65633175680869,0.758467910098477));
#29370=CARTESIAN_POINT('Ctrl Pts',(-15.646,-1.63180977190725,0.821661415923179));
#29371=CARTESIAN_POINT('Ctrl Pts',(-15.646,-1.60677175649931,0.886184739743799));
#29372=CARTESIAN_POINT('Ctrl Pts',(-15.646,-1.57813969140247,0.949342287961683));
#29373=CARTESIAN_POINT('Ctrl Pts',(-15.646,-1.546132490592,1.01086511111923));
#29374=CARTESIAN_POINT('Ctrl Pts',(-15.646,-1.51388293863644,1.07285377090927));
#29375=CARTESIAN_POINT('Ctrl Pts',(-15.646,-1.47820662246953,1.1331838390446));
#29376=CARTESIAN_POINT('Ctrl Pts',(-15.646,-1.43927596686557,1.19156917309334));
#29377=CARTESIAN_POINT('Ctrl Pts',(-15.646,-1.4294481205191,1.20630825423689));
#29378=CARTESIAN_POINT('Ctrl Pts',(-15.646,-1.41941263972777,1.22092330393712));
#29379=CARTESIAN_POINT('Ctrl Pts',(-15.646,-1.40917182388351,1.23540949097454));
#29380=CARTESIAN_POINT('Ctrl Pts',(-15.646,-1.40170116694523,1.24597713864501));
#29381=CARTESIAN_POINT('Ctrl Pts',(-15.646,-1.39412021842425,1.25647742423705));
#29382=CARTESIAN_POINT('Ctrl Pts',(-15.646,-1.3864413518955,1.26689325751344));
#29383=CARTESIAN_POINT('Ctrl Pts',(-15.646,-1.34360456056451,1.3249983013931));
#29384=CARTESIAN_POINT('Ctrl Pts',(-15.646,-1.29765039571163,1.38058334275533));
#29385=CARTESIAN_POINT('Ctrl Pts',(-15.646,-1.24882029809218,1.43336797698167));
#29386=CARTESIAN_POINT('Ctrl Pts',(-15.646,-1.19987423803885,1.48627796493359));
#29387=CARTESIAN_POINT('Ctrl Pts',(-15.646,-1.14803813754689,1.53637523807351));
#29388=CARTESIAN_POINT('Ctrl Pts',(-15.646,-1.09350553802909,1.58336120199917));
#29389=CARTESIAN_POINT('Ctrl Pts',(-15.646,-1.04013426283505,1.62934655448756));
#29390=CARTESIAN_POINT('Ctrl Pts',(-15.646,-0.984179545234824,1.6723525600043));
#29391=CARTESIAN_POINT('Ctrl Pts',(-15.646,-0.925783035097312,1.71207017058232));
#29392=CARTESIAN_POINT('Ctrl Pts',(-15.646,-0.904681296506683,1.72642223775017));
#29393=CARTESIAN_POINT('Ctrl Pts',(-15.646,-0.883260377259073,1.74034457784343));
#29394=CARTESIAN_POINT('Ctrl Pts',(-15.646,-0.861525859670562,1.75382131162753));
#29395=CARTESIAN_POINT('Ctrl Pts',(-15.646,-0.905541304193346,-1.2678739730866));
#29396=CARTESIAN_POINT('Ctrl Pts',(-15.6116698636785,-0.515499657429897,
-1.54330953138525));
#29397=CARTESIAN_POINT('Ctrl Pts',(-15.5403325616641,0.580821856359331,
-1.72219244777323));
#29398=CARTESIAN_POINT('Ctrl Pts',(-15.4319880939568,1.77133009557791,-0.489978596140976));
#29399=CARTESIAN_POINT('Ctrl Pts',(-15.3209665968779,1.37345033995276,1.2214745163176));
#29400=CARTESIAN_POINT('Ctrl Pts',(-15.2099450997991,-0.279367108572254,
1.81642835228867));
#29401=CARTESIAN_POINT('Ctrl Pts',(-15.1202708256386,-1.40814580884089,
0.95690627970636));
#29402=CARTESIAN_POINT('Ctrl Pts',(-15.067603717171,-1.55400039997039,0.220042953926479));
#29403=CARTESIAN_POINT('Ctrl Pts',(-15.0519437743963,-1.55320111767851,
0.000640865722738825));
#29404=CARTESIAN_POINT('Origin',(-15.646,-2.59090492670967E-16,0.));
#29405=CARTESIAN_POINT('',(-15.646,-1.954,-2.39295984553393E-16));
#29406=CARTESIAN_POINT('Origin',(-15.646,0.,0.));
#29407=CARTESIAN_POINT('Origin',(-15.646,0.,0.));
#29408=CARTESIAN_POINT('',(-15.646,0.903606778650233,-1.26612599672282));
#29409=CARTESIAN_POINT('Ctrl Pts',(-15.646,0.863566983235665,1.75638267756862));
#29410=CARTESIAN_POINT('Ctrl Pts',(-15.646,0.903502374498014,1.73186322492154));
#29411=CARTESIAN_POINT('Ctrl Pts',(-15.646,0.942431754046728,1.7058442816782));
#29412=CARTESIAN_POINT('Ctrl Pts',(-15.646,0.980258194321091,1.67832096079393));
#29413=CARTESIAN_POINT('Ctrl Pts',(-15.646,1.03835777356149,1.6360464736607));
#29414=CARTESIAN_POINT('Ctrl Pts',(-15.646,1.09385752849377,1.59022401101361));
#29415=CARTESIAN_POINT('Ctrl Pts',(-15.646,1.14659587359059,1.54119436771133));
#29416=CARTESIAN_POINT('Ctrl Pts',(-15.646,1.17214536647838,1.5174415836499));
#29417=CARTESIAN_POINT('Ctrl Pts',(-15.646,1.19704611900917,1.49293561765741));
#29418=CARTESIAN_POINT('Ctrl Pts',(-15.646,1.22127593441469,1.46771321296535));
#29419=CARTESIAN_POINT('Ctrl Pts',(-15.646,1.23155978876183,1.45700807420153));
#29420=CARTESIAN_POINT('Ctrl Pts',(-15.646,1.24172274779762,1.44617386383036));
#29421=CARTESIAN_POINT('Ctrl Pts',(-15.646,1.25176296848256,1.43521334664126));
#29422=CARTESIAN_POINT('Ctrl Pts',(-15.646,1.26224201312144,1.42377378246295));
#29423=CARTESIAN_POINT('Ctrl Pts',(-15.646,1.27258196295285,1.41220243610557));
#29424=CARTESIAN_POINT('Ctrl Pts',(-15.646,1.28277672403329,1.40050803765028));
#29425=CARTESIAN_POINT('Ctrl Pts',(-15.646,1.32968516061639,1.34669942516889));
#29426=CARTESIAN_POINT('Ctrl Pts',(-15.646,1.37355485596852,1.2902533722939));
#29427=CARTESIAN_POINT('Ctrl Pts',(-15.646,1.41422309221843,1.23150451481102));
#29428=CARTESIAN_POINT('Ctrl Pts',(-15.646,1.44333172695657,1.18945452220145));
#29429=CARTESIAN_POINT('Ctrl Pts',(-15.646,1.4707993065757,1.14622410435876));
#29430=CARTESIAN_POINT('Ctrl Pts',(-15.646,1.49655049600041,1.10193110550949));
#29431=CARTESIAN_POINT('Ctrl Pts',(-15.646,1.51135988777298,1.07645840357241));
#29432=CARTESIAN_POINT('Ctrl Pts',(-15.646,1.52560136048139,1.05063421753584));
#29433=CARTESIAN_POINT('Ctrl Pts',(-15.646,1.53925846964067,1.02448080677582));
#29434=CARTESIAN_POINT('Ctrl Pts',(-15.646,1.54512355904191,1.01324914050839));
#29435=CARTESIAN_POINT('Ctrl Pts',(-15.646,1.55087667965087,1.00196470925521));
#29436=CARTESIAN_POINT('Ctrl Pts',(-15.646,1.5565156774274,0.990632117118322));
#29437=CARTESIAN_POINT('Ctrl Pts',(-15.646,1.58753124253106,0.928300695269239));
#29438=CARTESIAN_POINT('Ctrl Pts',(-15.646,1.61511219349458,0.864487052005008));
#29439=CARTESIAN_POINT('Ctrl Pts',(-15.646,1.63910495617291,0.799499739891529));
#29440=CARTESIAN_POINT('Ctrl Pts',(-15.646,1.66250789621328,0.736110034038682));
#29441=CARTESIAN_POINT('Ctrl Pts',(-15.646,1.68249698900462,0.671602682530926));
#29442=CARTESIAN_POINT('Ctrl Pts',(-15.646,1.69888136394285,0.606259025222021));
#29443=CARTESIAN_POINT('Ctrl Pts',(-15.646,1.70968399200845,0.56317631812975));
#29444=CARTESIAN_POINT('Ctrl Pts',(-15.646,1.71891862839643,0.519729989653583));
#29445=CARTESIAN_POINT('Ctrl Pts',(-15.646,1.72651830953887,0.476002417985191));
#29446=CARTESIAN_POINT('Ctrl Pts',(-15.646,1.73293889141712,0.439059229320861));
#29447=CARTESIAN_POINT('Ctrl Pts',(-15.646,1.73819233547822,0.401915291206649));
#29448=CARTESIAN_POINT('Ctrl Pts',(-15.646,1.74223252542586,0.364622070603487));
#29449=CARTESIAN_POINT('Ctrl Pts',(-15.646,1.74345619948668,0.353326872286555));
#29450=CARTESIAN_POINT('Ctrl Pts',(-15.646,1.74456842691372,0.342018170207851));
#29451=CARTESIAN_POINT('Ctrl Pts',(-15.646,1.74556687996462,0.330711488807271));
#29452=CARTESIAN_POINT('Ctrl Pts',(-15.646,1.75129881468264,0.265801917338621));
#29453=CARTESIAN_POINT('Ctrl Pts',(-15.646,1.75329872256676,0.200840616042056));
#29454=CARTESIAN_POINT('Ctrl Pts',(-15.646,1.7513997771477,0.136088205278388));
#29455=CARTESIAN_POINT('Ctrl Pts',(-15.646,1.75084355022554,0.117121344103708));
#29456=CARTESIAN_POINT('Ctrl Pts',(-15.646,1.74995247314858,0.0981724485182577));
#29457=CARTESIAN_POINT('Ctrl Pts',(-15.646,1.74872150843178,0.0792482245434431));
#29458=CARTESIAN_POINT('Ctrl Pts',(-15.646,1.7442682940956,0.0107867777160483));
#29459=CARTESIAN_POINT('Ctrl Pts',(-15.646,1.73537089691159,-0.0573539081323246));
#29460=CARTESIAN_POINT('Ctrl Pts',(-15.646,1.72222163795807,-0.124837458918125));
#29461=CARTESIAN_POINT('Ctrl Pts',(-15.646,1.7103025383206,-0.186007686727107));
#29462=CARTESIAN_POINT('Ctrl Pts',(-15.646,1.69488873716282,-0.24663831729391));
#29463=CARTESIAN_POINT('Ctrl Pts',(-15.646,1.67609021756689,-0.306453003759262));
#29464=CARTESIAN_POINT('Ctrl Pts',(-15.646,1.67255876966726,-0.317689657146101));
#29465=CARTESIAN_POINT('Ctrl Pts',(-15.646,1.66891056048996,-0.328888546226132));
#29466=CARTESIAN_POINT('Ctrl Pts',(-15.646,1.6651481002395,-0.340044199921187));
#29467=CARTESIAN_POINT('Ctrl Pts',(-15.646,1.64443393500422,-0.401461474407603));
#29468=CARTESIAN_POINT('Ctrl Pts',(-15.646,1.62024853883519,-0.461608555356997));
#29469=CARTESIAN_POINT('Ctrl Pts',(-15.646,1.5927777004272,-0.520210875318301));
#29470=CARTESIAN_POINT('Ctrl Pts',(-15.646,1.56542737352935,-0.578556113425322));
#29471=CARTESIAN_POINT('Ctrl Pts',(-15.646,1.53481960882925,-0.635370945735342));
#29472=CARTESIAN_POINT('Ctrl Pts',(-15.646,1.50109845003964,-0.690351644448425));
#29473=CARTESIAN_POINT('Ctrl Pts',(-15.646,1.46807660782277,-0.744192141722088));
#29474=CARTESIAN_POINT('Ctrl Pts',(-15.646,1.43206841909097,-0.796274405573291));
#29475=CARTESIAN_POINT('Ctrl Pts',(-15.646,1.3931825738236,-0.846271253612836));
#29476=CARTESIAN_POINT('Ctrl Pts',(-15.646,1.38615361009627,-0.855308630296688));
#29477=CARTESIAN_POINT('Ctrl Pts',(-15.646,1.37903056784112,-0.864277742013307));
#29478=CARTESIAN_POINT('Ctrl Pts',(-15.646,1.37181402230227,-0.873176482427014));
#29479=CARTESIAN_POINT('Ctrl Pts',(-15.646,1.36525350796304,-0.881266269122166));
#29480=CARTESIAN_POINT('Ctrl Pts',(-15.646,1.35862187689793,-0.889290301674277));
#29481=CARTESIAN_POINT('Ctrl Pts',(-15.646,1.35191991563543,-0.897247368324002));
#29482=CARTESIAN_POINT('Ctrl Pts',(-15.646,1.31196126683496,-0.944689246795767));
#29483=CARTESIAN_POINT('Ctrl Pts',(-15.646,1.26950445045268,-0.989754560841547));
#29484=CARTESIAN_POINT('Ctrl Pts',(-15.646,1.22468770075641,-1.03217561515895));
#29485=CARTESIAN_POINT('Ctrl Pts',(-15.646,1.18068191727077,-1.07382905375448));
#29486=CARTESIAN_POINT('Ctrl Pts',(-15.646,1.13440012852228,-1.11293359637472));
#29487=CARTESIAN_POINT('Ctrl Pts',(-15.646,1.08595004589958,-1.14919178596454));
#29488=CARTESIAN_POINT('Ctrl Pts',(-15.646,1.03904162600828,-1.18429625410389));
#29489=CARTESIAN_POINT('Ctrl Pts',(-15.646,0.990100100246089,-1.21673292322258));
#29490=CARTESIAN_POINT('Ctrl Pts',(-15.646,0.939210854429017,-1.24618438366542));
#29491=CARTESIAN_POINT('Ctrl Pts',(-15.646,0.927446614173192,-1.25299277807118));
#29492=CARTESIAN_POINT('Ctrl Pts',(-15.646,0.915578253025946,-1.25964142336886));
#29493=CARTESIAN_POINT('Ctrl Pts',(-15.646,0.903606778650246,-1.26612599672281));
#29494=CARTESIAN_POINT('Origin',(-15.646,0.,0.));
#29495=CARTESIAN_POINT('Origin',(-16.9400562256037,0.,0.));
#29496=CARTESIAN_POINT('Ctrl Pts',(-15.646,0.903606778650232,-1.26612599672282));
#29497=CARTESIAN_POINT('Ctrl Pts',(-15.6089928343071,1.32418286847098,-0.965969924828001));
#29498=CARTESIAN_POINT('Ctrl Pts',(-15.5349785029212,1.83555016250808,0.0811162878112121));
#29499=CARTESIAN_POINT('Ctrl Pts',(-15.4239570058423,0.927248239037281,
1.58822321403664));
#29500=CARTESIAN_POINT('Ctrl Pts',(-15.3129355087635,-0.828910895913401,
1.63972535647931));
#29501=CARTESIAN_POINT('Ctrl Pts',(-15.2349685820173,-1.53012672072011,
0.625555336487783));
#29502=CARTESIAN_POINT('Ctrl Pts',(-15.194008820964,-1.55770177041248,0.0560323151841793));
#29503=CARTESIAN_POINT('Ctrl Pts',(-15.1900562256037,-1.55731346481242,
0.00103325697183652));
#29504=CARTESIAN_POINT('Ctrl Pts',(-15.8760740822721,1.13509973994377,-1.59049193030949));
#29505=CARTESIAN_POINT('Ctrl Pts',(-15.8390669165791,1.66342225971859,-1.21343955841462));
#29506=CARTESIAN_POINT('Ctrl Pts',(-15.7650525851932,2.30579557540391,0.101897284720716));
#29507=CARTESIAN_POINT('Ctrl Pts',(-15.6540310881144,1.16479785218828,1.99510649966415));
#29508=CARTESIAN_POINT('Ctrl Pts',(-15.5430095910356,-1.04126768924124,
2.05980285860533));
#29509=CARTESIAN_POINT('Ctrl Pts',(-15.4319880939568,-2.29557200334843,
0.245699716161034));
#29510=CARTESIAN_POINT('Ctrl Pts',(-15.3209665968779,-1.45300688747799,
-1.79439621415821));
#29511=CARTESIAN_POINT('Ctrl Pts',(-15.2099450997991,0.717101347881572,
-2.19440670210365));
#29512=CARTESIAN_POINT('Ctrl Pts',(-15.0989236027203,2.23202382251325,-0.590124666540823));
#29513=CARTESIAN_POINT('Ctrl Pts',(-14.9879021056415,1.70790504136699,1.55349118140293));
#29514=CARTESIAN_POINT('Ctrl Pts',(-14.8768806085626,-0.376501591705209,
2.27778871648529));
#29515=CARTESIAN_POINT('Ctrl Pts',(-14.7658591114838,-2.11694215263163,
0.921258901245484));
#29516=CARTESIAN_POINT('Ctrl Pts',(-14.654837614405,-1.92344217019805,-1.27692506070559));
#29517=CARTESIAN_POINT('Ctrl Pts',(-14.5438161173262,0.0272337144496871,
-2.30854902471789));
#29518=CARTESIAN_POINT('Ctrl Pts',(-14.4327946202473,1.95302852331423,-1.2311920503561));
#29519=CARTESIAN_POINT('Ctrl Pts',(-14.3217731231685,2.09462236852777,0.970933007055954));
#29520=CARTESIAN_POINT('Ctrl Pts',(-14.2107516260897,0.322660046842802,
2.28605351825641));
#29521=CARTESIAN_POINT('Ctrl Pts',(-14.0997301290109,-1.74407021311087,
1.5127364171163));
#29522=CARTESIAN_POINT('Ctrl Pts',(-13.988708631932,-2.21749402601248,-0.642551447391479));
#29523=CARTESIAN_POINT('Ctrl Pts',(-13.8776871348532,-0.665111842436208,
-2.21083194745943));
#29524=CARTESIAN_POINT('Ctrl Pts',(-13.7666656377744,1.49488751168712,-1.75939288428676));
#29525=CARTESIAN_POINT('Ctrl Pts',(-13.6556441406956,2.28922277847452,0.299350966372687));
#29526=CARTESIAN_POINT('Ctrl Pts',(-13.5446226436167,0.992223838228365,
2.0846207641111));
#29527=CARTESIAN_POINT('Ctrl Pts',(-13.4336011465379,-1.21122756867257,
1.96547187749358));
#29528=CARTESIAN_POINT('Ctrl Pts',(-13.3225796494591,-2.30815423967428,
0.0507534971524391));
#29529=CARTESIAN_POINT('Ctrl Pts',(-13.2115581523803,-1.29645175311226,
-1.91033105957732));
#29530=CARTESIAN_POINT('Ctrl Pts',(-13.1005366553014,0.89963257316349,-2.12622038973593));
#29531=CARTESIAN_POINT('Ctrl Pts',(-12.9895151582226,2.27385177436925,-0.399687400733145));
#29532=CARTESIAN_POINT('Ctrl Pts',(-12.8784936611438,1.57077905700222,1.69198258370345));
#29533=CARTESIAN_POINT('Ctrl Pts',(-12.767472164065,-0.56728897414607,2.23793099319152));
#29534=CARTESIAN_POINT('Ctrl Pts',(-12.6564506669861,-2.18710651309118,
0.739403144753916));
#29535=CARTESIAN_POINT('Ctrl Pts',(-12.5454291699073,-1.80887882518214,
-1.43461120371879));
#29536=CARTESIAN_POINT('Ctrl Pts',(-12.4344076728285,0.221861751741927,
-2.29802725686185));
#29537=CARTESIAN_POINT('Ctrl Pts',(-12.3233861757497,2.04991909791636,-1.06206572400144));
#29538=CARTESIAN_POINT('Ctrl Pts',(-12.2123646786708,2.00525966305359,1.14415278430378));
#29539=CARTESIAN_POINT('Ctrl Pts',(-12.101343181592,0.128682361216318,2.30512315506791));
#29540=CARTESIAN_POINT('Ctrl Pts',(-11.9903216845132,-1.86545353965054,
1.36023343640473));
#29541=CARTESIAN_POINT('Ctrl Pts',(-11.8793001874344,-2.15539235708442,
-0.827306289792927));
#29542=CARTESIAN_POINT('Ctrl Pts',(-11.7682786903555,-0.476258618959912,
-2.2590550320826));
#29543=CARTESIAN_POINT('Ctrl Pts',(-11.6572571932767,1.63796424475246,-1.62702951510483));
#29544=CARTESIAN_POINT('Ctrl Pts',(-11.5462356961979,2.25581433404732,0.491379283666496));
#29545=CARTESIAN_POINT('Ctrl Pts',(-11.435214199119,0.812850724616405,2.16088537632167));
#29546=CARTESIAN_POINT('Ctrl Pts',(-11.3241927020402,-1.37269789415048,
1.85630073035186));
#29547=CARTESIAN_POINT('Ctrl Pts',(-11.2131712049614,-2.30420951980991,
-0.144119391226494));
#29548=CARTESIAN_POINT('Ctrl Pts',(-11.1021497078826,-1.13069571341659,
-2.01287831568912));
#29549=CARTESIAN_POINT('Ctrl Pts',(-10.9911282108037,1.07577243683834,-2.04275930404171));
#29550=CARTESIAN_POINT('Ctrl Pts',(-10.8801067137249,2.2994617559248,-0.206464387121221));
#29551=CARTESIAN_POINT('Ctrl Pts',(-10.7690852166461,1.42246299320277,1.81844739904093));
#29552=CARTESIAN_POINT('Ctrl Pts',(-10.6580637195673,-0.75403598905343,
2.18210486396101));
#29553=CARTESIAN_POINT('Ctrl Pts',(-10.5470422224884,-2.24168054205987,
0.552286390797627));
#29554=CARTESIAN_POINT('Ctrl Pts',(-10.4360207254096,-1.68142341294711,
-1.58207686807671));
#29555=CARTESIAN_POINT('Ctrl Pts',(-10.3249992283308,0.414908893302569,
-2.27112362507384));
#29556=CARTESIAN_POINT('Ctrl Pts',(-10.213977731252,2.13219851056152,-0.885370782028248));
#29557=CARTESIAN_POINT('Ctrl Pts',(-10.1029562341731,1.90160445998143,1.30921823539425));
#29558=CARTESIAN_POINT('Ctrl Pts',(-9.99193473709432,-0.0662125798935141,
2.30776251039268));
#29559=CARTESIAN_POINT('Ctrl Pts',(-9.88091324001547,-1.97354069139653,
1.19803549593164));
#29560=CARTESIAN_POINT('Ctrl Pts',(-9.76989174293666,-2.07792800655941,
-1.00616455397024));
#29561=CARTESIAN_POINT('Ctrl Pts',(-9.65887024585783,-0.284010821989528,
-2.29117650195329));
#29562=CARTESIAN_POINT('Ctrl Pts',(-9.54784874877901,1.7693662763279,-1.48306941520065));
#29563=CARTESIAN_POINT('Ctrl Pts',(-9.43682725170018,2.20632742884456,0.679905277842615));
#29564=CARTESIAN_POINT('Ctrl Pts',(-9.32580575462136,0.62768396328097,2.22174812981805));
#29565=CARTESIAN_POINT('Ctrl Pts',(-9.21478425754252,-1.52438422544196,
1.73389868312246));
#29566=CARTESIAN_POINT('Ctrl Pts',(-9.10376276046371,-2.28384139715977,
-0.337965061403401));
#29567=CARTESIAN_POINT('Ctrl Pts',(-8.99274126338487,-0.956880566319905,
-2.10107864962485));
#29568=CARTESIAN_POINT('Ctrl Pts',(-8.88171976630606,1.24424466242879,-1.94473831919042));
#29569=CARTESIAN_POINT('Ctrl Pts',(-8.77069826922723,2.30868217437448,-0.0117697848585148));
#29570=CARTESIAN_POINT('Ctrl Pts',(-8.6596767721484,1.26400823191302,1.9319511121574));
#29571=CARTESIAN_POINT('Ctrl Pts',(-8.54865527506958,-0.935408563412113,
2.11072564053346));
#29572=CARTESIAN_POINT('Ctrl Pts',(-8.43763377799075,-2.28027684723519,
0.361233179640555));
#29573=CARTESIAN_POINT('Ctrl Pts',(-8.32661228091193,-1.54198354601843,
-1.71826617667884));
#29574=CARTESIAN_POINT('Ctrl Pts',(-8.2155907838331,0.604998744749697,-2.22803241200872));
#29575=CARTESIAN_POINT('Ctrl Pts',(-8.10456928675428,2.1992805397039,-0.702365302239374));
#29576=CARTESIAN_POINT('Ctrl Pts',(-7.99354778967544,1.78439544749182,1.46495214839276));
#29577=CARTESIAN_POINT('Ctrl Pts',(-7.88252629259663,-0.260635586535173,
2.29395313839267));
#29578=CARTESIAN_POINT('Ctrl Pts',(-7.77150479551778,-2.06756130355966,
1.02729847957288));
#29579=CARTESIAN_POINT('Ctrl Pts',(-7.66048329843898,-1.98565308907595,
-1.1778513148752));
#29580=CARTESIAN_POINT('Ctrl Pts',(-7.54946180136014,-0.0897387194211616,
-2.30696746235112));
#29581=CARTESIAN_POINT('Ctrl Pts',(-7.43844030428132,1.88815703473765,-1.32853864162123));
#29582=CARTESIAN_POINT('Ctrl Pts',(-7.3274188072025,2.1411147814535,0.863585202948405));
#29583=CARTESIAN_POINT('Ctrl Pts',(-7.21639731012367,0.438043343689854,
2.26677522907745));
#29584=CARTESIAN_POINT('Ctrl Pts',(-7.10537581304484,-1.66520540906234,
1.59913816030374));
#29585=CARTESIAN_POINT('Ctrl Pts',(-6.99435431596602,-2.24719504647279,
-0.529401863633136));
#29586=CARTESIAN_POINT('Ctrl Pts',(-6.88333281888719,-0.776245190777431,
-2.17430340888869));
#29587=CARTESIAN_POINT('Ctrl Pts',(-6.77231132180837,1.40384845329613,-1.83285608553649));
#29588=CARTESIAN_POINT('Ctrl Pts',(-6.66128982472955,2.30144731053276,0.183008707310951));
#29589=CARTESIAN_POINT('Ctrl Pts',(-6.5502683276507,1.09654416977377,2.03168471812071));
#29590=CARTESIAN_POINT('Ctrl Pts',(-6.4392468305719,-1.1101139524217,2.02430208287913));
#29591=CARTESIAN_POINT('Ctrl Pts',(-6.32822533349305,-2.302620330935,0.16760525551085));
#29592=CARTESIAN_POINT('Ctrl Pts',(-6.21720383641425,-1.39155309111705,
-1.84220843139767));
#29593=CARTESIAN_POINT('Ctrl Pts',(-6.10618233933541,0.790776428311071,
-2.16906075307671));
#29594=CARTESIAN_POINT('Ctrl Pts',(-5.99516084225658,2.25068705381848,-0.514353668096137));
#29595=CARTESIAN_POINT('Ctrl Pts',(-5.88413934517776,1.65446804044193,1.61024451971318));
#29596=CARTESIAN_POINT('Ctrl Pts',(-5.77311784809893,-0.453200896089194,
2.26379346626278));
#29597=CARTESIAN_POINT('Ctrl Pts',(-5.66209635102011,-2.14684523811403,
0.849239326513562));
#29598=CARTESIAN_POINT('Ctrl Pts',(-5.55107485394128,-1.87922530010751,
-1.34114286395817));
#29599=CARTESIAN_POINT('Ctrl Pts',(-5.44005335686246,0.105173001704038,
-2.30631536217895));
#29600=CARTESIAN_POINT('Ctrl Pts',(-5.32903185978363,1.99348983112823,-1.16453862250183));
#29601=CARTESIAN_POINT('Ctrl Pts',(-5.21801036270481,2.06064119925807,1.04110986837623));
#29602=CARTESIAN_POINT('Ctrl Pts',(-5.10698886562598,0.245280541688206,
2.29564574052253));
#29603=CARTESIAN_POINT('Ctrl Pts',(-4.99596736854716,-1.79415773287021,
1.45297967628323));
#29604=CARTESIAN_POINT('Ctrl Pts',(-4.88494587146833,-2.19453166699596,
-0.717065319662008));
#29605=CARTESIAN_POINT('Ctrl Pts',(-4.77392437438951,-0.590077077171925,
-2.23203067924847));
#29606=CARTESIAN_POINT('Ctrl Pts',(-4.66290287731068,1.55344622304472,-1.70791005097405));
#29607=CARTESIAN_POINT('Ctrl Pts',(-4.55188138023186,2.27780873136201,0.376482793021167));
#29608=CARTESIAN_POINT('Ctrl Pts',(-4.44085988315303,0.921264417775247,
2.11693735917044));
#29609=CARTESIAN_POINT('Ctrl Pts',(-4.3298383860742,-1.27690693206398,1.92345018052377));
#29610=CARTESIAN_POINT('Ctrl Pts',(-4.21881688899537,-2.30855173852655,
-0.0272172859738563));
#29611=CARTESIAN_POINT('Ctrl Pts',(-4.10779539191655,-1.23120425109033,
-1.95302022575508));
#29612=CARTESIAN_POINT('Ctrl Pts',(-3.99677389483772,0.970917801469463,
-2.09462897261033));
#29613=CARTESIAN_POINT('Ctrl Pts',(-3.88575239775891,2.28605164963331,-0.322675944744844));
#29614=CARTESIAN_POINT('Ctrl Pts',(-3.77473090068007,1.51274830487346,1.74405976853459));
#29615=CARTESIAN_POINT('Ctrl Pts',(-3.66370940360125,-0.642535986794508,
2.21749845902402));
#29616=CARTESIAN_POINT('Ctrl Pts',(-3.55268790652242,-2.21082739365792,
0.665127164948678));
#29617=CARTESIAN_POINT('Ctrl Pts',(-3.4416664094436,-1.75940321064622,-1.49487533009738));
#29618=CARTESIAN_POINT('Ctrl Pts',(-3.33064491236477,0.299335095435475,
-2.28922484930345));
#29619=CARTESIAN_POINT('Ctrl Pts',(-3.21962341528595,2.08461389911976,-0.992238278678359));
#29620=CARTESIAN_POINT('Ctrl Pts',(-3.10860191820712,1.96548026299592,1.21121395560337));
#29621=CARTESIAN_POINT('Ctrl Pts',(-2.99758042112829,0.050769486586585,
2.30815388756997));
#29622=CARTESIAN_POINT('Ctrl Pts',(-2.88655892404947,-1.91032208061755,
1.2964649854169));
#29623=CARTESIAN_POINT('Ctrl Pts',(-2.77553742697064,-2.12622662072629,
-0.8996178464995));
#29624=CARTESIAN_POINT('Ctrl Pts',(-2.66451592989181,-0.399703150196944,
-2.27384900489376));
#29625=CARTESIAN_POINT('Ctrl Pts',(-2.55349443281299,1.69197170262792,-1.5707907782725));
#29626=CARTESIAN_POINT('Ctrl Pts',(-2.44247293573417,2.23793492468817,0.567273476545088));
#29627=CARTESIAN_POINT('Ctrl Pts',(-2.33145143865534,0.739418289337298,
2.18710138509976));
#29628=CARTESIAN_POINT('Ctrl Pts',(-2.22042994157651,-1.43459866614401,
1.80888877426244));
#29629=CARTESIAN_POINT('Ctrl Pts',(-2.10940844449769,-2.29802880948203,
-0.221845857900401));
#29630=CARTESIAN_POINT('Ctrl Pts',(-1.99838694741886,-1.06207989233547,
-2.04991169691596));
#29631=CARTESIAN_POINT('Ctrl Pts',(-1.88736545034004,1.14413883704918,-2.00526767278129));
#29632=CARTESIAN_POINT('Ctrl Pts',(-1.77634395326121,2.30512237374665,-0.128698166199081));
#29633=CARTESIAN_POINT('Ctrl Pts',(-1.66532245618239,1.36024614796476,1.86544381076144));
#29634=CARTESIAN_POINT('Ctrl Pts',(-1.55430095910356,-0.827290961865428,
2.1553986720195));
#29635=CARTESIAN_POINT('Ctrl Pts',(-1.44327946202473,-2.25905249185057,
0.476273153560824));
#29636=CARTESIAN_POINT('Ctrl Pts',(-1.33225796494591,-1.62703941662637,
-1.63795085746574));
#29637=CARTESIAN_POINT('Ctrl Pts',(-1.22123646786708,0.491360911049524,
-2.25582176774822));
#29638=CARTESIAN_POINT('Ctrl Pts',(-1.11021497078826,2.16088497545151,-0.812858021785275));
#29639=CARTESIAN_POINT('Ctrl Pts',(-0.999193473709431,1.85630028593178,
1.37267043894513));
#29640=CARTESIAN_POINT('Ctrl Pts',(-0.888171976630606,-0.144084490198471,
2.30423829946203));
#29641=CARTESIAN_POINT('Ctrl Pts',(-0.777150479551781,-2.01290653192051,
1.13065678261724));
#29642=CARTESIAN_POINT('Ctrl Pts',(-0.666128982472955,-2.04269814678982,
-1.07565765858493));
#29643=CARTESIAN_POINT('Ctrl Pts',(-0.555107485394129,-0.206610916552875,
-2.2996518687847));
#29644=CARTESIAN_POINT('Ctrl Pts',(-0.444085988315305,1.81868635599406,
-1.42211079441787));
#29645=CARTESIAN_POINT('Ctrl Pts',(-0.333064491236478,2.18163438183212,
0.753324392930728));
#29646=CARTESIAN_POINT('Ctrl Pts',(-0.222042994157653,0.553226055458001,
2.24302138042127));
#29647=CARTESIAN_POINT('Ctrl Pts',(-0.111021497078828,-1.58398475473698,
1.67871039460253));
#29648=CARTESIAN_POINT('Ctrl Pts',(-0.0370071656929422,-2.03883201741979,
0.287355495504613));
#29649=CARTESIAN_POINT('Ctrl Pts',(0.,-1.92218901323832,-0.351148682734097));
#29650=CARTESIAN_POINT('Ctrl Pts',(-15.7993827215147,1.05793541951259,-1.48236995244726));
#29651=CARTESIAN_POINT('Ctrl Pts',(-15.7623755558218,1.55034246263605,-1.13094968055241));
#29652=CARTESIAN_POINT('Ctrl Pts',(-15.6883612244359,2.14904710443863,0.0949702857508803));
#29653=CARTESIAN_POINT('Ctrl Pts',(-15.5773397273571,1.08561464780462,1.85947873778831));
#29654=CARTESIAN_POINT('Ctrl Pts',(-15.4663182302782,-0.970482091465297,
1.91977702456333));
#29655=CARTESIAN_POINT('Ctrl Pts',(-15.3552967331994,-2.1395185329741,0.228996997483074));
#29656=CARTESIAN_POINT('Ctrl Pts',(-15.2442752361206,-1.35423117190993,
-1.6724127799477));
#29657=CARTESIAN_POINT('Ctrl Pts',(-15.1332537390418,0.668352646562777,
-2.04523047030762));
#29658=CARTESIAN_POINT('Ctrl Pts',(-15.0222322419629,2.08029037091456,-0.550007866879181));
#29659=CARTESIAN_POINT('Ctrl Pts',(-14.9112107448841,1.59180129537846,1.44788452227822));
#29660=CARTESIAN_POINT('Ctrl Pts',(-14.8001892478053,-0.350906933858996,
2.12294415771364));
#29661=CARTESIAN_POINT('Ctrl Pts',(-14.6891677507265,-1.97303197729494,
0.858631526263166));
#29662=CARTESIAN_POINT('Ctrl Pts',(-14.5781462536476,-1.7926861645986,-1.19011942496844));
#29663=CARTESIAN_POINT('Ctrl Pts',(-14.4671247565688,0.0253823607806043,
-2.15161337368581));
#29664=CARTESIAN_POINT('Ctrl Pts',(-14.35610325949,1.82026123117149,-1.14749535433649));
#29665=CARTESIAN_POINT('Ctrl Pts',(-14.2450817624112,1.9522294968358,0.90492877585299));
#29666=CARTESIAN_POINT('Ctrl Pts',(-14.1340602653323,0.300725548605529,
2.1306471165121));
#29667=CARTESIAN_POINT('Ctrl Pts',(-14.0230387682535,-1.62550795109711,
1.40990027548872));
#29668=CARTESIAN_POINT('Ctrl Pts',(-13.9120172711747,-2.06674831305342,
-0.598870664077681));
#29669=CARTESIAN_POINT('Ctrl Pts',(-13.8009957740958,-0.619897398695016,
-2.06053912400966));
#29670=CARTESIAN_POINT('Ctrl Pts',(-13.689974277017,1.39326474242623,-1.63978898384522));
#29671=CARTESIAN_POINT('Ctrl Pts',(-13.5789527799382,2.13360092975018,0.279001024356398));
#29672=CARTESIAN_POINT('Ctrl Pts',(-13.4679312828594,0.9247722518186,1.94290780360304));
#29673=CARTESIAN_POINT('Ctrl Pts',(-13.3569097857805,-1.12888806234094,
1.83185868350156));
#29674=CARTESIAN_POINT('Ctrl Pts',(-13.2458882887017,-2.15124542621297,
0.0473032636800278));
#29675=CARTESIAN_POINT('Ctrl Pts',(-13.1348667916229,-1.20831868869478,
-1.7804663500513));
#29676=CARTESIAN_POINT('Ctrl Pts',(-13.0238452945441,0.838475360538852,
-1.98167947787823));
#29677=CARTESIAN_POINT('Ctrl Pts',(-12.9128237974652,2.11927484975544,-0.372516566684666));
#29678=CARTESIAN_POINT('Ctrl Pts',(-12.8018023003864,1.46399716443733,1.576961249755));
#29679=CARTESIAN_POINT('Ctrl Pts',(-12.6907808033076,-0.528724549683909,
2.08579597088056));
#29680=CARTESIAN_POINT('Ctrl Pts',(-12.5797593062288,-2.03842654968845,
0.689138362566185));
#29681=CARTESIAN_POINT('Ctrl Pts',(-12.4687378091499,-1.68591086001068,
-1.33708603062395));
#29682=CARTESIAN_POINT('Ctrl Pts',(-12.3577163120711,0.206779542927678,
-2.1418068778343));
#29683=CARTESIAN_POINT('Ctrl Pts',(-12.2466948149923,1.91056516401672,-0.989866271423035));
#29684=CARTESIAN_POINT('Ctrl Pts',(-12.1356733179135,1.86894168698282,1.066373036002));
#29685=CARTESIAN_POINT('Ctrl Pts',(-12.0246518208346,0.119934507080401,
2.14842039537931));
#29686=CARTESIAN_POINT('Ctrl Pts',(-11.9136303237558,-1.73863961342216,
1.26776447966517));
#29687=CARTESIAN_POINT('Ctrl Pts',(-11.802608826677,-2.00886832871558,-0.771065833211139));
#29688=CARTESIAN_POINT('Ctrl Pts',(-11.6915873295982,-0.443882457299119,
-2.10548399313942));
#29689=CARTESIAN_POINT('Ctrl Pts',(-11.5805658325193,1.5266150889125,-1.51642370449935));
#29690=CARTESIAN_POINT('Ctrl Pts',(-11.4695443354405,2.10246359844209,0.45797521602046));
#29691=CARTESIAN_POINT('Ctrl Pts',(-11.3585228383617,0.757592960413117,
2.01398793134313));
#29692=CARTESIAN_POINT('Ctrl Pts',(-11.2475013412829,-1.27938160093674,
1.73010901403572));
#29693=CARTESIAN_POINT('Ctrl Pts',(-11.136479844204,-2.14756886923941,-0.134322124525075));
#29694=CARTESIAN_POINT('Ctrl Pts',(-11.0254583471252,-1.05383077964032,
-1.8760424220006));
#29695=CARTESIAN_POINT('Ctrl Pts',(-10.9144368500464,1.00264119902189,-1.9038920944442));
#29696=CARTESIAN_POINT('Ctrl Pts',(-10.8034153529675,2.14314385934751,-0.19242889441091));
#29697=CARTESIAN_POINT('Ctrl Pts',(-10.6923938558887,1.32576365802854,1.6948289601945));
#29698=CARTESIAN_POINT('Ctrl Pts',(-10.5813723588099,-0.702776463014917,
2.03376491372415));
#29699=CARTESIAN_POINT('Ctrl Pts',(-10.4703508617311,-2.0892906246237,0.51474184512501));
#29700=CARTESIAN_POINT('Ctrl Pts',(-10.3593293646523,-1.56711989366027,
-1.47452694792513));
#29701=CARTESIAN_POINT('Ctrl Pts',(-10.2483078675734,0.386703298969398,
-2.11673216062622));
#29702=CARTESIAN_POINT('Ctrl Pts',(-10.1372863704946,1.98725120478555,-0.8251830889818));
#29703=CARTESIAN_POINT('Ctrl Pts',(-10.0262648734158,1.77233298654189,1.22021730281073));
#29704=CARTESIAN_POINT('Ctrl Pts',(-9.91524337633695,-0.0617114347062867,
2.1508803267708));
#29705=CARTESIAN_POINT('Ctrl Pts',(-9.80422187925813,-1.83937897772859,
1.11659278949547));
#29706=CARTESIAN_POINT('Ctrl Pts',(-9.6932003821793,-1.93667002112544,-0.937765274755445));
#29707=CARTESIAN_POINT('Ctrl Pts',(-9.58217888510048,-0.264703706233324,
-2.13542183869359));
#29708=CARTESIAN_POINT('Ctrl Pts',(-9.47115738802165,1.64908438258572,-1.38225004263882));
#29709=CARTESIAN_POINT('Ctrl Pts',(-9.36013589094283,2.05634082352307,0.633685173233227));
#29710=CARTESIAN_POINT('Ctrl Pts',(-9.249114393864,0.585013874681943,2.07071322198242));
#29711=CARTESIAN_POINT('Ctrl Pts',(-9.13809289678517,-1.42075626334053,
1.61602788386891));
#29712=CARTESIAN_POINT('Ctrl Pts',(-9.02707139970635,-2.12858537587554,
-0.314990125038813));
#29713=CARTESIAN_POINT('Ctrl Pts',(-8.91604990262752,-0.891831623010708,
-1.95824687857819));
#29714=CARTESIAN_POINT('Ctrl Pts',(-8.8050284055487,1.15966064707945,-1.81253459687766));
#29715=CARTESIAN_POINT('Ctrl Pts',(-8.69400690846987,2.15173747180057,-0.0109696723941425));
#29716=CARTESIAN_POINT('Ctrl Pts',(-8.58298541139105,1.1780806849295,1.80061666688365));
#29717=CARTESIAN_POINT('Ctrl Pts',(-8.47196391431222,-0.871819291402609,
1.96723806500419));
#29718=CARTESIAN_POINT('Ctrl Pts',(-8.36094241723339,-2.12526314480885,
0.336676471676244));
#29719=CARTESIAN_POINT('Ctrl Pts',(-8.24992092015458,-1.43715917838138,
-1.60145807852011));
#29720=CARTESIAN_POINT('Ctrl Pts',(-8.13889942307573,0.563870802105082,
-2.07657029734043));
#29721=CARTESIAN_POINT('Ctrl Pts',(-8.02787792599693,2.04977298339684,-0.654618360420469));
#29722=CARTESIAN_POINT('Ctrl Pts',(-7.91685642891809,1.66309186751476,1.36536439146091));
#29723=CARTESIAN_POINT('Ctrl Pts',(-7.80583493183928,-0.242917524229776,
2.13800971880047));
#29724=CARTESIAN_POINT('Ctrl Pts',(-7.69481343476043,-1.92700804878851,
0.957462511625111));
#29725=CARTESIAN_POINT('Ctrl Pts',(-7.58379193768163,-1.85066797205159,
-1.09778073333686));
#29726=CARTESIAN_POINT('Ctrl Pts',(-7.47277044060278,-0.0836382622923028,
-2.15013932626328));
#29727=CARTESIAN_POINT('Ctrl Pts',(-7.36174894352397,1.75979972011074,-1.23822430373551));
#29728=CARTESIAN_POINT('Ctrl Pts',(-7.25072744644514,1.99556134569621,0.80487849817616));
#29729=CARTESIAN_POINT('Ctrl Pts',(-7.13970594936632,0.408265064525669,
2.11267936950949));
#29730=CARTESIAN_POINT('Ctrl Pts',(-7.02868445228748,-1.55200439311022,
1.49042840989756));
#29731=CARTESIAN_POINT('Ctrl Pts',(-6.91766295520867,-2.09443025186013,
-0.493413012957979));
#29732=CARTESIAN_POINT('Ctrl Pts',(-6.80664145812983,-0.723475878507756,
-2.02649380321791));
#29733=CARTESIAN_POINT('Ctrl Pts',(-6.69561996105102,1.30841453848234,-1.70825814113419));
#29734=CARTESIAN_POINT('Ctrl Pts',(-6.58459846397218,2.14499443553322,0.170567736675779));
#29735=CARTESIAN_POINT('Ctrl Pts',(-6.47357696689336,1.02200086515847,1.89357036121674));
#29736=CARTESIAN_POINT('Ctrl Pts',(-6.36255546981454,-1.03464817111157,
1.88668959908053));
#29737=CARTESIAN_POINT('Ctrl Pts',(-6.2515339727357,-2.14608771376038,0.156211414787358));
#29738=CARTESIAN_POINT('Ctrl Pts',(-6.14051247565689,-1.29695501762504,
-1.71697471254541));
#29739=CARTESIAN_POINT('Ctrl Pts',(-6.02949097857805,0.737019279440051,
-2.02160754425701));
#29740=CARTESIAN_POINT('Ctrl Pts',(-5.91846948149923,2.09768487180779,-0.479387796936746));
#29741=CARTESIAN_POINT('Ctrl Pts',(-5.8074479844204,1.54199695307992,1.500779756645));
#29742=CARTESIAN_POINT('Ctrl Pts',(-5.69642648734159,-0.42239220330661,
2.1099003075617));
#29743=CARTESIAN_POINT('Ctrl Pts',(-5.58540499026275,-2.00090224470079,
0.791507857455957));
#29744=CARTESIAN_POINT('Ctrl Pts',(-5.47438349318393,-1.7514751666901,-1.2499716883718));
#29745=CARTESIAN_POINT('Ctrl Pts',(-5.36336199610511,0.0980233188007598,
-2.14953155599876));
#29746=CARTESIAN_POINT('Ctrl Pts',(-5.25234049902627,1.85797197072144,-1.08537304060708));
#29747=CARTESIAN_POINT('Ctrl Pts',(-5.14131900194746,1.92055837464115,0.970334999296067));
#29748=CARTESIAN_POINT('Ctrl Pts',(-5.03029750486862,0.228606318579576,
2.1395872574795));
#29749=CARTESIAN_POINT('Ctrl Pts',(-4.91927600778981,-1.6721905106681,1.35420581053794));
#29750=CARTESIAN_POINT('Ctrl Pts',(-4.80825451071097,-2.04534694006012,
-0.668319067549202));
#29751=CARTESIAN_POINT('Ctrl Pts',(-4.69723301363215,-0.549963512645648,
-2.08029676152747));
#29752=CARTESIAN_POINT('Ctrl Pts',(-4.58621151655332,1.44784262019871,-1.59180596443137));
#29753=CARTESIAN_POINT('Ctrl Pts',(-4.4751900194745,2.12296281197481,0.350889413113472));
#29754=CARTESIAN_POINT('Ctrl Pts',(-4.36416852239567,0.858636667778067,
1.97302750969425));
#29755=CARTESIAN_POINT('Ctrl Pts',(-4.25314702531685,-1.19010252871572,
1.79269363038069));
#29756=CARTESIAN_POINT('Ctrl Pts',(-4.14212552823802,-2.15161590300918,
-0.0253670491160354));
#29757=CARTESIAN_POINT('Ctrl Pts',(-4.03110403115919,-1.14750672566223,
-1.82025349768217));
#29758=CARTESIAN_POINT('Ctrl Pts',(-3.92008253408037,0.904914603945486,
-1.95223565197143));
#29759=CARTESIAN_POINT('Ctrl Pts',(-3.80906103700155,2.13064537491839,-0.300740365764828));
#29760=CARTESIAN_POINT('Ctrl Pts',(-3.69803953992272,1.40991135511363,1.62549821654534));
#29761=CARTESIAN_POINT('Ctrl Pts',(-3.5870180428439,-0.598856254495366,
2.0667524447079));
#29762=CARTESIAN_POINT('Ctrl Pts',(-3.47599654576507,-2.06053487977653,
0.619911679579849));
#29763=CARTESIAN_POINT('Ctrl Pts',(-3.36497504868625,-1.63979860821658,
-1.39325338894354));
#29764=CARTESIAN_POINT('Ctrl Pts',(-3.25395355160741,0.278986232328857,
-2.13360285980372));
#29765=CARTESIAN_POINT('Ctrl Pts',(-3.1429320545286,1.94290140529526,-0.92478571060375));
#29766=CARTESIAN_POINT('Ctrl Pts',(-3.03191055744976,1.83186649895568,1.12887537469107));
#29767=CARTESIAN_POINT('Ctrl Pts',(-2.92088906037094,0.0473181661490567,
2.15124509804478));
#29768=CARTESIAN_POINT('Ctrl Pts',(-2.80986756329212,-1.78045798148312,
1.20833102146455));
#29769=CARTESIAN_POINT('Ctrl Pts',(-2.69884606621329,-1.98168528528455,
-0.838461634996595));
#29770=CARTESIAN_POINT('Ctrl Pts',(-2.58782456913446,-0.372531245496584,
-2.11927226854948));
#29771=CARTESIAN_POINT('Ctrl Pts',(-2.47680307205564,1.57695110837729,-1.46400808889317));
#29772=CARTESIAN_POINT('Ctrl Pts',(-2.36578157497681,2.08579963511323,0.528710105613121));
#29773=CARTESIAN_POINT('Ctrl Pts',(-2.25476007789799,0.689152477617587,
2.03842177029897));
#29774=CARTESIAN_POINT('Ctrl Pts',(-2.14373858081916,-1.33707434535616,
1.6859201327504));
#29775=CARTESIAN_POINT('Ctrl Pts',(-2.03271708374034,-2.14180832490704,
-0.206764729552862));
#29776=CARTESIAN_POINT('Ctrl Pts',(-1.92169558666151,-0.989879476590722,
-1.9105582661379));
#29777=CARTESIAN_POINT('Ctrl Pts',(-1.81067408958268,1.06636003688472,-1.86894915220754));
#29778=CARTESIAN_POINT('Ctrl Pts',(-1.69965259250385,2.14841966717244,-0.119949237637093));
#29779=CARTESIAN_POINT('Ctrl Pts',(-1.58863109542503,1.26777632709065,1.738630545905));
#29780=CARTESIAN_POINT('Ctrl Pts',(-1.4776095983462,-0.771051547279393,
2.00887421436004));
#29781=CARTESIAN_POINT('Ctrl Pts',(-1.36658810126738,-2.1054816255929,0.443896003834786));
#29782=CARTESIAN_POINT('Ctrl Pts',(-1.25556660418855,-1.51643293291336,
-1.52660261169636));
#29783=CARTESIAN_POINT('Ctrl Pts',(-1.14454510710973,0.457958092377877,
-2.10247052679843));
#29784=CARTESIAN_POINT('Ctrl Pts',(-1.0335236100309,2.01398755772421,-0.757599761518903));
#29785=CARTESIAN_POINT('Ctrl Pts',(-0.922502112952076,1.73010859982741,
1.27935601214206));
#29786=CARTESIAN_POINT('Ctrl Pts',(-0.811480615873251,-0.13428959607632,
2.1475956924447));
#29787=CARTESIAN_POINT('Ctrl Pts',(-0.700459118794427,-1.87606872008661,
1.05379449536493));
#29788=CARTESIAN_POINT('Ctrl Pts',(-0.589437621715599,-1.90383509467522,
-1.00253422341843));
#29789=CARTESIAN_POINT('Ctrl Pts',(-0.478416124636775,-0.192565462740806,
-2.14332104829499));
#29790=CARTESIAN_POINT('Ctrl Pts',(-0.367394627557949,1.6950516728034,-1.32543540179154));
#29791=CARTESIAN_POINT('Ctrl Pts',(-0.256373130479123,2.03332641506991,
0.70211324134716));
#29792=CARTESIAN_POINT('Ctrl Pts',(-0.145351633400297,0.515617631183002,
2.09054031250966));
#29793=CARTESIAN_POINT('Ctrl Pts',(-0.0343301363214737,-1.47630513604666,
1.56459130687665));
#29794=CARTESIAN_POINT('Ctrl Pts',(0.0396841950644127,-1.90023178559759,
0.267821008135351));
#29795=CARTESIAN_POINT('Ctrl Pts',(0.0766913607573549,-1.79151819751408,
-0.32727752100269));
#29796=CARTESIAN_POINT('Ctrl Pts',(-15.7226913607574,0.98077109908141,-1.37424797458504));
#29797=CARTESIAN_POINT('Ctrl Pts',(-15.6856841950644,1.43726266555351,-1.04845980269021));
#29798=CARTESIAN_POINT('Ctrl Pts',(-15.6116698636785,1.99229863347336,0.0880432867810469));
#29799=CARTESIAN_POINT('Ctrl Pts',(-15.5006483665997,1.00643144342095,1.72385097591248));
#29800=CARTESIAN_POINT('Ctrl Pts',(-15.3896268695209,-0.899696493689348,
1.77975119052132));
#29801=CARTESIAN_POINT('Ctrl Pts',(-15.2786053724421,-1.98346506259976,
0.212294278805113));
#29802=CARTESIAN_POINT('Ctrl Pts',(-15.1675838753632,-1.25545545634186,
-1.55042934573719));
#29803=CARTESIAN_POINT('Ctrl Pts',(-15.0565623782844,0.619603945243983,
-1.89605423851159));
#29804=CARTESIAN_POINT('Ctrl Pts',(-14.9455408812056,1.92855691931587,-0.509891067217538));
#29805=CARTESIAN_POINT('Ctrl Pts',(-14.8345193841267,1.47569754938993,1.34227786315351));
#29806=CARTESIAN_POINT('Ctrl Pts',(-14.7234978870479,-0.325312276012785,
1.968099598942));
#29807=CARTESIAN_POINT('Ctrl Pts',(-14.6124763899691,-1.82912180195825,
0.796004151280846));
#29808=CARTESIAN_POINT('Ctrl Pts',(-14.5014548928903,-1.66193015899916,
-1.1033137892313));
#29809=CARTESIAN_POINT('Ctrl Pts',(-14.3904333958114,0.023531007111521,
-1.99467772265372));
#29810=CARTESIAN_POINT('Ctrl Pts',(-14.2794118987326,1.68749393902876,-1.06379865831688));
#29811=CARTESIAN_POINT('Ctrl Pts',(-14.1683904016538,1.80983662514383,0.83892454465003));
#29812=CARTESIAN_POINT('Ctrl Pts',(-14.057368904575,0.278791050368257,1.97524071476778));
#29813=CARTESIAN_POINT('Ctrl Pts',(-13.9463474074961,-1.50694568908335,
1.30706413386114));
#29814=CARTESIAN_POINT('Ctrl Pts',(-13.8353259104173,-1.91600260009437,
-0.555189880763887));
#29815=CARTESIAN_POINT('Ctrl Pts',(-13.7243044133385,-0.574682954953825,
-1.91024630055989));
#29816=CARTESIAN_POINT('Ctrl Pts',(-13.6132829162597,1.29164197316535,-1.52018508340368));
#29817=CARTESIAN_POINT('Ctrl Pts',(-13.5022614191808,1.97797908102583,0.25865108234011));
#29818=CARTESIAN_POINT('Ctrl Pts',(-13.391239922102,0.857320665408837,1.80119484309498));
#29819=CARTESIAN_POINT('Ctrl Pts',(-13.2802184250232,-1.04654855600932,
1.69824548950954));
#29820=CARTESIAN_POINT('Ctrl Pts',(-13.1691969279444,-1.99433661275166,
0.0438530302076145));
#29821=CARTESIAN_POINT('Ctrl Pts',(-13.0581754308656,-1.1201856242773,-1.65060164052528));
#29822=CARTESIAN_POINT('Ctrl Pts',(-12.9471539337867,0.777318147914217,
-1.83713856602054));
#29823=CARTESIAN_POINT('Ctrl Pts',(-12.8361324367079,1.96469792514163,-0.345345732636185));
#29824=CARTESIAN_POINT('Ctrl Pts',(-12.725110939629,1.35721527187243,1.46193991580655));
#29825=CARTESIAN_POINT('Ctrl Pts',(-12.6140894425503,-0.490160125221753,
1.93366094856961));
#29826=CARTESIAN_POINT('Ctrl Pts',(-12.5030679454714,-1.88974658628572,
0.638873580378455));
#29827=CARTESIAN_POINT('Ctrl Pts',(-12.3920464483926,-1.56294289483922,
-1.23956085752912));
#29828=CARTESIAN_POINT('Ctrl Pts',(-12.2810249513137,0.19169733411343,-1.98558649880676));
#29829=CARTESIAN_POINT('Ctrl Pts',(-12.170003454235,1.77121123011709,-0.917666818844631));
#29830=CARTESIAN_POINT('Ctrl Pts',(-12.0589819571561,1.73262371091205,0.988593287700225));
#29831=CARTESIAN_POINT('Ctrl Pts',(-11.9479604600773,0.111186652944486,
1.99171763569072));
#29832=CARTESIAN_POINT('Ctrl Pts',(-11.8369389629984,-1.61182568719379,
1.17529552292561));
#29833=CARTESIAN_POINT('Ctrl Pts',(-11.7259174659196,-1.86234430034674,
-0.71482537662935));
#29834=CARTESIAN_POINT('Ctrl Pts',(-11.6148959688408,-0.41150629563833,
-1.95191295419624));
#29835=CARTESIAN_POINT('Ctrl Pts',(-11.503874471762,1.41526593307254,-1.40581789389388));
#29836=CARTESIAN_POINT('Ctrl Pts',(-11.3928529746831,1.94911286283686,0.424571148374424));
#29837=CARTESIAN_POINT('Ctrl Pts',(-11.2818314776043,0.702335196209829,
1.8670904863646));
#29838=CARTESIAN_POINT('Ctrl Pts',(-11.1708099805255,-1.186065307723,1.60391729771957));
#29839=CARTESIAN_POINT('Ctrl Pts',(-11.0597884834467,-1.99092821866891,
-0.124524857823653));
#29840=CARTESIAN_POINT('Ctrl Pts',(-10.9487669863679,-0.976965845864036,
-1.73920652831208));
#29841=CARTESIAN_POINT('Ctrl Pts',(-10.837745489289,0.929509961205432,-1.76502488484668));
#29842=CARTESIAN_POINT('Ctrl Pts',(-10.7267239922102,1.98682596277023,-0.1783934017006));
#29843=CARTESIAN_POINT('Ctrl Pts',(-10.6157024951314,1.22906432285431,1.57121052134806));
#29844=CARTESIAN_POINT('Ctrl Pts',(-10.5046809980525,-0.651516936976405,
1.88542496348729));
#29845=CARTESIAN_POINT('Ctrl Pts',(-10.3936595009737,-1.93690070718752,
0.477197299452391));
#29846=CARTESIAN_POINT('Ctrl Pts',(-10.2826380038949,-1.45281637437343,
-1.36697702777355));
#29847=CARTESIAN_POINT('Ctrl Pts',(-10.1716165068161,0.358497704636228,
-1.9623406961786));
#29848=CARTESIAN_POINT('Ctrl Pts',(-10.0605950097373,1.84230389900958,-0.76499539593535));
#29849=CARTESIAN_POINT('Ctrl Pts',(-9.94957351265842,1.64306151310234,1.13121637022721));
#29850=CARTESIAN_POINT('Ctrl Pts',(-9.8385520155796,-0.0572102895190575,
1.99399814314891));
#29851=CARTESIAN_POINT('Ctrl Pts',(-9.72753051850077,-1.70521726406064,
1.03515008305931));
#29852=CARTESIAN_POINT('Ctrl Pts',(-9.61650902142195,-1.79541203569147,
-0.869365995540654));
#29853=CARTESIAN_POINT('Ctrl Pts',(-9.50548752434313,-0.245396590477122,
-1.97966717543389));
#29854=CARTESIAN_POINT('Ctrl Pts',(-9.39446602726429,1.52880248884355,-1.28143067007698));
#29855=CARTESIAN_POINT('Ctrl Pts',(-9.28344453018548,1.90635421820158,0.587465068623835));
#29856=CARTESIAN_POINT('Ctrl Pts',(-9.17242303310664,0.542343786082916,
1.91967831414678));
#29857=CARTESIAN_POINT('Ctrl Pts',(-9.06140153602782,-1.3171283012391,1.49815708461536));
#29858=CARTESIAN_POINT('Ctrl Pts',(-8.95038003894899,-1.9733293545913,-0.292015188674224));
#29859=CARTESIAN_POINT('Ctrl Pts',(-8.83935854187017,-0.82678267970151,
-1.81541510753154));
#29860=CARTESIAN_POINT('Ctrl Pts',(-8.72833704479135,1.0750766317301,-1.6803308745649));
#29861=CARTESIAN_POINT('Ctrl Pts',(-8.61731554771252,1.99479276922667,-0.0101695599297692));
#29862=CARTESIAN_POINT('Ctrl Pts',(-8.50629405063369,1.09215313794598,1.6692822216099));
#29863=CARTESIAN_POINT('Ctrl Pts',(-8.39527255355487,-0.808230019393109,
1.82375048947492));
#29864=CARTESIAN_POINT('Ctrl Pts',(-8.28425105647603,-1.97024944238251,
0.312119763711931));
#29865=CARTESIAN_POINT('Ctrl Pts',(-8.17322955939722,-1.33233481074433,
-1.48464998036137));
#29866=CARTESIAN_POINT('Ctrl Pts',(-8.06220806231839,0.52274285946047,-1.92510818267215));
#29867=CARTESIAN_POINT('Ctrl Pts',(-7.95118656523957,1.90026542708978,-0.606871418601563));
#29868=CARTESIAN_POINT('Ctrl Pts',(-7.84016506816073,1.54178828753771,1.26577663452906));
#29869=CARTESIAN_POINT('Ctrl Pts',(-7.72914357108192,-0.225199461924381,
1.98206629920827));
#29870=CARTESIAN_POINT('Ctrl Pts',(-7.61812207400307,-1.78645479401735,
0.88762654367734));
#29871=CARTESIAN_POINT('Ctrl Pts',(-7.50710057692427,-1.71568285502723,
-1.01771015179853));
#29872=CARTESIAN_POINT('Ctrl Pts',(-7.39607907984543,-0.0775378051634432,
-1.99331119017544));
#29873=CARTESIAN_POINT('Ctrl Pts',(-7.28505758276661,1.63144240548383,-1.14790996584979));
#29874=CARTESIAN_POINT('Ctrl Pts',(-7.17403608568779,1.85000790993892,0.746171793403911));
#29875=CARTESIAN_POINT('Ctrl Pts',(-7.06301458860896,0.378486785361485,
1.95858350994154));
#29876=CARTESIAN_POINT('Ctrl Pts',(-6.95199309153013,-1.4388033771581,1.38171865949137));
#29877=CARTESIAN_POINT('Ctrl Pts',(-6.8409715944513,-1.94166545724747,-0.457424162282821));
#29878=CARTESIAN_POINT('Ctrl Pts',(-6.72995009737248,-0.670706566238076,
-1.87868419754713));
#29879=CARTESIAN_POINT('Ctrl Pts',(-6.61892860029366,1.21298062366854,-1.58366019673188));
#29880=CARTESIAN_POINT('Ctrl Pts',(-6.50790710321483,1.98854156053368,0.158126766040605));
#29881=CARTESIAN_POINT('Ctrl Pts',(-6.396885606136,0.947457560543175,1.75545600431277));
#29882=CARTESIAN_POINT('Ctrl Pts',(-6.28586410905718,-0.95918238980143,
1.74907711528194));
#29883=CARTESIAN_POINT('Ctrl Pts',(-6.17484261197835,-1.98955509658577,
0.144817574063867));
#29884=CARTESIAN_POINT('Ctrl Pts',(-6.06382111489954,-1.20235694413303,
-1.59174099369315));
#29885=CARTESIAN_POINT('Ctrl Pts',(-5.9527996178207,0.683262130569029,-1.87415433543731));
#29886=CARTESIAN_POINT('Ctrl Pts',(-5.84177812074188,1.9446826897971,-0.444421925777357));
#29887=CARTESIAN_POINT('Ctrl Pts',(-5.73075662366305,1.4295258657179,1.39131499357682));
#29888=CARTESIAN_POINT('Ctrl Pts',(-5.61973512658423,-0.391583510524026,
1.95600714886062));
#29889=CARTESIAN_POINT('Ctrl Pts',(-5.50871362950539,-1.85495925128755,
0.73377638839835));
#29890=CARTESIAN_POINT('Ctrl Pts',(-5.39769213242658,-1.62372503327269,
-1.15880051278543));
#29891=CARTESIAN_POINT('Ctrl Pts',(-5.28667063534774,0.09087363589748,-1.99274774981856));
#29892=CARTESIAN_POINT('Ctrl Pts',(-5.17564913826893,1.72245411031465,-1.00620745871233));
#29893=CARTESIAN_POINT('Ctrl Pts',(-5.0646276411901,1.78047555002424,0.899560130215906));
#29894=CARTESIAN_POINT('Ctrl Pts',(-4.95360614411127,0.211932095470946,
1.98352877443648));
#29895=CARTESIAN_POINT('Ctrl Pts',(-4.84258464703245,-1.55022328846599,
1.25543194479265));
#29896=CARTESIAN_POINT('Ctrl Pts',(-4.73156314995362,-1.89616221312428,
-0.619572815436396));
#29897=CARTESIAN_POINT('Ctrl Pts',(-4.6205416528748,-0.509849948119368,
-1.92856284380646));
#29898=CARTESIAN_POINT('Ctrl Pts',(-4.50952015579597,1.3422390173527,-1.4757018778887));
#29899=CARTESIAN_POINT('Ctrl Pts',(-4.39849865871714,1.96811689258761,0.325296033205782));
#29900=CARTESIAN_POINT('Ctrl Pts',(-4.28747716163832,0.796008917780889,
1.82911766021806));
#29901=CARTESIAN_POINT('Ctrl Pts',(-4.17645566455949,-1.10329812536747,
1.66193708023761));
#29902=CARTESIAN_POINT('Ctrl Pts',(-4.06543416748067,-1.9946800674918,-0.0235168122582161));
#29903=CARTESIAN_POINT('Ctrl Pts',(-3.95441267040184,-1.06380920023413,
-1.68748676960926));
#29904=CARTESIAN_POINT('Ctrl Pts',(-3.84339117332301,0.838911406421511,
-1.80984233133253));
#29905=CARTESIAN_POINT('Ctrl Pts',(-3.73236967624419,1.97523910020347,-0.27880478678481));
#29906=CARTESIAN_POINT('Ctrl Pts',(-3.62134817916536,1.30707440535381,1.50693666455608));
#29907=CARTESIAN_POINT('Ctrl Pts',(-3.51032668208654,-0.555176522196224,
1.91600643039178));
#29908=CARTESIAN_POINT('Ctrl Pts',(-3.39930518500771,-1.91024236589515,
0.574696194211018));
#29909=CARTESIAN_POINT('Ctrl Pts',(-3.28828368792889,-1.52019400578695,
-1.29163144778971));
#29910=CARTESIAN_POINT('Ctrl Pts',(-3.17726219085006,0.258637369222239,
-1.97798087030399));
#29911=CARTESIAN_POINT('Ctrl Pts',(-3.06624069377124,1.80118891147076,-0.857333142529141));
#29912=CARTESIAN_POINT('Ctrl Pts',(-2.95521919669241,1.69825273491544,1.04653679377876));
#29913=CARTESIAN_POINT('Ctrl Pts',(-2.84419769961359,0.0438668457115283,
1.9943363085196));
#29914=CARTESIAN_POINT('Ctrl Pts',(-2.73317620253476,-1.65059388234868,
1.1201970575122));
#29915=CARTESIAN_POINT('Ctrl Pts',(-2.62215470545594,-1.83714394984282,
-0.777305423493693));
#29916=CARTESIAN_POINT('Ctrl Pts',(-2.51113320837711,-0.345359340796222,
-1.9646955322052));
#29917=CARTESIAN_POINT('Ctrl Pts',(-2.40011171129828,1.46193051412666,-1.35722539951385));
#29918=CARTESIAN_POINT('Ctrl Pts',(-2.28909021421946,1.9336643455383,0.490146734681156));
#29919=CARTESIAN_POINT('Ctrl Pts',(-2.17806871714063,0.638886665897876,
1.88974215549818));
#29920=CARTESIAN_POINT('Ctrl Pts',(-2.06704722006181,-1.23955002456831,
1.56295149123835));
#29921=CARTESIAN_POINT('Ctrl Pts',(-1.95602572298298,-1.98558784033205,
-0.191683601205323));
#29922=CARTESIAN_POINT('Ctrl Pts',(-1.84500422590415,-0.917679060845975,
-1.77120483535984));
#29923=CARTESIAN_POINT('Ctrl Pts',(-1.73398272882533,0.988581236720258,
-1.73263063163378));
#29924=CARTESIAN_POINT('Ctrl Pts',(-1.6229612317465,1.99171696059823,-0.111200309075107));
#29925=CARTESIAN_POINT('Ctrl Pts',(-1.51193973466768,1.17530650621655,1.61181728104857));
#29926=CARTESIAN_POINT('Ctrl Pts',(-1.40091823758885,-0.714812132693357,
1.86234975670057));
#29927=CARTESIAN_POINT('Ctrl Pts',(-1.28989674051002,-1.95191075933523,
0.411518854108752));
#29928=CARTESIAN_POINT('Ctrl Pts',(-1.1788752434312,-1.40582644920036,-1.41525436592699));
#29929=CARTESIAN_POINT('Ctrl Pts',(-1.06785374635237,0.42455527370623,-1.94911928584864));
#29930=CARTESIAN_POINT('Ctrl Pts',(-0.956832249273549,1.86709013999691,
-0.702341501252534));
#29931=CARTESIAN_POINT('Ctrl Pts',(-0.845810752194721,1.60391691372304,
1.18604158533899));
#29932=CARTESIAN_POINT('Ctrl Pts',(-0.734789255115897,-0.124494701954168,
1.99095308542736));
#29933=CARTESIAN_POINT('Ctrl Pts',(-0.623767758037071,-1.73923090825272,
0.976932208112631));
#29934=CARTESIAN_POINT('Ctrl Pts',(-0.512746260958245,-1.76497204256062,
-0.929410788251921));
#29935=CARTESIAN_POINT('Ctrl Pts',(-0.40172476387942,-0.178520008928735,
-1.98699022780528));
#29936=CARTESIAN_POINT('Ctrl Pts',(-0.290703266800595,1.57141698961275,
-1.22876000916521));
#29937=CARTESIAN_POINT('Ctrl Pts',(-0.179681769721768,1.88501844830769,
0.650902089763596));
#29938=CARTESIAN_POINT('Ctrl Pts',(-0.0686602726429429,0.478009206908001,
1.93805924459805));
#29939=CARTESIAN_POINT('Ctrl Pts',(0.0423612244358815,-1.36862551735633,
1.45047221915076));
#29940=CARTESIAN_POINT('Ctrl Pts',(0.116375555821768,-1.76163155377538,
0.248286520766087));
#29941=CARTESIAN_POINT('Ctrl Pts',(0.15338272151471,-1.66084738178985,-0.303406359271283));
#29942=CARTESIAN_POINT('Ctrl Pts',(-15.646,0.903606778650232,-1.26612599672282));
#29943=CARTESIAN_POINT('Ctrl Pts',(-15.6089928343071,1.32418286847098,-0.965969924828001));
#29944=CARTESIAN_POINT('Ctrl Pts',(-15.5349785029212,1.83555016250808,0.0811162878112121));
#29945=CARTESIAN_POINT('Ctrl Pts',(-15.4239570058423,0.927248239037281,
1.58822321403664));
#29946=CARTESIAN_POINT('Ctrl Pts',(-15.3129355087635,-0.828910895913401,
1.63972535647931));
#29947=CARTESIAN_POINT('Ctrl Pts',(-15.2019140116847,-1.82741159222543,
0.195591560127152));
#29948=CARTESIAN_POINT('Ctrl Pts',(-15.0908925146059,-1.15667974077379,
-1.42844591152668));
#29949=CARTESIAN_POINT('Ctrl Pts',(-14.979871017527,0.570855243925188,-1.74687800671557));
#29950=CARTESIAN_POINT('Ctrl Pts',(-14.8688495204482,1.77682346771718,-0.469774267555894));
#29951=CARTESIAN_POINT('Ctrl Pts',(-14.7578280233694,1.3595938034014,1.2366712040288));
#29952=CARTESIAN_POINT('Ctrl Pts',(-14.6468065262906,-0.299717618166574,
1.81325504017035));
#29953=CARTESIAN_POINT('Ctrl Pts',(-14.5357850292117,-1.68521162662156,
0.733376776298527));
#29954=CARTESIAN_POINT('Ctrl Pts',(-14.4247635321329,-1.53117415339972,
-1.01650815349415));
#29955=CARTESIAN_POINT('Ctrl Pts',(-14.3137420350541,0.0216796534424384,
-1.83774207162163));
#29956=CARTESIAN_POINT('Ctrl Pts',(-14.2027205379753,1.55472664688603,-0.980101962297276));
#29957=CARTESIAN_POINT('Ctrl Pts',(-14.0916990408964,1.66744375345186,0.772920313447068));
#29958=CARTESIAN_POINT('Ctrl Pts',(-13.9806775438176,0.256856552130983,
1.81983431302347));
#29959=CARTESIAN_POINT('Ctrl Pts',(-13.8696560467388,-1.38838342706959,
1.20422799223356));
#29960=CARTESIAN_POINT('Ctrl Pts',(-13.75863454966,-1.76525688713531,-0.511509097450093));
#29961=CARTESIAN_POINT('Ctrl Pts',(-13.6476130525811,-0.529468511212632,
-1.75995347711011));
#29962=CARTESIAN_POINT('Ctrl Pts',(-13.5365915555023,1.19001920390447,-1.40058118296215));
#29963=CARTESIAN_POINT('Ctrl Pts',(-13.4255700584235,1.82235723230149,0.238301140323824));
#29964=CARTESIAN_POINT('Ctrl Pts',(-13.3145485613446,0.789869078999073,
1.65948188258691));
#29965=CARTESIAN_POINT('Ctrl Pts',(-13.2035270642659,-0.964209049677692,
1.56463229551752));
#29966=CARTESIAN_POINT('Ctrl Pts',(-13.092505567187,-1.83742779929035,0.0404027967352005));
#29967=CARTESIAN_POINT('Ctrl Pts',(-12.9814840701082,-1.03205255985982,
-1.52073693099926));
#29968=CARTESIAN_POINT('Ctrl Pts',(-12.8704625730293,0.716160935289581,
-1.69259765416285));
#29969=CARTESIAN_POINT('Ctrl Pts',(-12.7594410759505,1.81012100052783,-0.318174898587703));
#29970=CARTESIAN_POINT('Ctrl Pts',(-12.6484195788717,1.25043337930754,1.3469185818581));
#29971=CARTESIAN_POINT('Ctrl Pts',(-12.5373980817929,-0.451595700759593,
1.78152592625865));
#29972=CARTESIAN_POINT('Ctrl Pts',(-12.426376584714,-1.74106662288298,0.588608798190727));
#29973=CARTESIAN_POINT('Ctrl Pts',(-12.3153550876353,-1.43997492966776,
-1.14203568443429));
#29974=CARTESIAN_POINT('Ctrl Pts',(-12.2043335905564,0.176615125299183,
-1.82936611977922));
#29975=CARTESIAN_POINT('Ctrl Pts',(-12.0933120934776,1.63185729621746,-0.845467366266227));
#29976=CARTESIAN_POINT('Ctrl Pts',(-11.9822905963988,1.59630573484127,0.910813539398446));
#29977=CARTESIAN_POINT('Ctrl Pts',(-11.8712690993199,0.10243879880857,1.83501487600212));
#29978=CARTESIAN_POINT('Ctrl Pts',(-11.7602476022411,-1.48501176096542,
1.08282656618605));
#29979=CARTESIAN_POINT('Ctrl Pts',(-11.6492261051623,-1.7158202719779,-0.658584920047561));
#29980=CARTESIAN_POINT('Ctrl Pts',(-11.5382046080835,-0.379130133977537,
-1.79834191525306));
#29981=CARTESIAN_POINT('Ctrl Pts',(-11.4271831110046,1.30391677723258,-1.2952120832884));
#29982=CARTESIAN_POINT('Ctrl Pts',(-11.3161616139258,1.79576212723163,0.391167080728389));
#29983=CARTESIAN_POINT('Ctrl Pts',(-11.205140116847,0.647077432006542,1.72019304138606));
#29984=CARTESIAN_POINT('Ctrl Pts',(-11.0941186197681,-1.09274901450927,
1.47772558140343));
#29985=CARTESIAN_POINT('Ctrl Pts',(-10.9830971226893,-1.83428756809842,
-0.114727591122236));
#29986=CARTESIAN_POINT('Ctrl Pts',(-10.8720756256105,-0.900100912087758,
-1.60237063462356));
#29987=CARTESIAN_POINT('Ctrl Pts',(-10.7610541285317,0.85637872338898,-1.62615767524916));
#29988=CARTESIAN_POINT('Ctrl Pts',(-10.6500326314529,1.83050806619295,-0.164357908990289));
#29989=CARTESIAN_POINT('Ctrl Pts',(-10.539011134374,1.13236498768008,1.44759208250163));
#29990=CARTESIAN_POINT('Ctrl Pts',(-10.4279896372952,-0.600257410937894,
1.73708501325043));
#29991=CARTESIAN_POINT('Ctrl Pts',(-10.3169681402164,-1.78451078975135,
0.439652753779773));
#29992=CARTESIAN_POINT('Ctrl Pts',(-10.2059466431376,-1.33851285508659,
-1.25942710762198));
#29993=CARTESIAN_POINT('Ctrl Pts',(-10.0949251460587,0.330292110303061,
-1.80794923173099));
#29994=CARTESIAN_POINT('Ctrl Pts',(-9.98390364897991,1.69735659323361,-0.704807702888898));
#29995=CARTESIAN_POINT('Ctrl Pts',(-9.87288215190106,1.51379003966279,1.04221543764369));
#29996=CARTESIAN_POINT('Ctrl Pts',(-9.76186065482225,-0.0527091443318308,
1.83711595952703));
#29997=CARTESIAN_POINT('Ctrl Pts',(-9.65083915774341,-1.5710555503927,0.953707376623146));
#29998=CARTESIAN_POINT('Ctrl Pts',(-9.53981766066459,-1.6541540502575,-0.800966716325862));
#29999=CARTESIAN_POINT('Ctrl Pts',(-9.42879616358577,-0.226089474720918,
-1.82391251217418));
#30000=CARTESIAN_POINT('Ctrl Pts',(-9.31777466650694,1.40852059510137,-1.18061129751514));
#30001=CARTESIAN_POINT('Ctrl Pts',(-9.20675316942812,1.75636761288009,0.541244964014445));
#30002=CARTESIAN_POINT('Ctrl Pts',(-9.09573167234929,0.499673697483888,
1.76864340631115));
#30003=CARTESIAN_POINT('Ctrl Pts',(-8.98471017527046,-1.21350033913767,
1.38028628536181));
#30004=CARTESIAN_POINT('Ctrl Pts',(-8.87368867819165,-1.81807333330707,
-0.269040252309636));
#30005=CARTESIAN_POINT('Ctrl Pts',(-8.7626671811128,-0.761733736392313,
-1.67258333648488));
#30006=CARTESIAN_POINT('Ctrl Pts',(-8.651645684034,0.990492616380764,-1.54812715225214));
#30007=CARTESIAN_POINT('Ctrl Pts',(-8.54062418695516,1.83784806665277,-0.00936944746539623));
#30008=CARTESIAN_POINT('Ctrl Pts',(-8.42960268987634,1.00622559096247,1.53794777633616));
#30009=CARTESIAN_POINT('Ctrl Pts',(-8.31858119279751,-0.744640747383609,
1.68026291394564));
#30010=CARTESIAN_POINT('Ctrl Pts',(-8.20755969571868,-1.81523573995617,
0.287563055747619));
#30011=CARTESIAN_POINT('Ctrl Pts',(-8.09653819863986,-1.22751044310728,
-1.36784188220264));
#30012=CARTESIAN_POINT('Ctrl Pts',(-7.98551670156104,0.481614916815858,
-1.77364606800387));
#30013=CARTESIAN_POINT('Ctrl Pts',(-7.87449520448221,1.75075787078272,-0.559124476782657));
#30014=CARTESIAN_POINT('Ctrl Pts',(-7.76347370740338,1.42048470756065,1.16618887759722));
#30015=CARTESIAN_POINT('Ctrl Pts',(-7.65245221032457,-0.207481399618984,
1.82612287961606));
#30016=CARTESIAN_POINT('Ctrl Pts',(-7.54143071324572,-1.6459015392462,0.817790575729572));
#30017=CARTESIAN_POINT('Ctrl Pts',(-7.43040921616691,-1.58069773800288,
-0.937639570260189));
#30018=CARTESIAN_POINT('Ctrl Pts',(-7.31938771908807,-0.0714373480345857,
-1.8364830540876));
#30019=CARTESIAN_POINT('Ctrl Pts',(-7.20836622200926,1.50308509085693,-1.05759562796407));
#30020=CARTESIAN_POINT('Ctrl Pts',(-7.09734472493043,1.70445447418163,0.687465088631667));
#30021=CARTESIAN_POINT('Ctrl Pts',(-6.9863232278516,0.348708506197304,1.80448765037358));
#30022=CARTESIAN_POINT('Ctrl Pts',(-6.87530173077278,-1.32560236120598,
1.27300890908518));
#30023=CARTESIAN_POINT('Ctrl Pts',(-6.76428023369395,-1.78890066263481,
-0.421435311607665));
#30024=CARTESIAN_POINT('Ctrl Pts',(-6.65325873661513,-0.617937253968403,
-1.73087459187634));
#30025=CARTESIAN_POINT('Ctrl Pts',(-6.5422372395363,1.11754670885474,-1.45906225232958));
#30026=CARTESIAN_POINT('Ctrl Pts',(-6.43121574245748,1.83208868553414,0.145685795405434));
#30027=CARTESIAN_POINT('Ctrl Pts',(-6.32019424537864,0.872914255927876,
1.6173416474088));
#30028=CARTESIAN_POINT('Ctrl Pts',(-6.20917274829983,-0.883716608491293,
1.61146463148335));
#30029=CARTESIAN_POINT('Ctrl Pts',(-6.09815125122099,-1.83302247941115,
0.133423733340373));
#30030=CARTESIAN_POINT('Ctrl Pts',(-5.98712975414218,-1.10775887064102,
-1.46650727484089));
#30031=CARTESIAN_POINT('Ctrl Pts',(-5.87610825706334,0.629504981698008,
-1.72670112661761));
#30032=CARTESIAN_POINT('Ctrl Pts',(-5.76508675998453,1.79168050778642,-0.409456054617966));
#30033=CARTESIAN_POINT('Ctrl Pts',(-5.65406526290569,1.31705477835589,1.28185023050864));
#30034=CARTESIAN_POINT('Ctrl Pts',(-5.54304376582688,-0.360774817741443,
1.80211399015954));
#30035=CARTESIAN_POINT('Ctrl Pts',(-5.43202226874804,-1.7090162578743,0.676044919340745));
#30036=CARTESIAN_POINT('Ctrl Pts',(-5.32100077166922,-1.49597489985528,
-1.06762933719906));
#30037=CARTESIAN_POINT('Ctrl Pts',(-5.20997927459039,0.0837239529942017,
-1.83596394363836));
#30038=CARTESIAN_POINT('Ctrl Pts',(-5.09895777751157,1.58693624990787,-0.927041876817589));
#30039=CARTESIAN_POINT('Ctrl Pts',(-4.98793628043274,1.64039272540732,0.828785261135749));
#30040=CARTESIAN_POINT('Ctrl Pts',(-4.87691478335392,0.195257872362318,
1.82747029139345));
#30041=CARTESIAN_POINT('Ctrl Pts',(-4.76589328627509,-1.42825606626389,
1.15665807904736));
#30042=CARTESIAN_POINT('Ctrl Pts',(-4.65487178919627,-1.74697748618844,
-0.57082656332359));
#30043=CARTESIAN_POINT('Ctrl Pts',(-4.54385029211744,-0.469736383593091,
-1.77682892608546));
#30044=CARTESIAN_POINT('Ctrl Pts',(-4.43282879503861,1.2366354145067,-1.35959779134602));
#30045=CARTESIAN_POINT('Ctrl Pts',(-4.32180729795979,1.8132709732004,0.299702653298089));
#30046=CARTESIAN_POINT('Ctrl Pts',(-4.21078580088097,0.733381167783709,
1.68520781074188));
#30047=CARTESIAN_POINT('Ctrl Pts',(-4.09976430380214,-1.01649372201922,
1.53118053009453));
#30048=CARTESIAN_POINT('Ctrl Pts',(-3.98874280672331,-1.83774423197443,
-0.0216665754003948));
#30049=CARTESIAN_POINT('Ctrl Pts',(-3.87772130964449,-0.980111674806025,
-1.55472004153636));
#30050=CARTESIAN_POINT('Ctrl Pts',(-3.76669981256566,0.772908208897534,
-1.66744901069363));
#30051=CARTESIAN_POINT('Ctrl Pts',(-3.65567831548684,1.81983282548855,-0.256869207804794));
#30052=CARTESIAN_POINT('Ctrl Pts',(-3.54465681840801,1.20423745559398,1.38837511256683));
#30053=CARTESIAN_POINT('Ctrl Pts',(-3.43363532132918,-0.511496789897079,
1.76526041607566));
#30054=CARTESIAN_POINT('Ctrl Pts',(-3.32261382425036,-1.75994985201377,
0.529480708842188));
#30055=CARTESIAN_POINT('Ctrl Pts',(-3.21159232717153,-1.40058940335731,
-1.19000950663588));
#30056=CARTESIAN_POINT('Ctrl Pts',(-3.1005708300927,0.238288506115619,-1.82235888080426));
#30057=CARTESIAN_POINT('Ctrl Pts',(-2.98954933301389,1.65947641764626,-0.789880574454531));
#30058=CARTESIAN_POINT('Ctrl Pts',(-2.87852783593505,1.5646389708752,0.964198212866461));
#30059=CARTESIAN_POINT('Ctrl Pts',(-2.76750633885623,0.0404155252740006,
1.83742751899441));
#30060=CARTESIAN_POINT('Ctrl Pts',(-2.6564848417774,-1.52072978321424,1.03206309355985));
#30061=CARTESIAN_POINT('Ctrl Pts',(-2.54546334469858,-1.69260261440109,
-0.716149211990789));
#30062=CARTESIAN_POINT('Ctrl Pts',(-2.43444184761975,-0.31818743609586,
-1.81011879586092));
#30063=CARTESIAN_POINT('Ctrl Pts',(-2.32342035054093,1.34690991987603,-1.25044271013452));
#30064=CARTESIAN_POINT('Ctrl Pts',(-2.2123988534621,1.78152905596337,0.45158336374919));
#30065=CARTESIAN_POINT('Ctrl Pts',(-2.10137735638328,0.588620854178164,
1.74106254069739));
#30066=CARTESIAN_POINT('Ctrl Pts',(-1.99035585930445,-1.14202570378047,
1.43998284972631));
#30067=CARTESIAN_POINT('Ctrl Pts',(-1.87933436222563,-1.82936735575706,
-0.176602472857783));
#30068=CARTESIAN_POINT('Ctrl Pts',(-1.7683128651468,-0.845478645101226,
-1.63185140458178));
#30069=CARTESIAN_POINT('Ctrl Pts',(-1.65729136806797,0.910802436555798,
-1.59631211106002));
#30070=CARTESIAN_POINT('Ctrl Pts',(-1.54626987098914,1.83501425402401,-0.102451380513119));
#30071=CARTESIAN_POINT('Ctrl Pts',(-1.43524837391032,1.08283668534245,1.48500401619214));
#30072=CARTESIAN_POINT('Ctrl Pts',(-1.32422687683149,-0.658572718107321,
1.71582529904111));
#30073=CARTESIAN_POINT('Ctrl Pts',(-1.21320537975267,-1.79833989307757,
0.379141704382714));
#30074=CARTESIAN_POINT('Ctrl Pts',(-1.10218388267384,-1.29521996548735,
-1.30390612015762));
#30075=CARTESIAN_POINT('Ctrl Pts',(-0.991162385595018,0.391152455034581,
-1.79576804489885));
#30076=CARTESIAN_POINT('Ctrl Pts',(-0.880140888516193,1.72019272226962,
-0.647083240986163));
#30077=CARTESIAN_POINT('Ctrl Pts',(-0.769119391437366,1.47772522761866,
1.09272715853592));
#30078=CARTESIAN_POINT('Ctrl Pts',(-0.658097894358541,-0.114699807832016,
1.83431047841002));
#30079=CARTESIAN_POINT('Ctrl Pts',(-0.547076397279716,-1.60239309641882,
0.900069920860329));
#30080=CARTESIAN_POINT('Ctrl Pts',(-0.43605490020089,-1.62610899044603,
-0.856287353085414));
#30081=CARTESIAN_POINT('Ctrl Pts',(-0.325033403122065,-0.164474555116665,
-1.83065940731556));
#30082=CARTESIAN_POINT('Ctrl Pts',(-0.21401190604324,1.4477823064221,-1.13208461653888));
#30083=CARTESIAN_POINT('Ctrl Pts',(-0.102990408964413,1.73671048154547,
0.599690938180032));
#30084=CARTESIAN_POINT('Ctrl Pts',(0.00803108811441221,0.440400782633002,
1.78557817668643));
#30085=CARTESIAN_POINT('Ctrl Pts',(0.119052585193236,-1.26094589866601,
1.33635313142488));
#30086=CARTESIAN_POINT('Ctrl Pts',(0.193066916579123,-1.62303132195317,
0.228752033396824));
#30087=CARTESIAN_POINT('Ctrl Pts',(0.230074082272065,-1.53017656606561,
-0.279535197539876));
#30088=CARTESIAN_POINT('',(0.,-1.92218901323832,-0.351148682734097));
#30089=CARTESIAN_POINT('Ctrl Pts',(1.0547118733939E-15,0.480182858679996,
1.4822056829043));
#30090=CARTESIAN_POINT('Ctrl Pts',(1.40003008271787E-15,0.446073771342386,
1.49837437681773));
#30091=CARTESIAN_POINT('Ctrl Pts',(3.73246695668943E-15,0.411402367961804,
1.5131874054692));
#30092=CARTESIAN_POINT('Ctrl Pts',(2.692290834716E-15,0.376229275515442,
1.52659018558423));
#30093=CARTESIAN_POINT('Ctrl Pts',(1.05407315971151E-15,0.320788673731233,
1.54771594233397));
#30094=CARTESIAN_POINT('Ctrl Pts',(-4.67470066845617E-15,0.264103101937485,
1.56534066809337));
#30095=CARTESIAN_POINT('Ctrl Pts',(-7.49400541621981E-15,0.206476417853331,
1.57959203319563));
#30096=CARTESIAN_POINT('Ctrl Pts',(-9.15600442216292E-15,0.172505102145218,
1.58799330824477));
#30097=CARTESIAN_POINT('Ctrl Pts',(-4.65850075858084E-15,0.138206098176861,
1.59522147264912));
#30098=CARTESIAN_POINT('Ctrl Pts',(-4.46864767411626E-15,0.1036374144592,
1.60129566587682));
#30099=CARTESIAN_POINT('Ctrl Pts',(-4.38277324586137E-15,0.0880012926750868,
1.60404314755197));
#30100=CARTESIAN_POINT('Ctrl Pts',(-1.04319479122915E-14,0.0723076512843924,
1.60655463309822));
#30101=CARTESIAN_POINT('Ctrl Pts',(-9.96425164601078E-15,0.0565846426208889,
1.60882871578729));
#30102=CARTESIAN_POINT('Ctrl Pts',(-8.12965378682446E-15,-0.00509085088565643,
1.61774909324972));
#30103=CARTESIAN_POINT('Ctrl Pts',(-4.56836786455393E-15,-0.0672895814378321,
1.62303444302115));
#30104=CARTESIAN_POINT('Ctrl Pts',(-3.94129173741931E-15,-0.129678743792337,
1.62482203126307));
#30105=CARTESIAN_POINT('Ctrl Pts',(-3.45837203070848E-15,-0.177725471585729,
1.62619867686024));
#30106=CARTESIAN_POINT('Ctrl Pts',(-8.22270713878231E-15,-0.225885969277299,
1.62549994364171));
#30107=CARTESIAN_POINT('Ctrl Pts',(-9.35362898246694E-15,-0.274016954341825,
1.62276943393303));
#30108=CARTESIAN_POINT('Ctrl Pts',(-9.74287591606784E-15,-0.290582942922006,
1.62182963200312));
#30109=CARTESIAN_POINT('Ctrl Pts',(-5.84326107154292E-15,-0.307145480266589,
1.62064899356115));
#30110=CARTESIAN_POINT('Ctrl Pts',(-5.77315972805081E-15,-0.32369883547967,
1.61922884021275));
#30111=CARTESIAN_POINT('Ctrl Pts',(-5.70623215198899E-15,-0.339502754276557,
1.61787298287094));
#30112=CARTESIAN_POINT('Ctrl Pts',(-7.88705881085276E-15,-0.355302127669727,
1.61629822797713));
#30113=CARTESIAN_POINT('Ctrl Pts',(-7.85482789922298E-15,-0.37106496199202,
1.6145090262086));
#30114=CARTESIAN_POINT('Ctrl Pts',(-7.72335550546971E-15,-0.435362788392118,
1.60721073312527));
#30115=CARTESIAN_POINT('Ctrl Pts',(-3.55546619181194E-15,-0.499135001074743,
1.59634267751575));
#30116=CARTESIAN_POINT('Ctrl Pts',(-3.41393580072236E-15,-0.562042543794224,
1.58204256350879));
#30117=CARTESIAN_POINT('Ctrl Pts',(-3.26945119203353E-15,-0.626263179541966,
1.56744395779171));
#30118=CARTESIAN_POINT('Ctrl Pts',(-5.59097293134417E-15,-0.689583748551309,
1.54926866320265));
#30119=CARTESIAN_POINT('Ctrl Pts',(-6.02295990859147E-15,-0.751656795048653,
1.52761115641076));
#30120=CARTESIAN_POINT('Ctrl Pts',(-6.30853923919458E-15,-0.792692242876652,
1.5132937426508));
#30121=CARTESIAN_POINT('Ctrl Pts',(-8.12105679605289E-15,-0.833182736037355,
1.49745341724689));
#30122=CARTESIAN_POINT('Ctrl Pts',(-8.77076189453874E-15,-0.873027345587097,
1.48010498047163));
#30123=CARTESIAN_POINT('Ctrl Pts',(-9.08990039389072E-15,-0.892599223549276,
1.471583338743));
#30124=CARTESIAN_POINT('Ctrl Pts',(-4.31109323122687E-15,-0.912015235103237,
1.46269766499479));
#30125=CARTESIAN_POINT('Ctrl Pts',(-4.44089209850063E-15,-0.931263178081411,
1.45344884058705));
#30126=CARTESIAN_POINT('Ctrl Pts',(-4.52342416443145E-15,-0.943501901979956,
1.44756801433768));
#30127=CARTESIAN_POINT('Ctrl Pts',(-6.71139558524068E-15,-0.955672671980721,
1.4415403547937));
#30128=CARTESIAN_POINT('Ctrl Pts',(-6.9111383282916E-15,-0.967772301054401,
1.43536596810798));
#30129=CARTESIAN_POINT('Ctrl Pts',(-7.06505675977478E-15,-0.977096073723701,
1.4306080885499));
#30130=CARTESIAN_POINT('Ctrl Pts',(-7.66117988453509E-15,-0.986374557138314,
1.42576457472066));
#30131=CARTESIAN_POINT('Ctrl Pts',(-7.38298311375729E-15,-0.995598865169279,
1.42083978831382));
#30132=CARTESIAN_POINT('Ctrl Pts',(-5.5803017413817E-15,-1.05537126372727,
1.38892776901282));
#30133=CARTESIAN_POINT('Ctrl Pts',(3.49033535941956E-16,-1.11296260466219,
1.35355987724473));
#30134=CARTESIAN_POINT('Ctrl Pts',(-5.55111512312578E-17,-1.16801443157665,
1.31484833578652));
#30135=CARTESIAN_POINT('Ctrl Pts',(-1.58292162970789E-16,-1.18200122376002,
1.30501305300262));
#30136=CARTESIAN_POINT('Ctrl Pts',(-8.42000433806714E-15,-1.19582408399153,
1.29496167698215));
#30137=CARTESIAN_POINT('Ctrl Pts',(-8.2572837456496E-15,-1.20947707828799,
1.28469551483091));
#30138=CARTESIAN_POINT('Ctrl Pts',(-7.63946596890415E-15,-1.2613147864529,
1.24571693577246));
#30139=CARTESIAN_POINT('Ctrl Pts',(-3.87298011944514E-15,-1.31070559621982,
1.20364581809758));
#30140=CARTESIAN_POINT('Ctrl Pts',(-3.05311331771918E-15,-1.35758932481216,
1.15879636045725));
#30141=CARTESIAN_POINT('Ctrl Pts',(-2.60837798406203E-15,-1.38302132258876,
1.13446784945275));
#30142=CARTESIAN_POINT('Ctrl Pts',(-3.43302993469709E-15,-1.40771522401955,
1.10932096817457));
#30143=CARTESIAN_POINT('Ctrl Pts',(-3.6498581934552E-15,-1.43165822803284,
1.08340051001308));
#30144=CARTESIAN_POINT('Ctrl Pts',(-3.8156193117322E-15,-1.44996220345968,
1.06358480814972));
#30145=CARTESIAN_POINT('Ctrl Pts',(-2.87284372802704E-15,-1.46782728641225,
1.04331692584045));
#30146=CARTESIAN_POINT('Ctrl Pts',(-3.1641356201817E-15,-1.48524671954972,
1.02261561267638));
#30147=CARTESIAN_POINT('Ctrl Pts',(-3.32383551962965E-15,-1.49479687111733,
1.01126618030362));
#30148=CARTESIAN_POINT('Ctrl Pts',(-6.89733966939696E-15,-1.50421538093661,
0.999783335138857));
#30149=CARTESIAN_POINT('Ctrl Pts',(-6.74460487459783E-15,-1.51348427825112,
0.988191590561737));
#30150=CARTESIAN_POINT('Ctrl Pts',(-6.04666371398387E-15,-1.55583968886863,
0.935221632574525));
#30151=CARTESIAN_POINT('Ctrl Pts',(-3.0413638622061E-15,-1.59514251466625,
0.879902068251074));
#30152=CARTESIAN_POINT('Ctrl Pts',(-2.94209101525666E-15,-1.6313405550829,
0.822591921935408));
#30153=CARTESIAN_POINT('Ctrl Pts',(-2.84072911148816E-15,-1.66830033212234,
0.764075764553859));
#30154=CARTESIAN_POINT('Ctrl Pts',(-2.77218863047414E-15,-1.70202388244217,
0.703483705813104));
#30155=CARTESIAN_POINT('Ctrl Pts',(-2.85188539450587E-15,-1.73242530624915,
0.641151720491997));
#30156=CARTESIAN_POINT('Ctrl Pts',(-2.93218559451239E-15,-1.76305691898579,
0.578347779216597));
#30157=CARTESIAN_POINT('Ctrl Pts',(-2.99436507783698E-15,-1.79031650407563,
0.513776618683869));
#30158=CARTESIAN_POINT('Ctrl Pts',(-3.77475828372553E-15,-1.81407668145728,
0.447747080004075));
#30159=CARTESIAN_POINT('Ctrl Pts',(-3.97176467194236E-15,-1.8200748202084,
0.431078250966644));
#30160=CARTESIAN_POINT('Ctrl Pts',(-5.93455269918665E-15,-1.82584972626931,
0.414316345880479));
#30161=CARTESIAN_POINT('Ctrl Pts',(-6.07153216591882E-15,-1.83139888490863,
0.397466087487765));
#30162=CARTESIAN_POINT('Ctrl Pts',(-6.17145811240212E-15,-1.8354469728626,
0.385173894660996));
#30163=CARTESIAN_POINT('Ctrl Pts',(-3.09749045409741E-15,-1.83937529592778,
0.37283314186271));
#30164=CARTESIAN_POINT('Ctrl Pts',(-2.82412981889024E-15,-1.84317748112416,
0.360463942797997));
#30165=CARTESIAN_POINT('Ctrl Pts',(-1.2991746729061E-15,-1.86438814986878,
0.291461784710604));
#30166=CARTESIAN_POINT('Ctrl Pts',(1.37739593958821E-15,-1.88171855913059,
0.221453627220656));
#30167=CARTESIAN_POINT('Ctrl Pts',(1.30451205393456E-15,-1.89508700640948,
0.150800366152206));
#30168=CARTESIAN_POINT('Ctrl Pts',(1.23145509346081E-15,-1.90848719927364,
0.0799793272500314));
#30169=CARTESIAN_POINT('Ctrl Pts',(-1.27203037467893E-15,-1.91790714514985,
0.00850916986176715));
#30170=CARTESIAN_POINT('Ctrl Pts',(-2.42167397246362E-15,-1.92322202108538,
-0.0632768841144876));
#30171=CARTESIAN_POINT('Ctrl Pts',(-3.54683445949221E-15,-1.92842371003285,
-0.133534163509098));
#30172=CARTESIAN_POINT('Ctrl Pts',(-4.48891627368549E-15,-1.92969366211441,
-0.204094995398863));
#30173=CARTESIAN_POINT('Ctrl Pts',(-6.6040922730437E-15,-1.9268677763229,
-0.274661643730342));
#30174=CARTESIAN_POINT('Ctrl Pts',(-7.36841819229932E-15,-1.92584663304406,
-0.300161138037724));
#30175=CARTESIAN_POINT('Ctrl Pts',(3.63423914059134E-17,-1.92429019227826,
-0.325661462754304));
#30176=CARTESIAN_POINT('Ctrl Pts',(0.,-1.92218901323832,-0.351148682734097));
#30177=CARTESIAN_POINT('Ctrl Pts',(0.,-1.92218901323832,-0.351148682734097));
#30178=CARTESIAN_POINT('Ctrl Pts',(-0.00671010262525542,-1.94333860721344,
-0.235375737618954));
#30179=CARTESIAN_POINT('Ctrl Pts',(-0.0134202052505109,-1.9531764658261,
-0.117723130693868));
#30180=CARTESIAN_POINT('Ctrl Pts',(-0.0201303078757663,-1.95230810266922,
-4.45419903166711E-5));
#30181=CARTESIAN_POINT('Origin',(-7.7,0.,0.));
#30182=CARTESIAN_POINT('Origin',(0.,0.,0.));
#30183=CARTESIAN_POINT('Origin',(-16.,1.6,0.));
#30184=CARTESIAN_POINT('',(-16.,-1.6,-1.95943487863577E-16));
#30185=CARTESIAN_POINT('Origin',(-16.,0.,0.));
#30186=CARTESIAN_POINT('Origin',(-15.8,0.,0.));
#30187=CARTESIAN_POINT('',(-15.8,-1.8,-2.20436423846524E-16));
#30188=CARTESIAN_POINT('Origin',(2.51157561548264,0.,0.));
#30189=CARTESIAN_POINT('',(2.38930775492008,3.5,-2.02072594216369));
#30190=CARTESIAN_POINT('',(2.38930775492008,-7.42402667107435E-16,-4.04145188432738));
#30191=CARTESIAN_POINT('Ctrl Pts',(2.38930775492008,3.5,-2.02072594216369));
#30192=CARTESIAN_POINT('Ctrl Pts',(2.98258118464813,1.75,-3.03108891324554));
#30193=CARTESIAN_POINT('Ctrl Pts',(2.38930775492008,-7.42402667107435E-16,
-4.04145188432738));
#30194=CARTESIAN_POINT('',(2.38930775492008,3.5,2.02072594216369));
#30195=CARTESIAN_POINT('Ctrl Pts',(2.38930775492008,3.5,2.02072594216369));
#30196=CARTESIAN_POINT('Ctrl Pts',(2.98258118464813,3.5,-3.60822483003176E-15));
#30197=CARTESIAN_POINT('Ctrl Pts',(2.38930775492008,3.5,-2.02072594216369));
#30198=CARTESIAN_POINT('',(2.38930775492008,2.47467555702478E-16,4.04145188432738));
#30199=CARTESIAN_POINT('Ctrl Pts',(2.38930775492008,2.47467555702478E-16,
4.04145188432738));
#30200=CARTESIAN_POINT('Ctrl Pts',(2.98258118464813,1.75,3.03108891324553));
#30201=CARTESIAN_POINT('Ctrl Pts',(2.38930775492008,3.5,2.02072594216369));
#30202=CARTESIAN_POINT('',(2.38930775492008,-3.5,2.02072594216369));
#30203=CARTESIAN_POINT('Ctrl Pts',(2.38930775492008,-3.5,2.02072594216369));
#30204=CARTESIAN_POINT('Ctrl Pts',(2.98258118464813,-1.75,3.03108891324554));
#30205=CARTESIAN_POINT('Ctrl Pts',(2.38930775492008,2.47467555702478E-16,
4.04145188432738));
#30206=CARTESIAN_POINT('',(2.70724202769303,-3.5,-4.31113475248839E-16));
#30207=CARTESIAN_POINT('Ctrl Pts',(2.70724202769303,-3.5,-4.33600570796104E-16));
#30208=CARTESIAN_POINT('Ctrl Pts',(2.70724202769303,-3.5,0.937822173508931));
#30209=CARTESIAN_POINT('Ctrl Pts',(2.38930775492008,-3.5,2.02072594216369));
#30210=CARTESIAN_POINT('',(2.8,-3.34203030879952,-4.09280672032477E-16));
#30211=CARTESIAN_POINT('',(2.51157561548264,-3.83322594216369,-4.69434788047936E-16));
#30212=CARTESIAN_POINT('Origin',(2.8,0.,0.));
#30213=CARTESIAN_POINT('',(2.38930775492008,-3.5,-2.02072594216369));
#30214=CARTESIAN_POINT('Ctrl Pts',(2.38930775492008,-3.5,-2.02072594216369));
#30215=CARTESIAN_POINT('Ctrl Pts',(2.70724202769302,-3.5,-0.93782217350893));
#30216=CARTESIAN_POINT('Ctrl Pts',(2.70724202769303,-3.5,-4.33600570796104E-16));
#30217=CARTESIAN_POINT('Ctrl Pts',(2.38930775492008,-7.42402667107435E-16,
-4.04145188432738));
#30218=CARTESIAN_POINT('Ctrl Pts',(2.98258118464813,-1.75,-3.03108891324553));
#30219=CARTESIAN_POINT('Ctrl Pts',(2.38930775492008,-3.5,-2.02072594216369));
#30220=CARTESIAN_POINT('Origin',(0.,2.47467555702478E-16,4.04145188432738));
#30221=CARTESIAN_POINT('',(0.,2.47467555702478E-16,4.04145188432738));
#30222=CARTESIAN_POINT('',(0.,2.47467555702478E-16,4.04145188432738));
#30223=CARTESIAN_POINT('',(0.,-3.5,2.02072594216369));
#30224=CARTESIAN_POINT('',(0.,2.47467555702478E-16,4.04145188432738));
#30225=CARTESIAN_POINT('',(0.,-3.5,2.02072594216369));
#30226=CARTESIAN_POINT('Origin',(0.,3.5,2.02072594216369));
#30227=CARTESIAN_POINT('',(0.,3.5,2.02072594216369));
#30228=CARTESIAN_POINT('',(0.,3.5,2.02072594216369));
#30229=CARTESIAN_POINT('',(0.,3.5,2.02072594216369));
#30230=CARTESIAN_POINT('Origin',(0.,3.5,-2.02072594216369));
#30231=CARTESIAN_POINT('',(0.,3.5,-2.02072594216369));
#30232=CARTESIAN_POINT('',(0.,3.5,-2.02072594216369));
#30233=CARTESIAN_POINT('',(0.,3.5,-2.02072594216369));
#30234=CARTESIAN_POINT('Origin',(0.,-7.42402667107435E-16,-4.04145188432738));
#30235=CARTESIAN_POINT('',(0.,-7.42402667107435E-16,-4.04145188432738));
#30236=CARTESIAN_POINT('',(0.,-7.42402667107435E-16,-4.04145188432738));
#30237=CARTESIAN_POINT('',(0.,-7.42402667107435E-16,-4.04145188432738));
#30238=CARTESIAN_POINT('Origin',(0.,-3.5,-2.02072594216369));
#30239=CARTESIAN_POINT('',(0.,-3.5,-2.02072594216369));
#30240=CARTESIAN_POINT('',(0.,-3.5,-2.02072594216369));
#30241=CARTESIAN_POINT('',(0.,-3.5,-2.02072594216369));
#30242=CARTESIAN_POINT('Origin',(0.,-3.5,2.02072594216369));
#30243=CARTESIAN_POINT('',(0.,-3.5,2.02072594216369));
#30244=CARTESIAN_POINT('Origin',(2.8,0.,0.));
#30245=CARTESIAN_POINT('Origin',(0.,0.,0.));
#37161=UNCERTAINTY_MEASURE_WITH_UNIT(LENGTH_MEASURE(0.01),#37182,
'DISTANCE_ACCURACY_VALUE',
'Maximum model space distance between geometric entities at asserted c
onnectivities');
#37166=UNCERTAINTY_MEASURE_WITH_UNIT(LENGTH_MEASURE(0.01),#37182,
'DISTANCE_ACCURACY_VALUE',
'Maximum model space distance between geometric entities at asserted c
onnectivities');
#37176=(
GEOMETRIC_REPRESENTATION_CONTEXT(3)
GLOBAL_UNCERTAINTY_ASSIGNED_CONTEXT((#37161))
GLOBAL_UNIT_ASSIGNED_CONTEXT((#37182,#37184,#37185))
REPRESENTATION_CONTEXT('','3D')
);
#37181=(
GEOMETRIC_REPRESENTATION_CONTEXT(3)
GLOBAL_UNCERTAINTY_ASSIGNED_CONTEXT((#37166))
GLOBAL_UNIT_ASSIGNED_CONTEXT((#37182,#37184,#37185))
REPRESENTATION_CONTEXT('','3D')
);
#37182=(
LENGTH_UNIT()
NAMED_UNIT(*)
SI_UNIT(.MILLI.,.METRE.)
);
#37184=(
NAMED_UNIT(*)
PLANE_ANGLE_UNIT()
SI_UNIT($,.RADIAN.)
);
#37185=(
NAMED_UNIT(*)
SI_UNIT($,.STERADIAN.)
SOLID_ANGLE_UNIT()
);
#37195=SHAPE_DEFINITION_REPRESENTATION(#37209,#37246);
#37209=PRODUCT_DEFINITION_SHAPE('',$,#37261);
#37246=SHAPE_REPRESENTATION('',(#15848),#37176);
#37251=PRODUCT_DEFINITION_CONTEXT('part definition',#37295,'design');
#37261=PRODUCT_DEFINITION('2026-10-20-13-23-59-935','09_ISO_4017_M4x16',
#37275,#37251);
#37275=PRODUCT_DEFINITION_FORMATION('',$,#37306);
#37295=APPLICATION_CONTEXT(
'Core Data for Automotive Mechanical Design Process');
#37296=PRODUCT_CONTEXT('part definition',#37295,'mechanical');
#37306=PRODUCT('2026-10-20-13-23-59-935','09_ISO_4017_M4x16',$,(#37296));
#37374=COLOUR_RGB('Black',0.12,0.14,0.17);
#37375=FILL_AREA_STYLE_COLOUR('',#37374);
#37376=FILL_AREA_STYLE('',(#37375));
#37377=SURFACE_STYLE_FILL_AREA(#37376);
#37378=SURFACE_SIDE_STYLE('',(#37377));
#37379=SURFACE_STYLE_USAGE(.BOTH.,#37378);
#37380=PRESENTATION_STYLE_ASSIGNMENT((#37379));
ENDSEC;
END-ISO-10303-21;
